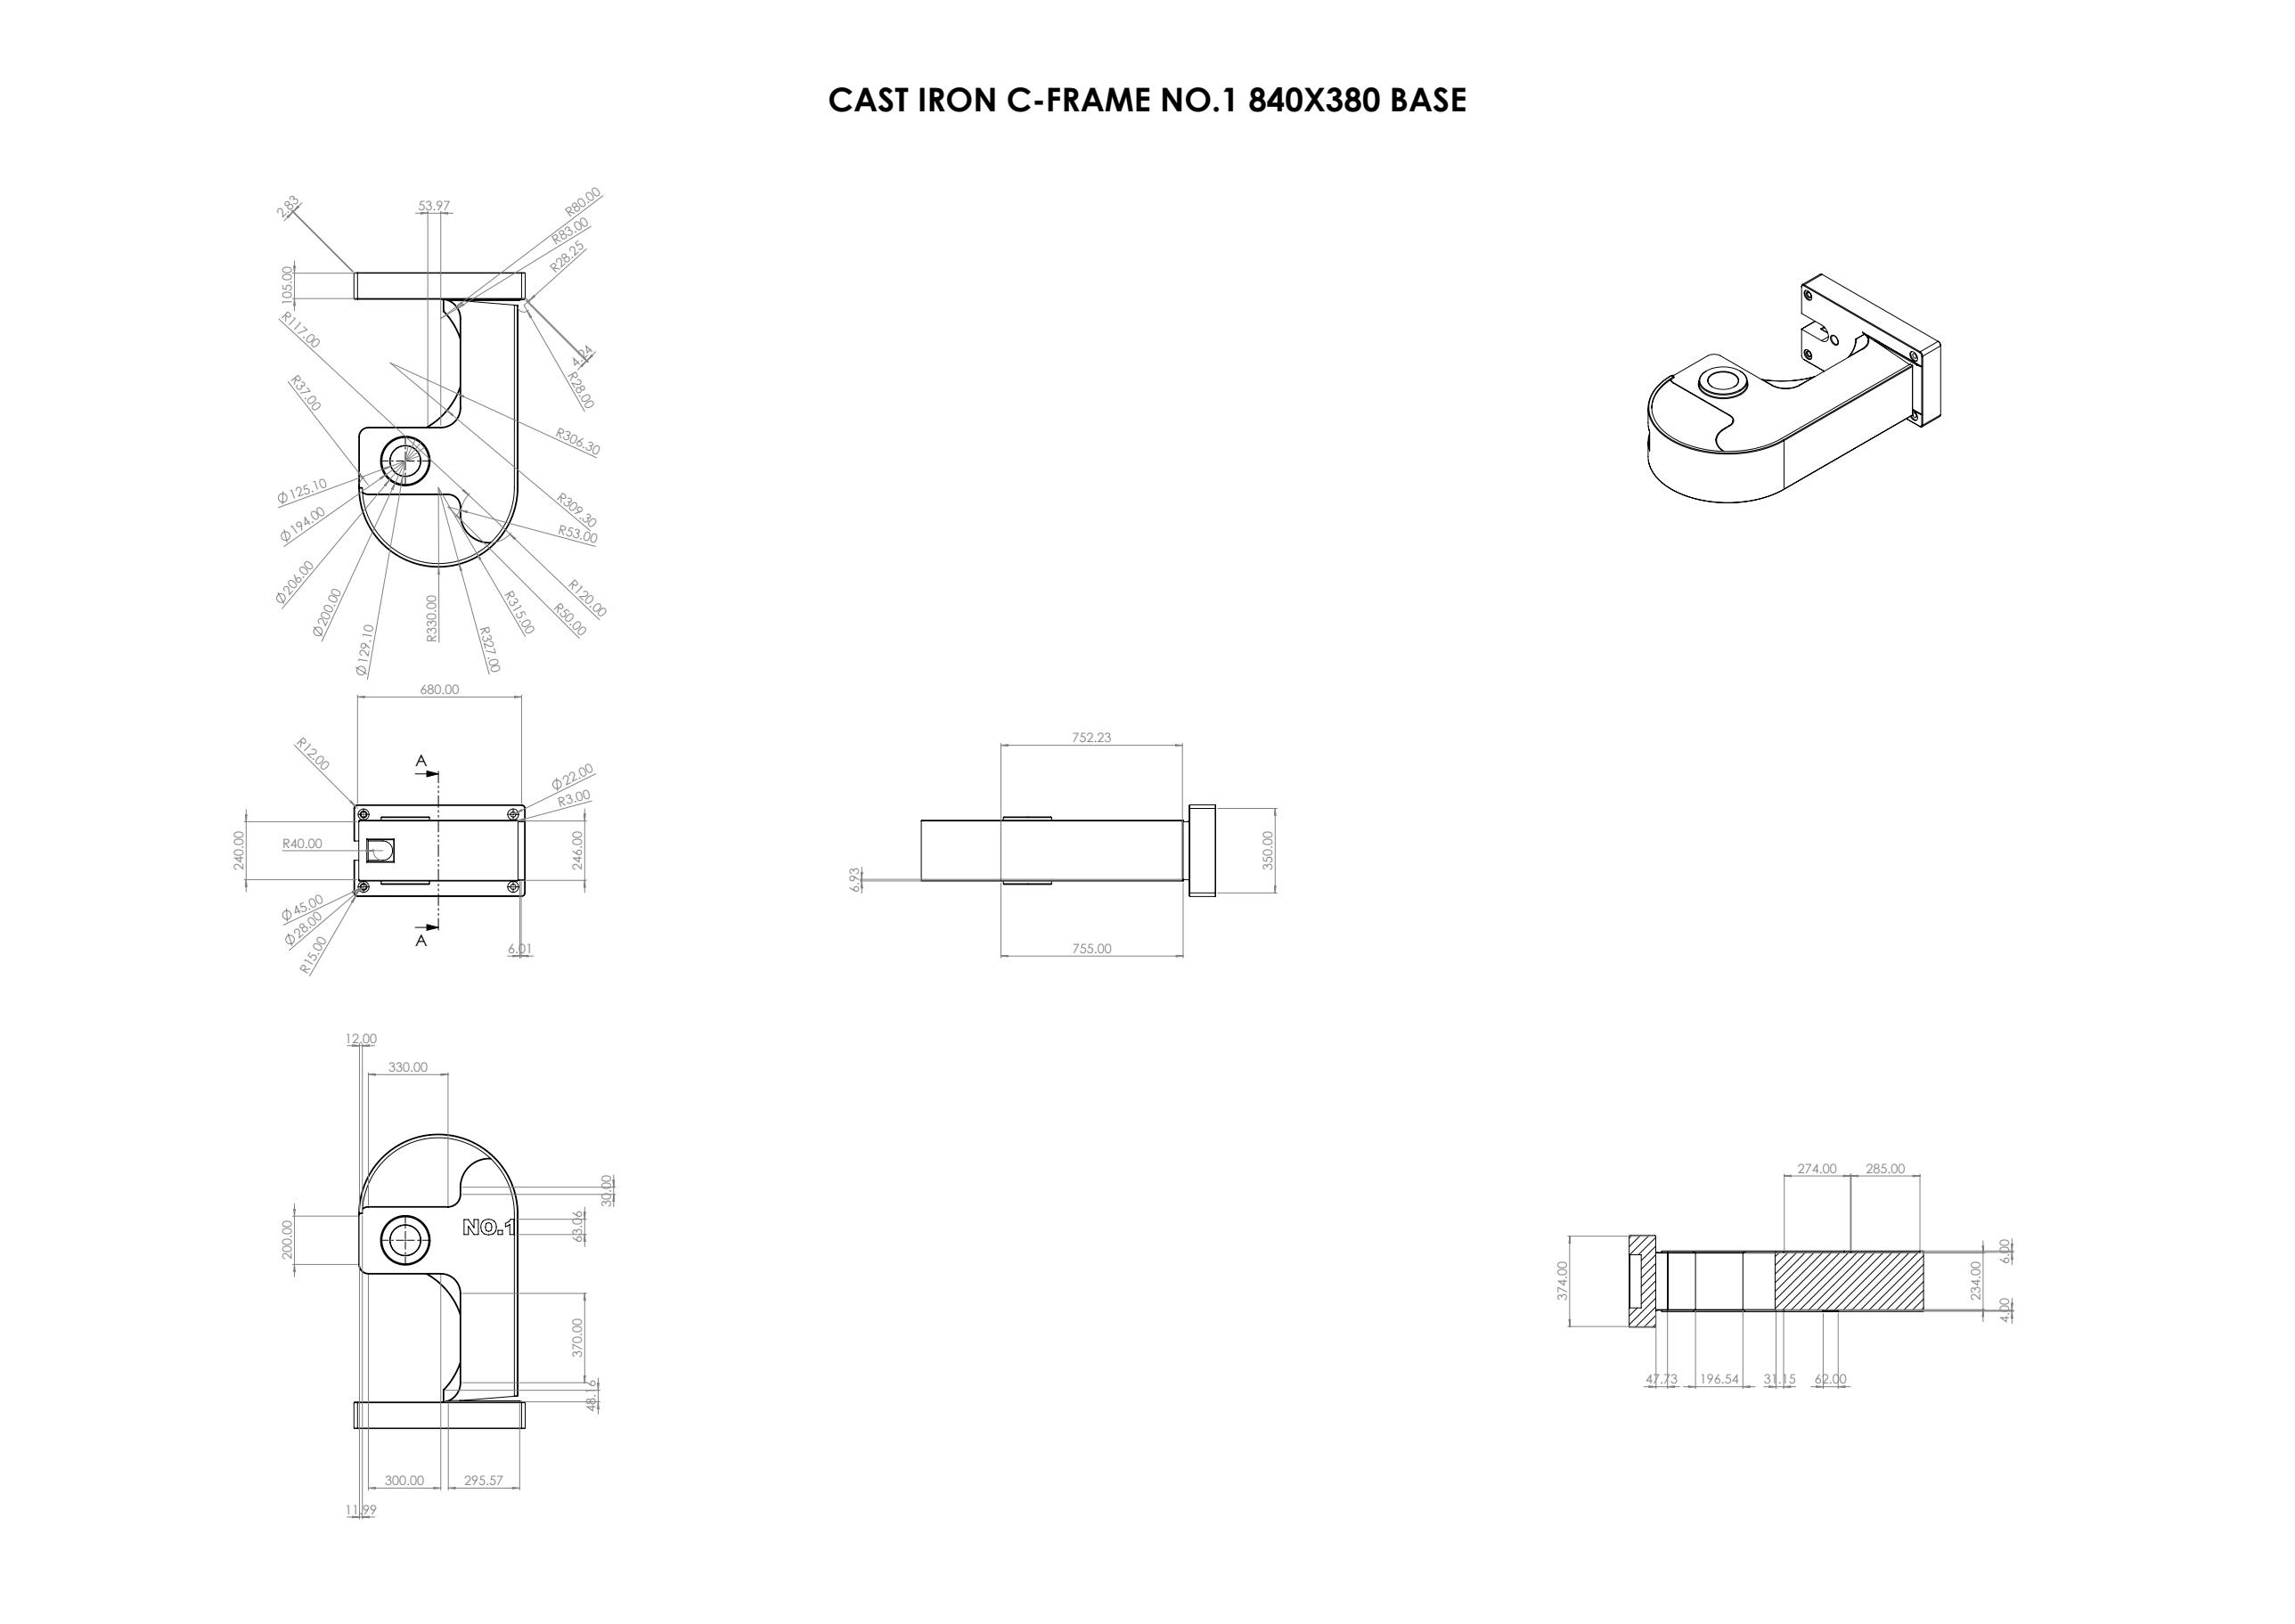
ISO-10303-21;
HEADER;
/* Generated by software containing ST-Developer
 * from STEP Tools, Inc. (www.steptools.com) 
 */

FILE_DESCRIPTION(
/* description */ (''),
/* implementation_level */ '2;1');

FILE_NAME(
/* name */ '01_Cast_Iron_C-Frame_NO.1_840x380_Base.step',
/* time_stamp */ '2026-10-19T23:58:09-07:00',
/* author */ (''),
/* organization */ (''),
/* preprocessor_version */ 'ST-DEVELOPER v20.2',
/* originating_system */ 'Autodesk Translation Framework v15.15.0.0',
/* authorisation */ '');

FILE_SCHEMA (('AP203_CONFIGURATION_CONTROLLED_3D_DESIGN_OF_MECHANICAL_PARTS_AND_ASSEMBLIES_MIM_LF { 1 0 10303 203 3 1 4 }',
'AUTOMOTIVE_DESIGN { 1 0 10303 214 3 1 1 }','INTEGRATED_CNC_SCHEMA','MODEL_BASED_INTEGRATED_MANUFACTURING_SCHEMA',
'PROCESS_PLANNING_SCHEMA','AP242_MANAGED_MODEL_BASED_3D_ENGINEERING_MIM_LF { 1 0 10303 442 3 1 4 }'));
ENDSEC;

DATA;
#10=MECHANICAL_DESIGN_GEOMETRIC_PRESENTATION_REPRESENTATION('',(#420,#421,#422,#423,#424,#425,#426,#427,#428,#429,#430,#431,#432,#433,#434,#435,#436,#437,#438,#439,#440,#441,#442,#443,#444,#445,#446,#447,#448,#449,#450,#451,#452,#453,#454,#455,#456,#457,#458,#459,#460,#461,#462,#463,#464,#465),#70757);
#103=ELLIPSE('',#28418,0.424264068711927,0.3);
#104=ELLIPSE('',#28419,0.42426406871193,0.3);
#105=ELLIPSE('',#28420,0.424264068711931,0.3);
#106=ELLIPSE('',#28425,0.42426406871193,0.3);
#107=ELLIPSE('',#28426,0.424264068711927,0.3);
#108=ELLIPSE('',#28427,0.424264068711928,0.3);
#109=ELLIPSE('',#28431,0.42426406871193,0.3);
#110=ELLIPSE('',#28438,0.424264068711929,0.3);
#111=ELLIPSE('',#28443,0.424264068711926,0.3);
#112=ELLIPSE('',#28444,0.424264068711926,0.3);
#113=ELLIPSE('',#28447,0.424264068711929,0.3);
#114=ELLIPSE('',#28449,0.424264068711931,0.3);
#115=ELLIPSE('',#28458,0.424264068711927,0.3);
#116=ELLIPSE('',#28461,0.42426406871193,0.3);
#117=ELLIPSE('',#28597,5.65698522452918,4.00009261333671);
#118=ELLIPSE('',#28598,5.65698522452918,4.00009261333671);
#119=ELLIPSE('',#28641,0.424264068711926,0.3);
#120=ELLIPSE('',#28642,0.424264068711926,0.3);
#121=ELLIPSE('',#28652,0.424264068711926,0.3);
#122=ELLIPSE('',#28653,0.424264068711926,0.3);
#123=ELLIPSE('',#28709,5.65698522452937,4.00009261333671);
#124=ELLIPSE('',#28711,5.65698522452937,4.00009261333671);
#125=ELLIPSE('',#28723,11.3137084989848,8.);
#126=ELLIPSE('',#28726,11.3137084989848,8.);
#127=ELLIPSE('',#28730,2.63010371137609,2.21164478264163);
#128=ELLIPSE('',#28733,2.63010371137609,2.21164478264163);
#129=ELLIPSE('',#28734,6.83962146739207,5.75141317362232);
#130=ELLIPSE('',#28736,3.53553390593276,2.5);
#131=ELLIPSE('',#28768,11.3130048280025,7.99950242947666);
#132=ELLIPSE('',#28770,11.3130048280025,7.99950242947666);
#133=ELLIPSE('',#28840,6.83962146739207,5.75141317362232);
#134=ELLIPSE('',#28854,3.53553390593276,2.5);
#136=SPHERICAL_SURFACE('',#28433,0.3);
#137=SPHERICAL_SURFACE('',#28439,0.300000000000001);
#138=SPHERICAL_SURFACE('',#28506,0.300000000000004);
#139=SPHERICAL_SURFACE('',#28510,0.299999999999997);
#140=SPHERICAL_SURFACE('',#28532,0.3);
#141=SPHERICAL_SURFACE('',#28555,0.3);
#143=TOROIDAL_SURFACE('',#28397,6.555,0.3);
#144=TOROIDAL_SURFACE('',#28407,6.555,0.3);
#145=TOROIDAL_SURFACE('',#28452,4.3,0.3);
#146=TOROIDAL_SURFACE('',#28476,1.4,0.3);
#147=TOROIDAL_SURFACE('',#28484,1.4,0.3);
#148=TOROIDAL_SURFACE('',#28486,1.4,0.3);
#149=TOROIDAL_SURFACE('',#28494,1.4,0.3);
#150=TOROIDAL_SURFACE('',#28496,1.4,0.3);
#151=TOROIDAL_SURFACE('',#28501,1.4,0.3);
#152=TOROIDAL_SURFACE('',#28516,30.9296013460341,0.3);
#153=TOROIDAL_SURFACE('',#28519,30.9296013460341,0.3);
#154=TOROIDAL_SURFACE('',#28541,32.7,0.3);
#155=TOROIDAL_SURFACE('',#28557,32.7,0.3);
#156=TOROIDAL_SURFACE('',#28568,1.10499999999999,0.3);
#157=TOROIDAL_SURFACE('',#28580,1.10499999999999,0.3);
#158=TOROIDAL_SURFACE('',#28586,1.10499999999999,0.3);
#159=TOROIDAL_SURFACE('',#28592,1.10499999999999,0.3);
#160=TOROIDAL_SURFACE('',#28609,2.3,0.3);
#161=TOROIDAL_SURFACE('',#28615,30.9296013460341,0.3);
#162=TOROIDAL_SURFACE('',#28621,30.9296013460341,0.3);
#163=TOROIDAL_SURFACE('',#28626,2.3,0.3);
#164=TOROIDAL_SURFACE('',#28643,1.10499999999999,0.3);
#165=TOROIDAL_SURFACE('',#28645,1.10499999999999,0.3);
#166=TOROIDAL_SURFACE('',#28647,1.10499999999999,0.3);
#167=TOROIDAL_SURFACE('',#28649,1.10499999999999,0.3);
#168=TOROIDAL_SURFACE('',#28661,32.7,0.3);
#169=TOROIDAL_SURFACE('',#28665,32.7,0.3);
#253=(
BOUNDED_CURVE()
B_SPLINE_CURVE(2,(#64951,#64952,#64953),.UNSPECIFIED.,.F.,.F.)
B_SPLINE_CURVE_WITH_KNOTS((3,3),(0.394392820917162,0.426830556686088),
 .UNSPECIFIED.)
CURVE()
GEOMETRIC_REPRESENTATION_ITEM()
RATIONAL_B_SPLINE_CURVE((1.00046081345666,1.00036632900905,1.00025318515883))
REPRESENTATION_ITEM('')
);
#254=(
BOUNDED_CURVE()
B_SPLINE_CURVE(2,(#64957,#64958,#64959),.UNSPECIFIED.,.F.,.F.)
B_SPLINE_CURVE_WITH_KNOTS((3,3),(0.0334492257654482,0.0658869615343763),
 .UNSPECIFIED.)
CURVE()
GEOMETRIC_REPRESENTATION_ITEM()
RATIONAL_B_SPLINE_CURVE((1.00025318515883,1.00036632900905,1.00046081345666))
REPRESENTATION_ITEM('')
);
#255=(
BOUNDED_CURVE()
B_SPLINE_CURVE(2,(#64996,#64997,#64998),.UNSPECIFIED.,.F.,.F.)
B_SPLINE_CURVE_WITH_KNOTS((3,3),(0.,0.193661196741385),.UNSPECIFIED.)
CURVE()
GEOMETRIC_REPRESENTATION_ITEM()
RATIONAL_B_SPLINE_CURVE((1.,1.00036563245858,1.00040353743124))
REPRESENTATION_ITEM('')
);
#256=(
BOUNDED_CURVE()
B_SPLINE_CURVE(2,(#65154,#65155,#65156),.UNSPECIFIED.,.F.,.F.)
B_SPLINE_CURVE_WITH_KNOTS((3,3),(0.238458916052879,0.432120112749345),
 .UNSPECIFIED.)
CURVE()
GEOMETRIC_REPRESENTATION_ITEM()
RATIONAL_B_SPLINE_CURVE((1.00040353742038,1.0003656324504,1.))
REPRESENTATION_ITEM('')
);
#257=(
BOUNDED_CURVE()
B_SPLINE_CURVE(2,(#65254,#65255,#65256),.UNSPECIFIED.,.F.,.F.)
B_SPLINE_CURVE_WITH_KNOTS((3,3),(0.486252464127642,0.752075607120858),
 .UNSPECIFIED.)
CURVE()
GEOMETRIC_REPRESENTATION_ITEM()
RATIONAL_B_SPLINE_CURVE((1.,1.,1.))
REPRESENTATION_ITEM('')
);
#258=(
BOUNDED_CURVE()
B_SPLINE_CURVE(2,(#65267,#65268,#65269),.UNSPECIFIED.,.F.,.F.)
B_SPLINE_CURVE_WITH_KNOTS((3,3),(0.121648463702186,0.387471606699022),
 .UNSPECIFIED.)
CURVE()
GEOMETRIC_REPRESENTATION_ITEM()
RATIONAL_B_SPLINE_CURVE((1.,1.,1.))
REPRESENTATION_ITEM('')
);
#259=(
BOUNDED_CURVE()
B_SPLINE_CURVE(2,(#65453,#65454,#65455),.UNSPECIFIED.,.F.,.F.)
B_SPLINE_CURVE_WITH_KNOTS((3,3),(0.000218747198876324,0.428298822677418),
 .UNSPECIFIED.)
CURVE()
GEOMETRIC_REPRESENTATION_ITEM()
RATIONAL_B_SPLINE_CURVE((1.,1.,1.))
REPRESENTATION_ITEM('')
);
#260=(
BOUNDED_CURVE()
B_SPLINE_CURVE(2,(#65456,#65457,#65458),.UNSPECIFIED.,.F.,.F.)
B_SPLINE_CURVE_WITH_KNOTS((3,3),(0.432240466163625,0.733007100595233),
 .UNSPECIFIED.)
CURVE()
GEOMETRIC_REPRESENTATION_ITEM()
RATIONAL_B_SPLINE_CURVE((1.,1.,1.))
REPRESENTATION_ITEM('')
);
#261=(
BOUNDED_CURVE()
B_SPLINE_CURVE(2,(#65913,#65914,#65915),.UNSPECIFIED.,.F.,.F.)
B_SPLINE_CURVE_WITH_KNOTS((3,3),(0.,0.428080075478541),.UNSPECIFIED.)
CURVE()
GEOMETRIC_REPRESENTATION_ITEM()
RATIONAL_B_SPLINE_CURVE((1.,1.,1.))
REPRESENTATION_ITEM('')
);
#262=(
BOUNDED_CURVE()
B_SPLINE_CURVE(2,(#65916,#65917,#65918),.UNSPECIFIED.,.F.,.F.)
B_SPLINE_CURVE_WITH_KNOTS((3,3),(0.12344249829562,0.424209132727228),
 .UNSPECIFIED.)
CURVE()
GEOMETRIC_REPRESENTATION_ITEM()
RATIONAL_B_SPLINE_CURVE((1.,1.,1.))
REPRESENTATION_ITEM('')
);
#287=B_SPLINE_SURFACE_WITH_KNOTS('',2,1,((#65478,#65479),(#65480,#65481),
(#65482,#65483)),.UNSPECIFIED.,.F.,.F.,.F.,(3,3),(2,2),(-1.,0.),(0.,0.4),
 .UNSPECIFIED.);
#288=B_SPLINE_SURFACE_WITH_KNOTS('',2,1,((#65489,#65490),(#65491,#65492),
(#65493,#65494)),.UNSPECIFIED.,.F.,.F.,.F.,(3,3),(2,2),(-1.,0.),(0.,0.4),
 .UNSPECIFIED.);
#289=B_SPLINE_SURFACE_WITH_KNOTS('',2,1,((#65504,#65505),(#65506,#65507),
(#65508,#65509)),.UNSPECIFIED.,.F.,.F.,.F.,(3,3),(2,2),(-1.,0.),(0.,0.4),
 .UNSPECIFIED.);
#290=B_SPLINE_SURFACE_WITH_KNOTS('',2,1,((#65515,#65516),(#65517,#65518),
(#65519,#65520)),.UNSPECIFIED.,.F.,.F.,.F.,(3,3),(2,2),(-1.,0.),(0.,0.4),
 .UNSPECIFIED.);
#291=B_SPLINE_SURFACE_WITH_KNOTS('',2,1,((#65570,#65571),(#65572,#65573),
(#65574,#65575)),.UNSPECIFIED.,.F.,.F.,.F.,(3,3),(2,2),(-1.,0.),(0.,0.4),
 .UNSPECIFIED.);
#292=B_SPLINE_SURFACE_WITH_KNOTS('',2,1,((#65588,#65589),(#65590,#65591),
(#65592,#65593)),.UNSPECIFIED.,.F.,.F.,.F.,(3,3),(2,2),(-1.,0.),(0.,0.4),
 .UNSPECIFIED.);
#293=B_SPLINE_SURFACE_WITH_KNOTS('',2,1,((#65603,#65604),(#65605,#65606),
(#65607,#65608)),.UNSPECIFIED.,.F.,.F.,.F.,(3,3),(2,2),(-1.,0.),(0.,0.4),
 .UNSPECIFIED.);
#294=B_SPLINE_SURFACE_WITH_KNOTS('',2,1,((#65618,#65619),(#65620,#65621),
(#65622,#65623)),.UNSPECIFIED.,.F.,.F.,.F.,(3,3),(2,2),(-1.,0.),(0.,0.4),
 .UNSPECIFIED.);
#295=B_SPLINE_SURFACE_WITH_KNOTS('',2,1,((#65633,#65634),(#65635,#65636),
(#65637,#65638)),.UNSPECIFIED.,.F.,.F.,.F.,(3,3),(2,2),(-1.,0.),(0.,0.4),
 .UNSPECIFIED.);
#296=B_SPLINE_SURFACE_WITH_KNOTS('',2,1,((#65648,#65649),(#65650,#65651),
(#65652,#65653)),.UNSPECIFIED.,.F.,.F.,.F.,(3,3),(2,2),(-1.,0.),(0.,0.4),
 .UNSPECIFIED.);
#297=B_SPLINE_SURFACE_WITH_KNOTS('',2,1,((#65663,#65664),(#65665,#65666),
(#65667,#65668)),.UNSPECIFIED.,.F.,.F.,.F.,(3,3),(2,2),(-1.,0.),(0.,0.4),
 .UNSPECIFIED.);
#298=B_SPLINE_SURFACE_WITH_KNOTS('',2,1,((#65678,#65679),(#65680,#65681),
(#65682,#65683)),.UNSPECIFIED.,.F.,.F.,.F.,(3,3),(2,2),(-1.,0.),(0.,0.4),
 .UNSPECIFIED.);
#299=B_SPLINE_SURFACE_WITH_KNOTS('',2,1,((#65690,#65691),(#65692,#65693),
(#65694,#65695)),.UNSPECIFIED.,.F.,.F.,.F.,(3,3),(2,2),(-1.,0.),(0.,0.4),
 .UNSPECIFIED.);
#300=B_SPLINE_SURFACE_WITH_KNOTS('',2,1,((#65703,#65704),(#65705,#65706),
(#65707,#65708)),.UNSPECIFIED.,.F.,.F.,.F.,(3,3),(2,2),(-1.,0.),(0.,0.4),
 .UNSPECIFIED.);
#301=B_SPLINE_SURFACE_WITH_KNOTS('',2,1,((#65714,#65715),(#65716,#65717),
(#65718,#65719)),.UNSPECIFIED.,.F.,.F.,.F.,(3,3),(2,2),(-1.,0.),(0.,0.4),
 .UNSPECIFIED.);
#302=B_SPLINE_SURFACE_WITH_KNOTS('',2,1,((#65725,#65726),(#65727,#65728),
(#65729,#65730)),.UNSPECIFIED.,.F.,.F.,.F.,(3,3),(2,2),(-1.,0.),(0.,0.4),
 .UNSPECIFIED.);
#303=B_SPLINE_SURFACE_WITH_KNOTS('',2,1,((#65736,#65737),(#65738,#65739),
(#65740,#65741)),.UNSPECIFIED.,.F.,.F.,.F.,(3,3),(2,2),(-1.,0.),(0.,0.4),
 .UNSPECIFIED.);
#304=B_SPLINE_SURFACE_WITH_KNOTS('',2,1,((#65747,#65748),(#65749,#65750),
(#65751,#65752)),.UNSPECIFIED.,.F.,.F.,.F.,(3,3),(2,2),(-1.,0.),(0.,0.4),
 .UNSPECIFIED.);
#305=B_SPLINE_SURFACE_WITH_KNOTS('',2,1,((#65758,#65759),(#65760,#65761),
(#65762,#65763)),.UNSPECIFIED.,.F.,.F.,.F.,(3,3),(2,2),(-1.,0.),(0.,0.4),
 .UNSPECIFIED.);
#306=B_SPLINE_SURFACE_WITH_KNOTS('',2,1,((#65769,#65770),(#65771,#65772),
(#65773,#65774)),.UNSPECIFIED.,.F.,.F.,.F.,(3,3),(2,2),(-1.,0.),(0.,0.4),
 .UNSPECIFIED.);
#307=B_SPLINE_SURFACE_WITH_KNOTS('',2,1,((#65780,#65781),(#65782,#65783),
(#65784,#65785)),.UNSPECIFIED.,.F.,.F.,.F.,(3,3),(2,2),(-1.,0.),(0.,0.4),
 .UNSPECIFIED.);
#308=B_SPLINE_SURFACE_WITH_KNOTS('',2,1,((#65791,#65792),(#65793,#65794),
(#65795,#65796)),.UNSPECIFIED.,.F.,.F.,.F.,(3,3),(2,2),(-1.,0.),(0.,0.4),
 .UNSPECIFIED.);
#390=SHAPE_REPRESENTATION_RELATIONSHIP('SRR','None',#70831,#405);
#405=ADVANCED_BREP_SHAPE_REPRESENTATION('',(#480),#70755);
#420=STYLED_ITEM('',(#71026),#26633);
#421=STYLED_ITEM('',(#71026),#26634);
#422=STYLED_ITEM('',(#71026),#26635);
#423=STYLED_ITEM('',(#71026),#26636);
#424=STYLED_ITEM('',(#71026),#26637);
#425=STYLED_ITEM('',(#71026),#26638);
#426=STYLED_ITEM('',(#71026),#26639);
#427=STYLED_ITEM('',(#71026),#26640);
#428=STYLED_ITEM('',(#71026),#26641);
#429=STYLED_ITEM('',(#71026),#26642);
#430=STYLED_ITEM('',(#71026),#26643);
#431=STYLED_ITEM('',(#71026),#26644);
#432=STYLED_ITEM('',(#71026),#26645);
#433=STYLED_ITEM('',(#71026),#26646);
#434=STYLED_ITEM('',(#71026),#26647);
#435=STYLED_ITEM('',(#71026),#26648);
#436=STYLED_ITEM('',(#71026),#26649);
#437=STYLED_ITEM('',(#71026),#26650);
#438=STYLED_ITEM('',(#71026),#26651);
#439=STYLED_ITEM('',(#71026),#26652);
#440=STYLED_ITEM('',(#71026),#26653);
#441=STYLED_ITEM('',(#71026),#26654);
#442=STYLED_ITEM('',(#71026),#26655);
#443=STYLED_ITEM('',(#71026),#26656);
#444=STYLED_ITEM('',(#71026),#26657);
#445=STYLED_ITEM('',(#71026),#26658);
#446=STYLED_ITEM('',(#71026),#26659);
#447=STYLED_ITEM('',(#71026),#26660);
#448=STYLED_ITEM('',(#71026),#26661);
#449=STYLED_ITEM('',(#71026),#26662);
#450=STYLED_ITEM('',(#71026),#26663);
#451=STYLED_ITEM('',(#71026),#26664);
#452=STYLED_ITEM('',(#71026),#26665);
#453=STYLED_ITEM('',(#71026),#26666);
#454=STYLED_ITEM('',(#71026),#26667);
#455=STYLED_ITEM('',(#71026),#26668);
#456=STYLED_ITEM('',(#71026),#26669);
#457=STYLED_ITEM('',(#71026),#26670);
#458=STYLED_ITEM('',(#71026),#26671);
#459=STYLED_ITEM('',(#71026),#26672);
#460=STYLED_ITEM('',(#71026),#26673);
#461=STYLED_ITEM('',(#71026),#26674);
#462=STYLED_ITEM('',(#71026),#26675);
#463=STYLED_ITEM('',(#71026),#26676);
#464=STYLED_ITEM('',(#71026),#26677);
#465=STYLED_ITEM('',(#71026),#480);
#480=MANIFOLD_SOLID_BREP('Frame',#26885);
#741=CYLINDRICAL_SURFACE('',#28401,0.3);
#742=CYLINDRICAL_SURFACE('',#28404,0.3);
#743=CYLINDRICAL_SURFACE('',#28414,6.255);
#744=CYLINDRICAL_SURFACE('',#28417,0.3);
#745=CYLINDRICAL_SURFACE('',#28424,0.3);
#746=CYLINDRICAL_SURFACE('',#28430,0.3);
#747=CYLINDRICAL_SURFACE('',#28437,0.3);
#748=CYLINDRICAL_SURFACE('',#28442,0.3);
#749=CYLINDRICAL_SURFACE('',#28445,0.3);
#750=CYLINDRICAL_SURFACE('',#28446,0.3);
#751=CYLINDRICAL_SURFACE('',#28448,0.3);
#752=CYLINDRICAL_SURFACE('',#28450,0.3);
#753=CYLINDRICAL_SURFACE('',#28456,0.3);
#754=CYLINDRICAL_SURFACE('',#28457,0.3);
#755=CYLINDRICAL_SURFACE('',#28459,0.3);
#756=CYLINDRICAL_SURFACE('',#28460,0.3);
#757=CYLINDRICAL_SURFACE('',#28480,1.1);
#758=CYLINDRICAL_SURFACE('',#28490,1.1);
#759=CYLINDRICAL_SURFACE('',#28499,1.1);
#760=CYLINDRICAL_SURFACE('',#28504,1.1);
#761=CYLINDRICAL_SURFACE('',#28514,0.3);
#762=CYLINDRICAL_SURFACE('',#28515,0.3);
#763=CYLINDRICAL_SURFACE('',#28522,0.3);
#764=CYLINDRICAL_SURFACE('',#28527,0.3);
#765=CYLINDRICAL_SURFACE('',#28529,0.3);
#766=CYLINDRICAL_SURFACE('',#28534,31.5);
#767=CYLINDRICAL_SURFACE('',#28544,33.);
#768=CYLINDRICAL_SURFACE('',#28550,0.3);
#769=CYLINDRICAL_SURFACE('',#28553,0.3);
#770=CYLINDRICAL_SURFACE('',#28562,31.5);
#771=CYLINDRICAL_SURFACE('',#28566,0.3);
#772=CYLINDRICAL_SURFACE('',#28578,0.804999999999993);
#773=CYLINDRICAL_SURFACE('',#28584,0.804999999999993);
#774=CYLINDRICAL_SURFACE('',#28590,0.804999999999993);
#775=CYLINDRICAL_SURFACE('',#28596,4.00009261333671);
#776=CYLINDRICAL_SURFACE('',#28599,0.804999999999993);
#777=CYLINDRICAL_SURFACE('',#28601,0.3);
#778=CYLINDRICAL_SURFACE('',#28612,2.);
#779=CYLINDRICAL_SURFACE('',#28618,30.6296013460341);
#780=CYLINDRICAL_SURFACE('',#28639,0.3);
#781=CYLINDRICAL_SURFACE('',#28651,0.3);
#782=CYLINDRICAL_SURFACE('',#28654,0.3);
#783=CYLINDRICAL_SURFACE('',#28669,0.3);
#784=CYLINDRICAL_SURFACE('',#28686,4.00009261333671);
#785=CYLINDRICAL_SURFACE('',#28691,12.);
#786=CYLINDRICAL_SURFACE('',#28705,4.00009261333671);
#787=CYLINDRICAL_SURFACE('',#28708,4.00009261333671);
#788=CYLINDRICAL_SURFACE('',#28710,4.00009261333671);
#789=CYLINDRICAL_SURFACE('',#28722,8.);
#790=CYLINDRICAL_SURFACE('',#28724,8.);
#791=CYLINDRICAL_SURFACE('',#28735,2.5);
#792=CYLINDRICAL_SURFACE('',#28740,7.99950242947665);
#793=CYLINDRICAL_SURFACE('',#28741,7.99950242947665);
#794=CYLINDRICAL_SURFACE('',#28746,12.);
#795=CYLINDRICAL_SURFACE('',#28754,4.00009261333671);
#796=CYLINDRICAL_SURFACE('',#28758,4.00009261333671);
#797=CYLINDRICAL_SURFACE('',#28760,5.00011576667089);
#798=CYLINDRICAL_SURFACE('',#28767,7.99950242947666);
#799=CYLINDRICAL_SURFACE('',#28769,7.99950242947666);
#800=CYLINDRICAL_SURFACE('',#28772,30.6296013460341);
#801=CYLINDRICAL_SURFACE('',#28802,2.25);
#802=CYLINDRICAL_SURFACE('',#28805,2.25);
#803=CYLINDRICAL_SURFACE('',#28806,2.25);
#804=CYLINDRICAL_SURFACE('',#28807,2.25);
#805=CYLINDRICAL_SURFACE('',#28811,4.);
#806=CYLINDRICAL_SURFACE('',#28830,10.);
#807=CYLINDRICAL_SURFACE('',#28836,10.);
#808=CYLINDRICAL_SURFACE('',#28851,5.);
#809=CYLINDRICAL_SURFACE('',#28853,2.5);
#810=CYLINDRICAL_SURFACE('',#28873,1.5);
#811=CYLINDRICAL_SURFACE('',#28876,1.5);
#812=CYLINDRICAL_SURFACE('',#28889,1.5);
#813=CYLINDRICAL_SURFACE('',#28890,1.5);
#887=FACE_BOUND('',#5214,.T.);
#888=FACE_BOUND('',#5215,.T.);
#889=FACE_BOUND('',#5216,.T.);
#890=FACE_BOUND('',#5217,.T.);
#891=FACE_BOUND('',#5219,.T.);
#892=FACE_BOUND('',#5225,.T.);
#893=FACE_BOUND('',#5230,.T.);
#894=FACE_BOUND('',#5252,.T.);
#895=FACE_BOUND('',#5263,.T.);
#896=FACE_BOUND('',#5264,.T.);
#897=FACE_BOUND('',#5265,.T.);
#898=FACE_BOUND('',#5276,.T.);
#899=FACE_BOUND('',#5277,.T.);
#900=FACE_BOUND('',#5278,.T.);
#901=FACE_BOUND('',#5279,.T.);
#902=FACE_BOUND('',#5290,.T.);
#903=FACE_BOUND('',#5291,.T.);
#904=FACE_BOUND('',#5292,.T.);
#905=FACE_BOUND('',#5293,.T.);
#906=FACE_BOUND('',#5294,.T.);
#907=FACE_BOUND('',#5295,.T.);
#908=FACE_BOUND('',#5318,.T.);
#909=FACE_BOUND('',#5319,.T.);
#910=FACE_BOUND('',#5320,.T.);
#911=FACE_BOUND('',#5321,.T.);
#912=FACE_BOUND('',#5322,.T.);
#913=FACE_BOUND('',#5330,.T.);
#914=FACE_BOUND('',#5418,.T.);
#915=FACE_BOUND('',#5425,.T.);
#916=FACE_BOUND('',#5428,.T.);
#917=FACE_BOUND('',#5446,.T.);
#918=FACE_BOUND('',#5449,.T.);
#1398=B_SPLINE_CURVE_WITH_KNOTS('',3,(#63938,#63939,#63940,#63941,#63942,
#63943,#63944,#63945,#63946,#63947,#63948,#63949),.UNSPECIFIED.,.F.,.F.,
(4,2,2,2,2,4),(-1.10588413989679,-1.10499782596143,-0.91656040147052,-0.772228700060969,
-0.6650055247649,-0.579920166124102),.UNSPECIFIED.);
#1399=B_SPLINE_CURVE_WITH_KNOTS('',3,(#63952,#63953,#63954,#63955,#63956,
#63957,#63958,#63959,#63960,#63961,#63962,#63963,#63964,#63965),
 .UNSPECIFIED.,.F.,.F.,(4,2,2,2,2,2,4),(-0.568877288175113,-0.484148554868537,
-0.388033769227592,-0.2597032346067,-0.133006563450214,0.,0.00108165162707012),
 .UNSPECIFIED.);
#1400=B_SPLINE_CURVE_WITH_KNOTS('',3,(#63974,#63975,#63976,#63977,#63978,
#63979,#63980,#63981,#63982,#63983,#63984,#63985),.UNSPECIFIED.,.F.,.F.,
(4,2,2,2,2,4),(-0.00108165162924514,0.,0.229967778999105,0.40610922702663,
0.536963676703178,0.64080128223702),.UNSPECIFIED.);
#1401=B_SPLINE_CURVE_WITH_KNOTS('',3,(#63996,#63997,#63998,#63999,#64000,
#64001,#64002,#64003,#64004,#64005,#64006,#64007,#64008,#64009),
 .UNSPECIFIED.,.F.,.F.,(4,2,2,2,2,2,4),(0.,0.0839640955338038,0.179211489526657,
0.306383900210746,0.431937192294976,0.563743432804494,0.564815323027158),
 .UNSPECIFIED.);
#1402=B_SPLINE_CURVE_WITH_KNOTS('',3,(#64272,#64273,#64274,#64275,#64276,
#64277,#64278,#64279,#64280,#64281),.UNSPECIFIED.,.F.,.F.,(4,2,2,2,4),(-0.454509794253164,
-0.340166127818439,-0.225822461383713,-0.112911230691856,0.),
 .UNSPECIFIED.);
#1403=B_SPLINE_CURVE_WITH_KNOTS('',3,(#64287,#64288,#64289,#64290,#64291,
#64292,#64293,#64294,#64295,#64296,#64297,#64298,#64299,#64300),
 .UNSPECIFIED.,.F.,.F.,(4,2,2,2,2,2,4),(0.896032537461048,1.25582804826943,
1.43572580367362,1.61562355907781,1.76667897073219,1.80865046008187,1.84248908085934),
 .UNSPECIFIED.);
#1404=B_SPLINE_CURVE_WITH_KNOTS('',3,(#64306,#64307,#64308,#64309,#64310,
#64311,#64312,#64313,#64314,#64315,#64316,#64317,#64318,#64319),
 .UNSPECIFIED.,.F.,.F.,(4,2,2,2,2,2,4),(-1.84248908085934,-1.80865046008187,
-1.76667897073219,-1.61562355907781,-1.43572580367362,-1.25582804826943,
-0.896032537461048),.UNSPECIFIED.);
#1405=B_SPLINE_CURVE_WITH_KNOTS('',3,(#64325,#64326,#64327,#64328,#64329,
#64330,#64331,#64332,#64333,#64334),.UNSPECIFIED.,.F.,.F.,(4,2,2,2,4),(0.910251315816355,
1.02316254650821,1.13607377720007,1.25041744363479,1.36476111006952),
 .UNSPECIFIED.);
#1406=B_SPLINE_CURVE_WITH_KNOTS('',3,(#64358,#64359,#64360,#64361,#64362,
#64363,#64364,#64365,#64366,#64367),.UNSPECIFIED.,.F.,.F.,(4,2,2,2,4),(0.45204596998448,
0.565054126336166,0.678062282687852,0.791068360433516,0.904074438179181),
 .UNSPECIFIED.);
#1407=B_SPLINE_CURVE_WITH_KNOTS('',3,(#64376,#64377,#64378,#64379,#64380,
#64381),.UNSPECIFIED.,.F.,.F.,(4,2,4),(1.02915974263557,1.15320944997464,
1.25900965381776),.UNSPECIFIED.);
#1408=B_SPLINE_CURVE_WITH_KNOTS('',3,(#64400,#64401,#64402,#64403,#64404,
#64405),.UNSPECIFIED.,.F.,.F.,(4,2,4),(1.70043874542,2.00091514457436,2.20444648124611),
 .UNSPECIFIED.);
#1409=B_SPLINE_CURVE_WITH_KNOTS('',3,(#64413,#64414,#64415,#64416,#64417,
#64418),.UNSPECIFIED.,.F.,.F.,(4,2,4),(1.92266359511738,1.95634912709283,
2.38915999737552),.UNSPECIFIED.);
#1410=B_SPLINE_CURVE_WITH_KNOTS('',3,(#64457,#64458,#64459,#64460,#64461,
#64462),.UNSPECIFIED.,.F.,.F.,(4,2,4),(0.941765464328093,1.04756566817122,
1.17161537551029),.UNSPECIFIED.);
#1411=B_SPLINE_CURVE_WITH_KNOTS('',3,(#64472,#64473,#64474,#64475,#64476,
#64477,#64478,#64479,#64480,#64481),.UNSPECIFIED.,.F.,.F.,(4,2,2,2,4),(1.80814887635836,
1.92115495410403,2.03416103184969,2.14716918820138,2.26017734455306),
 .UNSPECIFIED.);
#1412=B_SPLINE_CURVE_WITH_KNOTS('',3,(#64506,#64507,#64508,#64509,#64510,
#64511),.UNSPECIFIED.,.F.,.F.,(4,2,4),(1.52353825936373,1.95634912840093,
1.99003466162308),.UNSPECIFIED.);
#1413=B_SPLINE_CURVE_WITH_KNOTS('',3,(#64519,#64520,#64521,#64522,#64523,
#64524),.UNSPECIFIED.,.F.,.F.,(4,2,4),(1.79738380790266,2.00091514457441,
2.30139154372878),.UNSPECIFIED.);
#1414=B_SPLINE_CURVE_WITH_KNOTS('',3,(#64530,#64531,#64532,#64533,#64534,
#64535,#64536,#64537,#64538,#64539),.UNSPECIFIED.,.F.,.F.,(4,2,2,2,4),(-0.385669957148059,
-0.267638091880424,-0.132795783635376,0.,0.000970573886634806),
 .UNSPECIFIED.);
#1415=B_SPLINE_CURVE_WITH_KNOTS('',3,(#64542,#64543,#64544,#64545,#64546,
#64547,#64548,#64549,#64550,#64551),.UNSPECIFIED.,.F.,.F.,(4,2,2,2,4),(-0.384357938358326,
-0.383393117455112,-0.251376894581821,-0.117331137795169,-6.31601177111807E-6),
 .UNSPECIFIED.);
#1416=B_SPLINE_CURVE_WITH_KNOTS('',3,(#64554,#64555,#64556,#64557,#64558,
#64559),.UNSPECIFIED.,.F.,.F.,(4,2,4),(0.29237536973302,0.349212088502275,
0.491998450222318),.UNSPECIFIED.);
#1417=B_SPLINE_CURVE_WITH_KNOTS('',3,(#64566,#64567,#64568,#64569,#64570,
#64571),.UNSPECIFIED.,.F.,.F.,(4,2,4),(1.47810928760726,1.6208956493273,
1.67773236809654),.UNSPECIFIED.);
#1418=B_SPLINE_CURVE_WITH_KNOTS('',3,(#64629,#64630,#64631,#64632,#64633,
#64634,#64635,#64636,#64637,#64638),.UNSPECIFIED.,.F.,.F.,(4,2,2,2,4),(-0.00645513076503384,
0.,0.607350167241916,1.21470033231699,1.22115546305417),.UNSPECIFIED.);
#1419=B_SPLINE_CURVE_WITH_KNOTS('',3,(#64646,#64647,#64648,#64649,#64650,
#64651,#64652,#64653,#64654,#64655,#64656,#64657,#64658,#64659,#64660,#64661,
#64662,#64663),.UNSPECIFIED.,.F.,.F.,(4,2,2,2,2,2,2,2,4),(0.,0.753367592696705,
1.50673518539341,2.26010277809012,3.01347037078682,3.76683796348352,4.52020555618022,
5.27357314887692,6.02694074157362),.UNSPECIFIED.);
#1420=B_SPLINE_CURVE_WITH_KNOTS('',3,(#64674,#64675,#64676,#64677,#64678,
#64679,#64680,#64681,#64682,#64683,#64684,#64685,#64686,#64687,#64688,#64689,
#64690,#64691),.UNSPECIFIED.,.F.,.F.,(4,2,2,2,2,2,2,2,4),(-6.02694148316008,
-5.27373586786722,-4.52034502960047,-3.76695419133371,-3.01356335306695,
-2.26017251480021,-1.50678167653347,-0.753390838266739,0.),
 .UNSPECIFIED.);
#1421=B_SPLINE_CURVE_WITH_KNOTS('',3,(#64698,#64699,#64700,#64701,#64702,
#64703,#64704,#64705,#64706,#64707,#64708,#64709,#64710,#64711),
 .UNSPECIFIED.,.F.,.F.,(4,2,2,2,2,2,4),(-1.35055637186862,-1.34938170454602,
-1.1819777528807,-1.01919166368985,-0.865721094274056,-0.748962828335224,
-0.646651719983809),.UNSPECIFIED.);
#1422=B_SPLINE_CURVE_WITH_KNOTS('',3,(#64713,#64714,#64715,#64716,#64717,
#64718,#64719,#64720,#64721,#64722,#64723,#64724,#64725,#64726),
 .UNSPECIFIED.,.F.,.F.,(4,2,2,2,2,2,4),(-0.575633174348645,-0.491826207716573,
-0.3961850186411,-0.270471368845074,-0.13712701884174,0.,0.000962215215251001),
 .UNSPECIFIED.);
#1423=B_SPLINE_CURVE_WITH_KNOTS('',3,(#64768,#64769,#64770,#64771,#64772,
#64773,#64774,#64775,#64776,#64777,#64778,#64779,#64780,#64781),
 .UNSPECIFIED.,.F.,.F.,(4,2,2,2,2,2,4),(-1.35886617414881,-1.31800777766679,
-1.27191156834586,-1.14095894304151,-0.942079387318738,-0.807488859272477,
-0.672898331226217),.UNSPECIFIED.);
#1424=B_SPLINE_CURVE_WITH_KNOTS('',3,(#64785,#64786,#64787,#64788,#64789,
#64790,#64791,#64792,#64793,#64794,#64795,#64796,#64797,#64798),
 .UNSPECIFIED.,.F.,.F.,(4,2,2,2,2,2,4),(0.896032537461047,1.25582804826943,
1.43572580367362,1.61562355907781,1.76667897073219,1.80865046008187,1.84248908085934),
 .UNSPECIFIED.);
#1425=B_SPLINE_CURVE_WITH_KNOTS('',3,(#64814,#64815,#64816,#64817,#64818,
#64819,#64820,#64821,#64822,#64823,#64824,#64825,#64826,#64827),
 .UNSPECIFIED.,.F.,.F.,(4,2,2,2,2,2,4),(-1.84248908085934,-1.80865046008187,
-1.76667897073219,-1.61562355907781,-1.43572580367362,-1.25582804826943,
-0.896032537461046),.UNSPECIFIED.);
#1426=B_SPLINE_CURVE_WITH_KNOTS('',3,(#64830,#64831,#64832,#64833,#64834,
#64835,#64836,#64837,#64838,#64839,#64840,#64841,#64842,#64843),
 .UNSPECIFIED.,.F.,.F.,(4,2,2,2,2,2,4),(0.672898331226217,0.807488859272477,
0.942079387318738,1.14095894304151,1.27191156834586,1.31800777766679,1.35886617414881),
 .UNSPECIFIED.);
#1427=B_SPLINE_CURVE_WITH_KNOTS('',3,(#64924,#64925,#64926,#64927,#64928,
#64929),.UNSPECIFIED.,.F.,.F.,(4,2,4),(-0.154287651470972,-0.153320461931147,
-0.0301403351196061),.UNSPECIFIED.);
#1428=B_SPLINE_CURVE_WITH_KNOTS('',3,(#64933,#64934,#64935,#64936,#64937,
#64938),.UNSPECIFIED.,.F.,.F.,(4,2,4),(0.0301403351196109,0.153320461931147,
0.154287651470978),.UNSPECIFIED.);
#1429=B_SPLINE_CURVE_WITH_KNOTS('',3,(#65002,#65003,#65004,#65005),
 .UNSPECIFIED.,.F.,.F.,(4,4),(23.0837010026238,23.1300949206487),
 .UNSPECIFIED.);
#1430=B_SPLINE_CURVE_WITH_KNOTS('',3,(#65006,#65007,#65008,#65009,#65010,
#65011),.UNSPECIFIED.,.F.,.F.,(4,2,4),(-0.978411907643555,-0.753390838266736,
0.),.UNSPECIFIED.);
#1431=B_SPLINE_CURVE_WITH_KNOTS('',3,(#65020,#65021,#65022,#65023,#65024,
#65025,#65026,#65027,#65028,#65029),.UNSPECIFIED.,.F.,.F.,(4,2,2,2,4),(-6.02694148316005,
-5.27373586786722,-4.52034502960046,-3.7669541913337,-3.53970622743003),
 .UNSPECIFIED.);
#1432=B_SPLINE_CURVE_WITH_KNOTS('',2,(#65054,#65055,#65056),
 .UNSPECIFIED.,.F.,.F.,(3,3),(0.,1.),.UNSPECIFIED.);
#1433=B_SPLINE_CURVE_WITH_KNOTS('',2,(#65058,#65059,#65060),
 .UNSPECIFIED.,.F.,.F.,(3,3),(0.,1.),.UNSPECIFIED.);
#1434=B_SPLINE_CURVE_WITH_KNOTS('',2,(#65062,#65063,#65064),
 .UNSPECIFIED.,.F.,.F.,(3,3),(0.,1.),.UNSPECIFIED.);
#1435=B_SPLINE_CURVE_WITH_KNOTS('',2,(#65066,#65067,#65068),
 .UNSPECIFIED.,.F.,.F.,(3,3),(0.,1.),.UNSPECIFIED.);
#1436=B_SPLINE_CURVE_WITH_KNOTS('',2,(#65070,#65071,#65072),
 .UNSPECIFIED.,.F.,.F.,(3,3),(0.,1.),.UNSPECIFIED.);
#1437=B_SPLINE_CURVE_WITH_KNOTS('',2,(#65074,#65075,#65076),
 .UNSPECIFIED.,.F.,.F.,(3,3),(0.,1.),.UNSPECIFIED.);
#1438=B_SPLINE_CURVE_WITH_KNOTS('',2,(#65078,#65079,#65080),
 .UNSPECIFIED.,.F.,.F.,(3,3),(0.,1.),.UNSPECIFIED.);
#1439=B_SPLINE_CURVE_WITH_KNOTS('',2,(#65082,#65083,#65084),
 .UNSPECIFIED.,.F.,.F.,(3,3),(0.,1.),.UNSPECIFIED.);
#1440=B_SPLINE_CURVE_WITH_KNOTS('',2,(#65086,#65087,#65088),
 .UNSPECIFIED.,.F.,.F.,(3,3),(0.,1.),.UNSPECIFIED.);
#1441=B_SPLINE_CURVE_WITH_KNOTS('',2,(#65089,#65090,#65091),
 .UNSPECIFIED.,.F.,.F.,(3,3),(0.,1.),.UNSPECIFIED.);
#1442=B_SPLINE_CURVE_WITH_KNOTS('',2,(#65130,#65131,#65132),
 .UNSPECIFIED.,.F.,.F.,(3,3),(0.,1.),.UNSPECIFIED.);
#1443=B_SPLINE_CURVE_WITH_KNOTS('',2,(#65134,#65135,#65136),
 .UNSPECIFIED.,.F.,.F.,(3,3),(0.,1.),.UNSPECIFIED.);
#1444=B_SPLINE_CURVE_WITH_KNOTS('',2,(#65140,#65141,#65142),
 .UNSPECIFIED.,.F.,.F.,(3,3),(0.,1.),.UNSPECIFIED.);
#1445=B_SPLINE_CURVE_WITH_KNOTS('',2,(#65144,#65145,#65146),
 .UNSPECIFIED.,.F.,.F.,(3,3),(0.,1.),.UNSPECIFIED.);
#1446=B_SPLINE_CURVE_WITH_KNOTS('',3,(#65197,#65198,#65199,#65200,#65201,
#65202),.UNSPECIFIED.,.F.,.F.,(4,2,4),(0.,0.753367592696704,0.978410263145562),
 .UNSPECIFIED.);
#1447=B_SPLINE_CURVE_WITH_KNOTS('',3,(#65203,#65204,#65205,#65206),
 .UNSPECIFIED.,.F.,.F.,(4,4),(0.978410263146837,1.02480406428257),
 .UNSPECIFIED.);
#1448=B_SPLINE_CURVE_WITH_KNOTS('',3,(#65281,#65282,#65283,#65284,#65285,
#65286,#65287,#65288,#65289,#65290,#65291,#65292,#65293,#65294,#65295,#65296,
#65297,#65298,#65299,#65300),.UNSPECIFIED.,.F.,.F.,(4,2,2,2,2,2,2,2,2,4),
(0.,1.50665307727383,3.01330615454765,4.51995923182148,6.0266123090953,
7.53326538636832,9.03991846364135,10.5465715409144,12.0532246181874,12.0542197677389),
 .UNSPECIFIED.);
#1449=B_SPLINE_CURVE_WITH_KNOTS('',3,(#65302,#65303,#65304,#65305,#65306,
#65307,#65308,#65309,#65310,#65311,#65312,#65313,#65314,#65315,#65316,#65317,
#65318,#65319),.UNSPECIFIED.,.F.,.F.,(4,2,2,2,2,2,2,2,4),(-12.0542237737762,
-10.5474458020542,-9.04066783033219,-7.53388985861016,-6.02711188688813,
-4.5203339151661,-3.01355594344407,-1.50677797172204,0.),.UNSPECIFIED.);
#1450=B_SPLINE_CURVE_WITH_KNOTS('',3,(#65378,#65379,#65380,#65381,#65382,
#65383,#65384,#65385,#65386,#65387),.UNSPECIFIED.,.F.,.F.,(4,2,2,2,4),(3.5397019033151,
3.76683796348352,4.52020555618022,5.27357314887692,6.02694074157362),
 .UNSPECIFIED.);
#1451=B_SPLINE_CURVE_WITH_KNOTS('',3,(#65410,#65411,#65412,#65413,#65414,
#65415,#65416,#65417,#65418,#65419,#65420,#65421,#65422,#65423,#65424,#65425),
 .UNSPECIFIED.,.F.,.F.,(4,2,2,2,2,2,2,4),(0.,1.50665307727383,3.01330615454765,
4.51995923182148,6.02661230909531,7.53326538636833,9.03991846364136,9.06280469595813),
 .UNSPECIFIED.);
#1452=B_SPLINE_CURVE_WITH_KNOTS('',3,(#65431,#65432,#65433,#65434,#65435,
#65436,#65437,#65438,#65439,#65440,#65441,#65442,#65443,#65444,#65445,#65446),
 .UNSPECIFIED.,.F.,.F.,(4,2,2,2,2,2,2,4),(-9.06285135664527,-9.0406678303322,
-7.53388985861017,-6.02711188688814,-4.5203339151661,-3.01355594344407,
-1.50677797172204,0.),.UNSPECIFIED.);
#1453=B_SPLINE_CURVE_WITH_KNOTS('',2,(#65485,#65486,#65487),
 .UNSPECIFIED.,.F.,.F.,(3,3),(-1.,0.),.UNSPECIFIED.);
#1454=B_SPLINE_CURVE_WITH_KNOTS('',2,(#65496,#65497,#65498),
 .UNSPECIFIED.,.F.,.F.,(3,3),(-1.,0.),.UNSPECIFIED.);
#1455=B_SPLINE_CURVE_WITH_KNOTS('',2,(#65511,#65512,#65513),
 .UNSPECIFIED.,.F.,.F.,(3,3),(-1.,0.),.UNSPECIFIED.);
#1456=B_SPLINE_CURVE_WITH_KNOTS('',2,(#65522,#65523,#65524),
 .UNSPECIFIED.,.F.,.F.,(3,3),(-1.,0.),.UNSPECIFIED.);
#1457=B_SPLINE_CURVE_WITH_KNOTS('',2,(#65578,#65579,#65580),
 .UNSPECIFIED.,.F.,.F.,(3,3),(0.,1.),.UNSPECIFIED.);
#1458=B_SPLINE_CURVE_WITH_KNOTS('',2,(#65584,#65585,#65586),
 .UNSPECIFIED.,.F.,.F.,(3,3),(-1.,0.),.UNSPECIFIED.);
#1459=B_SPLINE_CURVE_WITH_KNOTS('',2,(#65595,#65596,#65597),
 .UNSPECIFIED.,.F.,.F.,(3,3),(0.,1.),.UNSPECIFIED.);
#1460=B_SPLINE_CURVE_WITH_KNOTS('',2,(#65599,#65600,#65601),
 .UNSPECIFIED.,.F.,.F.,(3,3),(-1.,0.),.UNSPECIFIED.);
#1461=B_SPLINE_CURVE_WITH_KNOTS('',2,(#65610,#65611,#65612),
 .UNSPECIFIED.,.F.,.F.,(3,3),(0.,1.),.UNSPECIFIED.);
#1462=B_SPLINE_CURVE_WITH_KNOTS('',2,(#65614,#65615,#65616),
 .UNSPECIFIED.,.F.,.F.,(3,3),(-1.,0.),.UNSPECIFIED.);
#1463=B_SPLINE_CURVE_WITH_KNOTS('',2,(#65625,#65626,#65627),
 .UNSPECIFIED.,.F.,.F.,(3,3),(0.,1.),.UNSPECIFIED.);
#1464=B_SPLINE_CURVE_WITH_KNOTS('',2,(#65629,#65630,#65631),
 .UNSPECIFIED.,.F.,.F.,(3,3),(-1.,0.),.UNSPECIFIED.);
#1465=B_SPLINE_CURVE_WITH_KNOTS('',2,(#65640,#65641,#65642),
 .UNSPECIFIED.,.F.,.F.,(3,3),(0.,1.),.UNSPECIFIED.);
#1466=B_SPLINE_CURVE_WITH_KNOTS('',2,(#65644,#65645,#65646),
 .UNSPECIFIED.,.F.,.F.,(3,3),(-1.,0.),.UNSPECIFIED.);
#1467=B_SPLINE_CURVE_WITH_KNOTS('',2,(#65655,#65656,#65657),
 .UNSPECIFIED.,.F.,.F.,(3,3),(0.,1.),.UNSPECIFIED.);
#1468=B_SPLINE_CURVE_WITH_KNOTS('',2,(#65659,#65660,#65661),
 .UNSPECIFIED.,.F.,.F.,(3,3),(-1.,0.),.UNSPECIFIED.);
#1469=B_SPLINE_CURVE_WITH_KNOTS('',2,(#65670,#65671,#65672),
 .UNSPECIFIED.,.F.,.F.,(3,3),(0.,1.),.UNSPECIFIED.);
#1470=B_SPLINE_CURVE_WITH_KNOTS('',2,(#65674,#65675,#65676),
 .UNSPECIFIED.,.F.,.F.,(3,3),(-1.,0.),.UNSPECIFIED.);
#1471=B_SPLINE_CURVE_WITH_KNOTS('',2,(#65684,#65685,#65686),
 .UNSPECIFIED.,.F.,.F.,(3,3),(0.,1.),.UNSPECIFIED.);
#1472=B_SPLINE_CURVE_WITH_KNOTS('',2,(#65687,#65688,#65689),
 .UNSPECIFIED.,.F.,.F.,(3,3),(-1.,0.),.UNSPECIFIED.);
#1473=B_SPLINE_CURVE_WITH_KNOTS('',2,(#65699,#65700,#65701),
 .UNSPECIFIED.,.F.,.F.,(3,3),(-1.,0.),.UNSPECIFIED.);
#1474=B_SPLINE_CURVE_WITH_KNOTS('',2,(#65710,#65711,#65712),
 .UNSPECIFIED.,.F.,.F.,(3,3),(-1.,0.),.UNSPECIFIED.);
#1475=B_SPLINE_CURVE_WITH_KNOTS('',2,(#65721,#65722,#65723),
 .UNSPECIFIED.,.F.,.F.,(3,3),(-1.,0.),.UNSPECIFIED.);
#1476=B_SPLINE_CURVE_WITH_KNOTS('',2,(#65732,#65733,#65734),
 .UNSPECIFIED.,.F.,.F.,(3,3),(-1.,0.),.UNSPECIFIED.);
#1477=B_SPLINE_CURVE_WITH_KNOTS('',2,(#65743,#65744,#65745),
 .UNSPECIFIED.,.F.,.F.,(3,3),(-1.,0.),.UNSPECIFIED.);
#1478=B_SPLINE_CURVE_WITH_KNOTS('',2,(#65754,#65755,#65756),
 .UNSPECIFIED.,.F.,.F.,(3,3),(-1.,0.),.UNSPECIFIED.);
#1479=B_SPLINE_CURVE_WITH_KNOTS('',2,(#65765,#65766,#65767),
 .UNSPECIFIED.,.F.,.F.,(3,3),(-1.,0.),.UNSPECIFIED.);
#1480=B_SPLINE_CURVE_WITH_KNOTS('',2,(#65776,#65777,#65778),
 .UNSPECIFIED.,.F.,.F.,(3,3),(-1.,0.),.UNSPECIFIED.);
#1481=B_SPLINE_CURVE_WITH_KNOTS('',2,(#65787,#65788,#65789),
 .UNSPECIFIED.,.F.,.F.,(3,3),(-1.,0.),.UNSPECIFIED.);
#1482=B_SPLINE_CURVE_WITH_KNOTS('',2,(#65797,#65798,#65799),
 .UNSPECIFIED.,.F.,.F.,(3,3),(-1.,0.),.UNSPECIFIED.);
#2426=PLANE('',#28411);
#2427=PLANE('',#28412);
#2428=PLANE('',#28421);
#2429=PLANE('',#28422);
#2430=PLANE('',#28423);
#2431=PLANE('',#28428);
#2432=PLANE('',#28429);
#2433=PLANE('',#28462);
#2434=PLANE('',#28463);
#2435=PLANE('',#28472);
#2436=PLANE('',#28474);
#2437=PLANE('',#28475);
#2438=PLANE('',#28482);
#2439=PLANE('',#28492);
#2440=PLANE('',#28523);
#2441=PLANE('',#28526);
#2442=PLANE('',#28539);
#2443=PLANE('',#28560);
#2444=PLANE('',#28567);
#2445=PLANE('',#28573);
#2446=PLANE('',#28604);
#2447=PLANE('',#28620);
#2448=PLANE('',#28623);
#2449=PLANE('',#28625);
#2450=PLANE('',#28629);
#2451=PLANE('',#28656);
#2452=PLANE('',#28659);
#2453=PLANE('',#28660);
#2454=PLANE('',#28663);
#2455=PLANE('',#28667);
#2456=PLANE('',#28671);
#2457=PLANE('',#28672);
#2458=PLANE('',#28673);
#2459=PLANE('',#28678);
#2460=PLANE('',#28688);
#2461=PLANE('',#28689);
#2462=PLANE('',#28690);
#2463=PLANE('',#28696);
#2464=PLANE('',#28707);
#2465=PLANE('',#28712);
#2466=PLANE('',#28715);
#2467=PLANE('',#28718);
#2468=PLANE('',#28720);
#2469=PLANE('',#28727);
#2470=PLANE('',#28732);
#2471=PLANE('',#28738);
#2472=PLANE('',#28739);
#2473=PLANE('',#28743);
#2474=PLANE('',#28744);
#2475=PLANE('',#28749);
#2476=PLANE('',#28750);
#2477=PLANE('',#28751);
#2478=PLANE('',#28752);
#2479=PLANE('',#28753);
#2480=PLANE('',#28756);
#2481=PLANE('',#28762);
#2482=PLANE('',#28764);
#2483=PLANE('',#28765);
#2484=PLANE('',#28766);
#2485=PLANE('',#28773);
#2486=PLANE('',#28774);
#2487=PLANE('',#28776);
#2488=PLANE('',#28777);
#2489=PLANE('',#28778);
#2490=PLANE('',#28779);
#2491=PLANE('',#28780);
#2492=PLANE('',#28781);
#2493=PLANE('',#28782);
#2494=PLANE('',#28783);
#2495=PLANE('',#28784);
#2496=PLANE('',#28785);
#2497=PLANE('',#28786);
#2498=PLANE('',#28787);
#2499=PLANE('',#28788);
#2500=PLANE('',#28789);
#2501=PLANE('',#28790);
#2502=PLANE('',#28791);
#2503=PLANE('',#28792);
#2504=PLANE('',#28793);
#2505=PLANE('',#28794);
#2506=PLANE('',#28795);
#2507=PLANE('',#28796);
#2508=PLANE('',#28797);
#2509=PLANE('',#28798);
#2510=PLANE('',#28799);
#2511=PLANE('',#28800);
#2512=PLANE('',#28803);
#2513=PLANE('',#28808);
#2514=PLANE('',#28809);
#2515=PLANE('',#28810);
#2516=PLANE('',#28812);
#2517=PLANE('',#28813);
#2518=PLANE('',#28814);
#2519=PLANE('',#28815);
#2520=PLANE('',#28816);
#2521=PLANE('',#28817);
#2522=PLANE('',#28818);
#2523=PLANE('',#28819);
#2524=PLANE('',#28822);
#2525=PLANE('',#28826);
#2526=PLANE('',#28832);
#2527=PLANE('',#28839);
#2528=PLANE('',#28842);
#2529=PLANE('',#28845);
#2530=PLANE('',#28846);
#2531=PLANE('',#28848);
#2532=PLANE('',#28849);
#2533=PLANE('',#28855);
#2534=PLANE('',#28857);
#2535=PLANE('',#28858);
#2536=PLANE('',#28859);
#2537=PLANE('',#28861);
#2538=PLANE('',#28862);
#2539=PLANE('',#28865);
#2540=PLANE('',#28870);
#2541=PLANE('',#28875);
#2542=PLANE('',#28878);
#2543=PLANE('',#28879);
#2544=PLANE('',#28883);
#2545=PLANE('',#28886);
#2546=PLANE('',#28888);
#2547=PLANE('',#28891);
#3653=FACE_OUTER_BOUND('',#5184,.T.);
#3654=FACE_OUTER_BOUND('',#5185,.T.);
#3655=FACE_OUTER_BOUND('',#5186,.T.);
#3656=FACE_OUTER_BOUND('',#5187,.T.);
#3657=FACE_OUTER_BOUND('',#5188,.T.);
#3658=FACE_OUTER_BOUND('',#5189,.T.);
#3659=FACE_OUTER_BOUND('',#5190,.T.);
#3660=FACE_OUTER_BOUND('',#5191,.T.);
#3661=FACE_OUTER_BOUND('',#5192,.T.);
#3662=FACE_OUTER_BOUND('',#5193,.T.);
#3663=FACE_OUTER_BOUND('',#5194,.T.);
#3664=FACE_OUTER_BOUND('',#5195,.T.);
#3665=FACE_OUTER_BOUND('',#5196,.T.);
#3666=FACE_OUTER_BOUND('',#5197,.T.);
#3667=FACE_OUTER_BOUND('',#5198,.T.);
#3668=FACE_OUTER_BOUND('',#5199,.T.);
#3669=FACE_OUTER_BOUND('',#5200,.T.);
#3670=FACE_OUTER_BOUND('',#5201,.T.);
#3671=FACE_OUTER_BOUND('',#5202,.T.);
#3672=FACE_OUTER_BOUND('',#5203,.T.);
#3673=FACE_OUTER_BOUND('',#5204,.T.);
#3674=FACE_OUTER_BOUND('',#5205,.T.);
#3675=FACE_OUTER_BOUND('',#5206,.T.);
#3676=FACE_OUTER_BOUND('',#5207,.T.);
#3677=FACE_OUTER_BOUND('',#5208,.T.);
#3678=FACE_OUTER_BOUND('',#5209,.T.);
#3679=FACE_OUTER_BOUND('',#5210,.T.);
#3680=FACE_OUTER_BOUND('',#5211,.T.);
#3681=FACE_OUTER_BOUND('',#5212,.T.);
#3682=FACE_OUTER_BOUND('',#5213,.T.);
#3683=FACE_OUTER_BOUND('',#5218,.T.);
#3684=FACE_OUTER_BOUND('',#5220,.T.);
#3685=FACE_OUTER_BOUND('',#5221,.T.);
#3686=FACE_OUTER_BOUND('',#5222,.T.);
#3687=FACE_OUTER_BOUND('',#5223,.T.);
#3688=FACE_OUTER_BOUND('',#5224,.T.);
#3689=FACE_OUTER_BOUND('',#5226,.T.);
#3690=FACE_OUTER_BOUND('',#5227,.T.);
#3691=FACE_OUTER_BOUND('',#5228,.T.);
#3692=FACE_OUTER_BOUND('',#5229,.T.);
#3693=FACE_OUTER_BOUND('',#5231,.T.);
#3694=FACE_OUTER_BOUND('',#5232,.T.);
#3695=FACE_OUTER_BOUND('',#5233,.T.);
#3696=FACE_OUTER_BOUND('',#5234,.T.);
#3697=FACE_OUTER_BOUND('',#5235,.T.);
#3698=FACE_OUTER_BOUND('',#5236,.T.);
#3699=FACE_OUTER_BOUND('',#5237,.T.);
#3700=FACE_OUTER_BOUND('',#5238,.T.);
#3701=FACE_OUTER_BOUND('',#5239,.T.);
#3702=FACE_OUTER_BOUND('',#5240,.T.);
#3703=FACE_OUTER_BOUND('',#5241,.T.);
#3704=FACE_OUTER_BOUND('',#5242,.T.);
#3705=FACE_OUTER_BOUND('',#5243,.T.);
#3706=FACE_OUTER_BOUND('',#5244,.T.);
#3707=FACE_OUTER_BOUND('',#5245,.T.);
#3708=FACE_OUTER_BOUND('',#5246,.T.);
#3709=FACE_OUTER_BOUND('',#5247,.T.);
#3710=FACE_OUTER_BOUND('',#5248,.T.);
#3711=FACE_OUTER_BOUND('',#5249,.T.);
#3712=FACE_OUTER_BOUND('',#5250,.T.);
#3713=FACE_OUTER_BOUND('',#5251,.T.);
#3714=FACE_OUTER_BOUND('',#5253,.T.);
#3715=FACE_OUTER_BOUND('',#5254,.T.);
#3716=FACE_OUTER_BOUND('',#5255,.T.);
#3717=FACE_OUTER_BOUND('',#5256,.T.);
#3718=FACE_OUTER_BOUND('',#5257,.T.);
#3719=FACE_OUTER_BOUND('',#5258,.T.);
#3720=FACE_OUTER_BOUND('',#5259,.T.);
#3721=FACE_OUTER_BOUND('',#5260,.T.);
#3722=FACE_OUTER_BOUND('',#5261,.T.);
#3723=FACE_OUTER_BOUND('',#5262,.T.);
#3724=FACE_OUTER_BOUND('',#5266,.T.);
#3725=FACE_OUTER_BOUND('',#5267,.T.);
#3726=FACE_OUTER_BOUND('',#5268,.T.);
#3727=FACE_OUTER_BOUND('',#5269,.T.);
#3728=FACE_OUTER_BOUND('',#5270,.T.);
#3729=FACE_OUTER_BOUND('',#5271,.T.);
#3730=FACE_OUTER_BOUND('',#5272,.T.);
#3731=FACE_OUTER_BOUND('',#5273,.T.);
#3732=FACE_OUTER_BOUND('',#5274,.T.);
#3733=FACE_OUTER_BOUND('',#5275,.T.);
#3734=FACE_OUTER_BOUND('',#5280,.T.);
#3735=FACE_OUTER_BOUND('',#5281,.T.);
#3736=FACE_OUTER_BOUND('',#5282,.T.);
#3737=FACE_OUTER_BOUND('',#5283,.T.);
#3738=FACE_OUTER_BOUND('',#5284,.T.);
#3739=FACE_OUTER_BOUND('',#5285,.T.);
#3740=FACE_OUTER_BOUND('',#5286,.T.);
#3741=FACE_OUTER_BOUND('',#5287,.T.);
#3742=FACE_OUTER_BOUND('',#5288,.T.);
#3743=FACE_OUTER_BOUND('',#5289,.T.);
#3744=FACE_OUTER_BOUND('',#5296,.T.);
#3745=FACE_OUTER_BOUND('',#5297,.T.);
#3746=FACE_OUTER_BOUND('',#5298,.T.);
#3747=FACE_OUTER_BOUND('',#5299,.T.);
#3748=FACE_OUTER_BOUND('',#5300,.T.);
#3749=FACE_OUTER_BOUND('',#5301,.T.);
#3750=FACE_OUTER_BOUND('',#5302,.T.);
#3751=FACE_OUTER_BOUND('',#5303,.T.);
#3752=FACE_OUTER_BOUND('',#5304,.T.);
#3753=FACE_OUTER_BOUND('',#5305,.T.);
#3754=FACE_OUTER_BOUND('',#5306,.T.);
#3755=FACE_OUTER_BOUND('',#5307,.T.);
#3756=FACE_OUTER_BOUND('',#5308,.T.);
#3757=FACE_OUTER_BOUND('',#5309,.T.);
#3758=FACE_OUTER_BOUND('',#5310,.T.);
#3759=FACE_OUTER_BOUND('',#5311,.T.);
#3760=FACE_OUTER_BOUND('',#5312,.T.);
#3761=FACE_OUTER_BOUND('',#5313,.T.);
#3762=FACE_OUTER_BOUND('',#5314,.T.);
#3763=FACE_OUTER_BOUND('',#5315,.T.);
#3764=FACE_OUTER_BOUND('',#5316,.T.);
#3765=FACE_OUTER_BOUND('',#5317,.T.);
#3766=FACE_OUTER_BOUND('',#5323,.T.);
#3767=FACE_OUTER_BOUND('',#5324,.T.);
#3768=FACE_OUTER_BOUND('',#5325,.T.);
#3769=FACE_OUTER_BOUND('',#5326,.T.);
#3770=FACE_OUTER_BOUND('',#5327,.T.);
#3771=FACE_OUTER_BOUND('',#5328,.T.);
#3772=FACE_OUTER_BOUND('',#5329,.T.);
#3773=FACE_OUTER_BOUND('',#5331,.T.);
#3774=FACE_OUTER_BOUND('',#5332,.T.);
#3775=FACE_OUTER_BOUND('',#5333,.T.);
#3776=FACE_OUTER_BOUND('',#5334,.T.);
#3777=FACE_OUTER_BOUND('',#5335,.T.);
#3778=FACE_OUTER_BOUND('',#5336,.T.);
#3779=FACE_OUTER_BOUND('',#5337,.T.);
#3780=FACE_OUTER_BOUND('',#5338,.T.);
#3781=FACE_OUTER_BOUND('',#5339,.T.);
#3782=FACE_OUTER_BOUND('',#5340,.T.);
#3783=FACE_OUTER_BOUND('',#5341,.T.);
#3784=FACE_OUTER_BOUND('',#5342,.T.);
#3785=FACE_OUTER_BOUND('',#5343,.T.);
#3786=FACE_OUTER_BOUND('',#5344,.T.);
#3787=FACE_OUTER_BOUND('',#5345,.T.);
#3788=FACE_OUTER_BOUND('',#5346,.T.);
#3789=FACE_OUTER_BOUND('',#5347,.T.);
#3790=FACE_OUTER_BOUND('',#5348,.T.);
#3791=FACE_OUTER_BOUND('',#5349,.T.);
#3792=FACE_OUTER_BOUND('',#5350,.T.);
#3793=FACE_OUTER_BOUND('',#5351,.T.);
#3794=FACE_OUTER_BOUND('',#5352,.T.);
#3795=FACE_OUTER_BOUND('',#5353,.T.);
#3796=FACE_OUTER_BOUND('',#5354,.T.);
#3797=FACE_OUTER_BOUND('',#5355,.T.);
#3798=FACE_OUTER_BOUND('',#5356,.T.);
#3799=FACE_OUTER_BOUND('',#5357,.T.);
#3800=FACE_OUTER_BOUND('',#5358,.T.);
#3801=FACE_OUTER_BOUND('',#5359,.T.);
#3802=FACE_OUTER_BOUND('',#5360,.T.);
#3803=FACE_OUTER_BOUND('',#5361,.T.);
#3804=FACE_OUTER_BOUND('',#5362,.T.);
#3805=FACE_OUTER_BOUND('',#5363,.T.);
#3806=FACE_OUTER_BOUND('',#5364,.T.);
#3807=FACE_OUTER_BOUND('',#5365,.T.);
#3808=FACE_OUTER_BOUND('',#5366,.T.);
#3809=FACE_OUTER_BOUND('',#5367,.T.);
#3810=FACE_OUTER_BOUND('',#5368,.T.);
#3811=FACE_OUTER_BOUND('',#5369,.T.);
#3812=FACE_OUTER_BOUND('',#5370,.T.);
#3813=FACE_OUTER_BOUND('',#5371,.T.);
#3814=FACE_OUTER_BOUND('',#5372,.T.);
#3815=FACE_OUTER_BOUND('',#5373,.T.);
#3816=FACE_OUTER_BOUND('',#5374,.T.);
#3817=FACE_OUTER_BOUND('',#5375,.T.);
#3818=FACE_OUTER_BOUND('',#5376,.T.);
#3819=FACE_OUTER_BOUND('',#5377,.T.);
#3820=FACE_OUTER_BOUND('',#5378,.T.);
#3821=FACE_OUTER_BOUND('',#5379,.T.);
#3822=FACE_OUTER_BOUND('',#5380,.T.);
#3823=FACE_OUTER_BOUND('',#5381,.T.);
#3824=FACE_OUTER_BOUND('',#5382,.T.);
#3825=FACE_OUTER_BOUND('',#5383,.T.);
#3826=FACE_OUTER_BOUND('',#5384,.T.);
#3827=FACE_OUTER_BOUND('',#5385,.T.);
#3828=FACE_OUTER_BOUND('',#5386,.T.);
#3829=FACE_OUTER_BOUND('',#5387,.T.);
#3830=FACE_OUTER_BOUND('',#5388,.T.);
#3831=FACE_OUTER_BOUND('',#5389,.T.);
#3832=FACE_OUTER_BOUND('',#5390,.T.);
#3833=FACE_OUTER_BOUND('',#5391,.T.);
#3834=FACE_OUTER_BOUND('',#5392,.T.);
#3835=FACE_OUTER_BOUND('',#5393,.T.);
#3836=FACE_OUTER_BOUND('',#5394,.T.);
#3837=FACE_OUTER_BOUND('',#5395,.T.);
#3838=FACE_OUTER_BOUND('',#5396,.T.);
#3839=FACE_OUTER_BOUND('',#5397,.T.);
#3840=FACE_OUTER_BOUND('',#5398,.T.);
#3841=FACE_OUTER_BOUND('',#5399,.T.);
#3842=FACE_OUTER_BOUND('',#5400,.T.);
#3843=FACE_OUTER_BOUND('',#5401,.T.);
#3844=FACE_OUTER_BOUND('',#5402,.T.);
#3845=FACE_OUTER_BOUND('',#5403,.T.);
#3846=FACE_OUTER_BOUND('',#5404,.T.);
#3847=FACE_OUTER_BOUND('',#5405,.T.);
#3848=FACE_OUTER_BOUND('',#5406,.T.);
#3849=FACE_OUTER_BOUND('',#5407,.T.);
#3850=FACE_OUTER_BOUND('',#5408,.T.);
#3851=FACE_OUTER_BOUND('',#5409,.T.);
#3852=FACE_OUTER_BOUND('',#5410,.T.);
#3853=FACE_OUTER_BOUND('',#5411,.T.);
#3854=FACE_OUTER_BOUND('',#5412,.T.);
#3855=FACE_OUTER_BOUND('',#5413,.T.);
#3856=FACE_OUTER_BOUND('',#5414,.T.);
#3857=FACE_OUTER_BOUND('',#5415,.T.);
#3858=FACE_OUTER_BOUND('',#5416,.T.);
#3859=FACE_OUTER_BOUND('',#5417,.T.);
#3860=FACE_OUTER_BOUND('',#5419,.T.);
#3861=FACE_OUTER_BOUND('',#5420,.T.);
#3862=FACE_OUTER_BOUND('',#5421,.T.);
#3863=FACE_OUTER_BOUND('',#5422,.T.);
#3864=FACE_OUTER_BOUND('',#5423,.T.);
#3865=FACE_OUTER_BOUND('',#5424,.T.);
#3866=FACE_OUTER_BOUND('',#5426,.T.);
#3867=FACE_OUTER_BOUND('',#5427,.T.);
#3868=FACE_OUTER_BOUND('',#5429,.T.);
#3869=FACE_OUTER_BOUND('',#5430,.T.);
#3870=FACE_OUTER_BOUND('',#5431,.T.);
#3871=FACE_OUTER_BOUND('',#5432,.T.);
#3872=FACE_OUTER_BOUND('',#5433,.T.);
#3873=FACE_OUTER_BOUND('',#5434,.T.);
#3874=FACE_OUTER_BOUND('',#5435,.T.);
#3875=FACE_OUTER_BOUND('',#5436,.T.);
#3876=FACE_OUTER_BOUND('',#5437,.T.);
#3877=FACE_OUTER_BOUND('',#5438,.T.);
#3878=FACE_OUTER_BOUND('',#5439,.T.);
#3879=FACE_OUTER_BOUND('',#5440,.T.);
#3880=FACE_OUTER_BOUND('',#5441,.T.);
#3881=FACE_OUTER_BOUND('',#5442,.T.);
#3882=FACE_OUTER_BOUND('',#5443,.T.);
#3883=FACE_OUTER_BOUND('',#5444,.T.);
#3884=FACE_OUTER_BOUND('',#5445,.T.);
#3885=FACE_OUTER_BOUND('',#5447,.T.);
#3886=FACE_OUTER_BOUND('',#5448,.T.);
#3887=FACE_OUTER_BOUND('',#5450,.T.);
#3888=FACE_OUTER_BOUND('',#5451,.T.);
#3889=FACE_OUTER_BOUND('',#5452,.T.);
#3890=FACE_OUTER_BOUND('',#5453,.T.);
#3891=FACE_OUTER_BOUND('',#5454,.T.);
#3892=FACE_OUTER_BOUND('',#5455,.T.);
#3893=FACE_OUTER_BOUND('',#5456,.T.);
#3894=FACE_OUTER_BOUND('',#5457,.T.);
#3895=FACE_OUTER_BOUND('',#5458,.T.);
#3896=FACE_OUTER_BOUND('',#5459,.T.);
#3897=FACE_OUTER_BOUND('',#5460,.T.);
#3898=FACE_OUTER_BOUND('',#5461,.T.);
#3899=FACE_OUTER_BOUND('',#5462,.T.);
#3900=FACE_OUTER_BOUND('',#5463,.T.);
#3901=FACE_OUTER_BOUND('',#5464,.T.);
#3902=FACE_OUTER_BOUND('',#5465,.T.);
#3903=FACE_OUTER_BOUND('',#5466,.T.);
#3904=FACE_OUTER_BOUND('',#5467,.T.);
#3905=FACE_OUTER_BOUND('',#5468,.T.);
#3906=FACE_OUTER_BOUND('',#5469,.T.);
#3907=FACE_OUTER_BOUND('',#5470,.T.);
#3908=FACE_OUTER_BOUND('',#5471,.T.);
#3909=FACE_OUTER_BOUND('',#5472,.T.);
#3910=FACE_OUTER_BOUND('',#5473,.T.);
#3911=FACE_OUTER_BOUND('',#5474,.T.);
#3912=FACE_OUTER_BOUND('',#5475,.T.);
#3913=FACE_OUTER_BOUND('',#5476,.T.);
#3914=FACE_OUTER_BOUND('',#5477,.T.);
#3915=FACE_OUTER_BOUND('',#5478,.T.);
#3916=FACE_OUTER_BOUND('',#5479,.T.);
#3917=FACE_OUTER_BOUND('',#5480,.T.);
#3918=FACE_OUTER_BOUND('',#5481,.T.);
#3919=FACE_OUTER_BOUND('',#5482,.T.);
#3920=FACE_OUTER_BOUND('',#5483,.T.);
#3921=FACE_OUTER_BOUND('',#5484,.T.);
#3922=FACE_OUTER_BOUND('',#5485,.T.);
#3923=FACE_OUTER_BOUND('',#5486,.T.);
#3924=FACE_OUTER_BOUND('',#5487,.T.);
#3925=FACE_OUTER_BOUND('',#5488,.T.);
#3926=FACE_OUTER_BOUND('',#5489,.T.);
#3927=FACE_OUTER_BOUND('',#5490,.T.);
#3928=FACE_OUTER_BOUND('',#5491,.T.);
#3929=FACE_OUTER_BOUND('',#5492,.T.);
#3930=FACE_OUTER_BOUND('',#5493,.T.);
#3931=FACE_OUTER_BOUND('',#5494,.T.);
#3932=FACE_OUTER_BOUND('',#5495,.T.);
#3933=FACE_OUTER_BOUND('',#5496,.T.);
#3934=FACE_OUTER_BOUND('',#5497,.T.);
#5184=EDGE_LOOP('',(#23168,#23169,#23170,#23171,#23172));
#5185=EDGE_LOOP('',(#23173,#23174,#23175,#23176,#23177,#23178));
#5186=EDGE_LOOP('',(#23179,#23180,#23181,#23182,#23183,#23184));
#5187=EDGE_LOOP('',(#23185,#23186,#23187,#23188,#23189));
#5188=EDGE_LOOP('',(#23190,#23191,#23192,#23193));
#5189=EDGE_LOOP('',(#23194,#23195,#23196,#23197,#23198,#23199,#23200,#23201,
#23202));
#5190=EDGE_LOOP('',(#23203,#23204,#23205,#23206,#23207,#23208,#23209,#23210,
#23211,#23212,#23213,#23214));
#5191=EDGE_LOOP('',(#23215,#23216,#23217,#23218,#23219));
#5192=EDGE_LOOP('',(#23220,#23221,#23222,#23223,#23224,#23225));
#5193=EDGE_LOOP('',(#23226,#23227,#23228,#23229));
#5194=EDGE_LOOP('',(#23230,#23231,#23232,#23233));
#5195=EDGE_LOOP('',(#23234,#23235,#23236,#23237,#23238));
#5196=EDGE_LOOP('',(#23239,#23240,#23241,#23242));
#5197=EDGE_LOOP('',(#23243,#23244,#23245,#23246,#23247,#23248));
#5198=EDGE_LOOP('',(#23249,#23250,#23251,#23252,#23253));
#5199=EDGE_LOOP('',(#23254,#23255,#23256));
#5200=EDGE_LOOP('',(#23257,#23258,#23259,#23260));
#5201=EDGE_LOOP('',(#23261,#23262,#23263));
#5202=EDGE_LOOP('',(#23264,#23265,#23266,#23267));
#5203=EDGE_LOOP('',(#23268,#23269,#23270,#23271));
#5204=EDGE_LOOP('',(#23272,#23273,#23274,#23275));
#5205=EDGE_LOOP('',(#23276,#23277,#23278,#23279));
#5206=EDGE_LOOP('',(#23280,#23281,#23282,#23283));
#5207=EDGE_LOOP('',(#23284,#23285,#23286,#23287));
#5208=EDGE_LOOP('',(#23288,#23289,#23290,#23291));
#5209=EDGE_LOOP('',(#23292,#23293,#23294,#23295));
#5210=EDGE_LOOP('',(#23296,#23297,#23298,#23299));
#5211=EDGE_LOOP('',(#23300,#23301,#23302,#23303,#23304));
#5212=EDGE_LOOP('',(#23305,#23306,#23307,#23308,#23309));
#5213=EDGE_LOOP('',(#23310,#23311,#23312,#23313,#23314,#23315,#23316,#23317,
#23318,#23319,#23320,#23321,#23322,#23323,#23324,#23325));
#5214=EDGE_LOOP('',(#23326));
#5215=EDGE_LOOP('',(#23327));
#5216=EDGE_LOOP('',(#23328));
#5217=EDGE_LOOP('',(#23329));
#5218=EDGE_LOOP('',(#23330,#23331,#23332,#23333,#23334,#23335,#23336,#23337));
#5219=EDGE_LOOP('',(#23338));
#5220=EDGE_LOOP('',(#23339,#23340,#23341,#23342));
#5221=EDGE_LOOP('',(#23343,#23344,#23345,#23346));
#5222=EDGE_LOOP('',(#23347,#23348,#23349,#23350));
#5223=EDGE_LOOP('',(#23351,#23352,#23353,#23354));
#5224=EDGE_LOOP('',(#23355));
#5225=EDGE_LOOP('',(#23356));
#5226=EDGE_LOOP('',(#23357,#23358,#23359,#23360));
#5227=EDGE_LOOP('',(#23361,#23362,#23363,#23364));
#5228=EDGE_LOOP('',(#23365,#23366,#23367,#23368));
#5229=EDGE_LOOP('',(#23369));
#5230=EDGE_LOOP('',(#23370));
#5231=EDGE_LOOP('',(#23371,#23372,#23373,#23374));
#5232=EDGE_LOOP('',(#23375,#23376,#23377,#23378));
#5233=EDGE_LOOP('',(#23379,#23380,#23381,#23382));
#5234=EDGE_LOOP('',(#23383,#23384,#23385,#23386));
#5235=EDGE_LOOP('',(#23387,#23388,#23389,#23390));
#5236=EDGE_LOOP('',(#23391,#23392,#23393));
#5237=EDGE_LOOP('',(#23394,#23395,#23396));
#5238=EDGE_LOOP('',(#23397,#23398,#23399,#23400));
#5239=EDGE_LOOP('',(#23401,#23402,#23403,#23404));
#5240=EDGE_LOOP('',(#23405,#23406,#23407,#23408));
#5241=EDGE_LOOP('',(#23409,#23410,#23411,#23412));
#5242=EDGE_LOOP('',(#23413,#23414,#23415,#23416));
#5243=EDGE_LOOP('',(#23417,#23418,#23419,#23420,#23421,#23422));
#5244=EDGE_LOOP('',(#23423,#23424,#23425,#23426,#23427,#23428,#23429,#23430));
#5245=EDGE_LOOP('',(#23431,#23432,#23433,#23434));
#5246=EDGE_LOOP('',(#23435,#23436,#23437,#23438,#23439,#23440));
#5247=EDGE_LOOP('',(#23441,#23442,#23443));
#5248=EDGE_LOOP('',(#23444,#23445,#23446,#23447,#23448,#23449,#23450,#23451,
#23452,#23453,#23454));
#5249=EDGE_LOOP('',(#23455,#23456,#23457,#23458,#23459,#23460));
#5250=EDGE_LOOP('',(#23461,#23462,#23463,#23464));
#5251=EDGE_LOOP('',(#23465,#23466,#23467,#23468,#23469,#23470,#23471,#23472));
#5252=EDGE_LOOP('',(#23473,#23474,#23475,#23476));
#5253=EDGE_LOOP('',(#23477,#23478,#23479,#23480,#23481,#23482));
#5254=EDGE_LOOP('',(#23483,#23484,#23485,#23486));
#5255=EDGE_LOOP('',(#23487,#23488,#23489));
#5256=EDGE_LOOP('',(#23490,#23491,#23492,#23493));
#5257=EDGE_LOOP('',(#23494,#23495,#23496,#23497,#23498,#23499));
#5258=EDGE_LOOP('',(#23500,#23501,#23502,#23503,#23504,#23505,#23506,#23507,
#23508,#23509,#23510));
#5259=EDGE_LOOP('',(#23511,#23512,#23513,#23514));
#5260=EDGE_LOOP('',(#23515,#23516,#23517,#23518,#23519,#23520));
#5261=EDGE_LOOP('',(#23521,#23522,#23523,#23524,#23525));
#5262=EDGE_LOOP('',(#23526,#23527,#23528,#23529,#23530,#23531,#23532,#23533,
#23534,#23535,#23536));
#5263=EDGE_LOOP('',(#23537));
#5264=EDGE_LOOP('',(#23538));
#5265=EDGE_LOOP('',(#23539));
#5266=EDGE_LOOP('',(#23540,#23541,#23542,#23543,#23544));
#5267=EDGE_LOOP('',(#23545,#23546,#23547,#23548,#23549));
#5268=EDGE_LOOP('',(#23550,#23551,#23552,#23553,#23554));
#5269=EDGE_LOOP('',(#23555,#23556,#23557,#23558,#23559));
#5270=EDGE_LOOP('',(#23560,#23561,#23562,#23563,#23564));
#5271=EDGE_LOOP('',(#23565,#23566,#23567,#23568,#23569,#23570,#23571));
#5272=EDGE_LOOP('',(#23572,#23573,#23574,#23575,#23576,#23577,#23578,#23579,
#23580,#23581));
#5273=EDGE_LOOP('',(#23582,#23583,#23584,#23585,#23586));
#5274=EDGE_LOOP('',(#23587,#23588,#23589,#23590,#23591,#23592));
#5275=EDGE_LOOP('',(#23593,#23594,#23595,#23596,#23597,#23598,#23599,#23600,
#23601,#23602));
#5276=EDGE_LOOP('',(#23603));
#5277=EDGE_LOOP('',(#23604));
#5278=EDGE_LOOP('',(#23605));
#5279=EDGE_LOOP('',(#23606));
#5280=EDGE_LOOP('',(#23607,#23608,#23609,#23610));
#5281=EDGE_LOOP('',(#23611,#23612,#23613,#23614,#23615));
#5282=EDGE_LOOP('',(#23616,#23617,#23618,#23619));
#5283=EDGE_LOOP('',(#23620,#23621,#23622,#23623));
#5284=EDGE_LOOP('',(#23624,#23625,#23626,#23627));
#5285=EDGE_LOOP('',(#23628,#23629,#23630,#23631));
#5286=EDGE_LOOP('',(#23632,#23633,#23634,#23635));
#5287=EDGE_LOOP('',(#23636,#23637,#23638,#23639));
#5288=EDGE_LOOP('',(#23640,#23641,#23642,#23643,#23644));
#5289=EDGE_LOOP('',(#23645,#23646,#23647,#23648,#23649,#23650,#23651,#23652,
#23653,#23654,#23655,#23656));
#5290=EDGE_LOOP('',(#23657));
#5291=EDGE_LOOP('',(#23658));
#5292=EDGE_LOOP('',(#23659));
#5293=EDGE_LOOP('',(#23660));
#5294=EDGE_LOOP('',(#23661,#23662,#23663,#23664,#23665,#23666,#23667,#23668,
#23669,#23670,#23671,#23672));
#5295=EDGE_LOOP('',(#23673));
#5296=EDGE_LOOP('',(#23674,#23675,#23676,#23677,#23678,#23679));
#5297=EDGE_LOOP('',(#23680,#23681,#23682,#23683));
#5298=EDGE_LOOP('',(#23684,#23685,#23686,#23687));
#5299=EDGE_LOOP('',(#23688,#23689,#23690,#23691));
#5300=EDGE_LOOP('',(#23692,#23693,#23694,#23695));
#5301=EDGE_LOOP('',(#23696,#23697,#23698,#23699,#23700,#23701,#23702,#23703));
#5302=EDGE_LOOP('',(#23704,#23705,#23706,#23707,#23708));
#5303=EDGE_LOOP('',(#23709,#23710,#23711,#23712,#23713,#23714));
#5304=EDGE_LOOP('',(#23715,#23716,#23717,#23718));
#5305=EDGE_LOOP('',(#23719,#23720,#23721,#23722,#23723,#23724,#23725,#23726,
#23727,#23728));
#5306=EDGE_LOOP('',(#23729,#23730,#23731,#23732));
#5307=EDGE_LOOP('',(#23733,#23734,#23735,#23736,#23737));
#5308=EDGE_LOOP('',(#23738,#23739,#23740,#23741,#23742,#23743));
#5309=EDGE_LOOP('',(#23744,#23745,#23746,#23747,#23748));
#5310=EDGE_LOOP('',(#23749,#23750,#23751,#23752,#23753,#23754));
#5311=EDGE_LOOP('',(#23755,#23756,#23757,#23758,#23759));
#5312=EDGE_LOOP('',(#23760,#23761,#23762,#23763,#23764,#23765));
#5313=EDGE_LOOP('',(#23766,#23767,#23768,#23769));
#5314=EDGE_LOOP('',(#23770,#23771,#23772,#23773,#23774));
#5315=EDGE_LOOP('',(#23775,#23776,#23777,#23778,#23779,#23780));
#5316=EDGE_LOOP('',(#23781,#23782,#23783,#23784));
#5317=EDGE_LOOP('',(#23785,#23786,#23787,#23788,#23789,#23790,#23791,#23792,
#23793,#23794,#23795,#23796,#23797,#23798,#23799,#23800,#23801,#23802,#23803,
#23804));
#5318=EDGE_LOOP('',(#23805,#23806,#23807,#23808,#23809,#23810,#23811,#23812,
#23813,#23814));
#5319=EDGE_LOOP('',(#23815,#23816,#23817,#23818));
#5320=EDGE_LOOP('',(#23819));
#5321=EDGE_LOOP('',(#23820,#23821,#23822,#23823,#23824,#23825,#23826,#23827,
#23828,#23829));
#5322=EDGE_LOOP('',(#23830,#23831,#23832,#23833,#23834,#23835,#23836,#23837,
#23838));
#5323=EDGE_LOOP('',(#23839,#23840,#23841,#23842,#23843));
#5324=EDGE_LOOP('',(#23844,#23845,#23846,#23847));
#5325=EDGE_LOOP('',(#23848,#23849,#23850,#23851,#23852));
#5326=EDGE_LOOP('',(#23853,#23854,#23855,#23856));
#5327=EDGE_LOOP('',(#23857,#23858,#23859,#23860));
#5328=EDGE_LOOP('',(#23861,#23862,#23863,#23864));
#5329=EDGE_LOOP('',(#23865,#23866,#23867,#23868,#23869,#23870,#23871,#23872,
#23873,#23874,#23875,#23876,#23877,#23878,#23879,#23880,#23881,#23882,#23883,
#23884));
#5330=EDGE_LOOP('',(#23885));
#5331=EDGE_LOOP('',(#23886,#23887,#23888,#23889,#23890,#23891));
#5332=EDGE_LOOP('',(#23892,#23893,#23894,#23895,#23896));
#5333=EDGE_LOOP('',(#23897,#23898,#23899,#23900));
#5334=EDGE_LOOP('',(#23901,#23902,#23903,#23904));
#5335=EDGE_LOOP('',(#23905,#23906,#23907,#23908));
#5336=EDGE_LOOP('',(#23909,#23910,#23911,#23912,#23913,#23914));
#5337=EDGE_LOOP('',(#23915,#23916,#23917,#23918,#23919,#23920));
#5338=EDGE_LOOP('',(#23921,#23922,#23923));
#5339=EDGE_LOOP('',(#23924,#23925,#23926));
#5340=EDGE_LOOP('',(#23927,#23928,#23929,#23930,#23931,#23932));
#5341=EDGE_LOOP('',(#23933,#23934,#23935,#23936,#23937,#23938));
#5342=EDGE_LOOP('',(#23939,#23940,#23941,#23942,#23943));
#5343=EDGE_LOOP('',(#23944,#23945,#23946,#23947));
#5344=EDGE_LOOP('',(#23948,#23949,#23950));
#5345=EDGE_LOOP('',(#23951,#23952,#23953,#23954));
#5346=EDGE_LOOP('',(#23955,#23956,#23957,#23958,#23959,#23960));
#5347=EDGE_LOOP('',(#23961,#23962,#23963));
#5348=EDGE_LOOP('',(#23964,#23965,#23966));
#5349=EDGE_LOOP('',(#23967,#23968,#23969,#23970));
#5350=EDGE_LOOP('',(#23971,#23972,#23973,#23974));
#5351=EDGE_LOOP('',(#23975,#23976,#23977,#23978));
#5352=EDGE_LOOP('',(#23979,#23980,#23981,#23982));
#5353=EDGE_LOOP('',(#23983,#23984,#23985,#23986));
#5354=EDGE_LOOP('',(#23987,#23988,#23989,#23990,#23991,#23992,#23993,#23994));
#5355=EDGE_LOOP('',(#23995,#23996,#23997,#23998));
#5356=EDGE_LOOP('',(#23999,#24000,#24001,#24002));
#5357=EDGE_LOOP('',(#24003,#24004,#24005,#24006));
#5358=EDGE_LOOP('',(#24007,#24008,#24009,#24010));
#5359=EDGE_LOOP('',(#24011,#24012,#24013,#24014,#24015,#24016,#24017,#24018));
#5360=EDGE_LOOP('',(#24019,#24020,#24021,#24022));
#5361=EDGE_LOOP('',(#24023,#24024,#24025,#24026));
#5362=EDGE_LOOP('',(#24027,#24028,#24029,#24030));
#5363=EDGE_LOOP('',(#24031,#24032,#24033,#24034,#24035,#24036));
#5364=EDGE_LOOP('',(#24037,#24038,#24039,#24040));
#5365=EDGE_LOOP('',(#24041,#24042,#24043,#24044,#24045,#24046,#24047,#24048));
#5366=EDGE_LOOP('',(#24049,#24050,#24051,#24052,#24053,#24054));
#5367=EDGE_LOOP('',(#24055,#24056,#24057,#24058));
#5368=EDGE_LOOP('',(#24059,#24060,#24061,#24062,#24063));
#5369=EDGE_LOOP('',(#24064,#24065,#24066,#24067));
#5370=EDGE_LOOP('',(#24068,#24069,#24070,#24071));
#5371=EDGE_LOOP('',(#24072,#24073,#24074,#24075));
#5372=EDGE_LOOP('',(#24076,#24077,#24078,#24079));
#5373=EDGE_LOOP('',(#24080,#24081,#24082,#24083));
#5374=EDGE_LOOP('',(#24084,#24085,#24086,#24087,#24088,#24089));
#5375=EDGE_LOOP('',(#24090,#24091,#24092,#24093,#24094,#24095,#24096,#24097,
#24098,#24099));
#5376=EDGE_LOOP('',(#24100,#24101,#24102,#24103,#24104,#24105));
#5377=EDGE_LOOP('',(#24106,#24107,#24108,#24109));
#5378=EDGE_LOOP('',(#24110,#24111,#24112,#24113));
#5379=EDGE_LOOP('',(#24114,#24115,#24116,#24117));
#5380=EDGE_LOOP('',(#24118,#24119,#24120,#24121));
#5381=EDGE_LOOP('',(#24122,#24123,#24124,#24125));
#5382=EDGE_LOOP('',(#24126,#24127,#24128,#24129));
#5383=EDGE_LOOP('',(#24130,#24131,#24132,#24133));
#5384=EDGE_LOOP('',(#24134,#24135,#24136,#24137));
#5385=EDGE_LOOP('',(#24138,#24139,#24140,#24141));
#5386=EDGE_LOOP('',(#24142,#24143,#24144,#24145));
#5387=EDGE_LOOP('',(#24146,#24147,#24148,#24149,#24150,#24151,#24152,#24153,
#24154));
#5388=EDGE_LOOP('',(#24155,#24156,#24157,#24158));
#5389=EDGE_LOOP('',(#24159,#24160,#24161,#24162));
#5390=EDGE_LOOP('',(#24163,#24164,#24165,#24166));
#5391=EDGE_LOOP('',(#24167,#24168,#24169,#24170));
#5392=EDGE_LOOP('',(#24171,#24172,#24173,#24174));
#5393=EDGE_LOOP('',(#24175,#24176,#24177,#24178));
#5394=EDGE_LOOP('',(#24179,#24180,#24181,#24182));
#5395=EDGE_LOOP('',(#24183,#24184,#24185,#24186));
#5396=EDGE_LOOP('',(#24187,#24188,#24189,#24190));
#5397=EDGE_LOOP('',(#24191,#24192,#24193,#24194));
#5398=EDGE_LOOP('',(#24195,#24196,#24197,#24198,#24199,#24200,#24201,#24202,
#24203,#24204));
#5399=EDGE_LOOP('',(#24205,#24206,#24207,#24208));
#5400=EDGE_LOOP('',(#24209,#24210,#24211,#24212));
#5401=EDGE_LOOP('',(#24213,#24214,#24215,#24216));
#5402=EDGE_LOOP('',(#24217,#24218,#24219,#24220));
#5403=EDGE_LOOP('',(#24221,#24222,#24223,#24224));
#5404=EDGE_LOOP('',(#24225,#24226,#24227,#24228));
#5405=EDGE_LOOP('',(#24229,#24230,#24231,#24232));
#5406=EDGE_LOOP('',(#24233,#24234,#24235,#24236));
#5407=EDGE_LOOP('',(#24237,#24238,#24239,#24240));
#5408=EDGE_LOOP('',(#24241,#24242,#24243,#24244));
#5409=EDGE_LOOP('',(#24245,#24246,#24247,#24248));
#5410=EDGE_LOOP('',(#24249,#24250,#24251,#24252));
#5411=EDGE_LOOP('',(#24253,#24254,#24255,#24256));
#5412=EDGE_LOOP('',(#24257,#24258,#24259,#24260));
#5413=EDGE_LOOP('',(#24261,#24262,#24263,#24264));
#5414=EDGE_LOOP('',(#24265,#24266,#24267,#24268));
#5415=EDGE_LOOP('',(#24269,#24270,#24271,#24272));
#5416=EDGE_LOOP('',(#24273,#24274,#24275,#24276));
#5417=EDGE_LOOP('',(#24277,#24278,#24279,#24280,#24281,#24282,#24283,#24284,
#24285,#24286));
#5418=EDGE_LOOP('',(#24287,#24288,#24289,#24290,#24291,#24292,#24293,#24294));
#5419=EDGE_LOOP('',(#24295,#24296,#24297,#24298));
#5420=EDGE_LOOP('',(#24299,#24300,#24301,#24302));
#5421=EDGE_LOOP('',(#24303,#24304,#24305,#24306));
#5422=EDGE_LOOP('',(#24307,#24308,#24309,#24310));
#5423=EDGE_LOOP('',(#24311,#24312,#24313,#24314));
#5424=EDGE_LOOP('',(#24315));
#5425=EDGE_LOOP('',(#24316));
#5426=EDGE_LOOP('',(#24317,#24318,#24319,#24320));
#5427=EDGE_LOOP('',(#24321));
#5428=EDGE_LOOP('',(#24322));
#5429=EDGE_LOOP('',(#24323,#24324,#24325,#24326));
#5430=EDGE_LOOP('',(#24327,#24328,#24329,#24330));
#5431=EDGE_LOOP('',(#24331,#24332,#24333,#24334));
#5432=EDGE_LOOP('',(#24335,#24336,#24337,#24338));
#5433=EDGE_LOOP('',(#24339,#24340,#24341,#24342));
#5434=EDGE_LOOP('',(#24343,#24344,#24345,#24346));
#5435=EDGE_LOOP('',(#24347,#24348,#24349,#24350));
#5436=EDGE_LOOP('',(#24351,#24352,#24353,#24354,#24355));
#5437=EDGE_LOOP('',(#24356,#24357,#24358,#24359));
#5438=EDGE_LOOP('',(#24360,#24361,#24362,#24363));
#5439=EDGE_LOOP('',(#24364,#24365,#24366,#24367,#24368));
#5440=EDGE_LOOP('',(#24369,#24370,#24371,#24372,#24373,#24374,#24375,#24376,
#24377));
#5441=EDGE_LOOP('',(#24378,#24379,#24380,#24381));
#5442=EDGE_LOOP('',(#24382,#24383,#24384,#24385,#24386));
#5443=EDGE_LOOP('',(#24387,#24388,#24389,#24390));
#5444=EDGE_LOOP('',(#24391,#24392,#24393,#24394));
#5445=EDGE_LOOP('',(#24395));
#5446=EDGE_LOOP('',(#24396));
#5447=EDGE_LOOP('',(#24397,#24398,#24399,#24400));
#5448=EDGE_LOOP('',(#24401));
#5449=EDGE_LOOP('',(#24402));
#5450=EDGE_LOOP('',(#24403,#24404,#24405,#24406));
#5451=EDGE_LOOP('',(#24407,#24408,#24409,#24410));
#5452=EDGE_LOOP('',(#24411,#24412,#24413,#24414,#24415,#24416,#24417,#24418));
#5453=EDGE_LOOP('',(#24419,#24420,#24421,#24422));
#5454=EDGE_LOOP('',(#24423,#24424,#24425,#24426));
#5455=EDGE_LOOP('',(#24427,#24428,#24429,#24430));
#5456=EDGE_LOOP('',(#24431,#24432,#24433,#24434));
#5457=EDGE_LOOP('',(#24435,#24436,#24437,#24438,#24439,#24440));
#5458=EDGE_LOOP('',(#24441,#24442,#24443,#24444));
#5459=EDGE_LOOP('',(#24445,#24446,#24447,#24448));
#5460=EDGE_LOOP('',(#24449,#24450,#24451,#24452));
#5461=EDGE_LOOP('',(#24453,#24454,#24455,#24456));
#5462=EDGE_LOOP('',(#24457,#24458,#24459,#24460));
#5463=EDGE_LOOP('',(#24461,#24462,#24463,#24464));
#5464=EDGE_LOOP('',(#24465,#24466,#24467,#24468,#24469));
#5465=EDGE_LOOP('',(#24470,#24471,#24472,#24473,#24474,#24475));
#5466=EDGE_LOOP('',(#24476,#24477,#24478,#24479,#24480,#24481));
#5467=EDGE_LOOP('',(#24482,#24483,#24484,#24485));
#5468=EDGE_LOOP('',(#24486,#24487,#24488));
#5469=EDGE_LOOP('',(#24489,#24490,#24491,#24492,#24493,#24494));
#5470=EDGE_LOOP('',(#24495,#24496,#24497,#24498));
#5471=EDGE_LOOP('',(#24499,#24500,#24501,#24502,#24503));
#5472=EDGE_LOOP('',(#24504,#24505,#24506,#24507));
#5473=EDGE_LOOP('',(#24508,#24509,#24510,#24511));
#5474=EDGE_LOOP('',(#24512,#24513,#24514,#24515));
#5475=EDGE_LOOP('',(#24516,#24517,#24518,#24519));
#5476=EDGE_LOOP('',(#24520,#24521,#24522,#24523));
#5477=EDGE_LOOP('',(#24524,#24525,#24526,#24527));
#5478=EDGE_LOOP('',(#24528,#24529,#24530,#24531));
#5479=EDGE_LOOP('',(#24532,#24533,#24534,#24535));
#5480=EDGE_LOOP('',(#24536,#24537,#24538,#24539));
#5481=EDGE_LOOP('',(#24540,#24541,#24542,#24543));
#5482=EDGE_LOOP('',(#24544,#24545,#24546,#24547));
#5483=EDGE_LOOP('',(#24548,#24549,#24550,#24551));
#5484=EDGE_LOOP('',(#24552,#24553,#24554,#24555));
#5485=EDGE_LOOP('',(#24556,#24557,#24558,#24559));
#5486=EDGE_LOOP('',(#24560,#24561,#24562,#24563));
#5487=EDGE_LOOP('',(#24564,#24565,#24566,#24567,#24568,#24569,#24570,#24571,
#24572,#24573));
#5488=EDGE_LOOP('',(#24574,#24575,#24576,#24577));
#5489=EDGE_LOOP('',(#24578,#24579,#24580,#24581));
#5490=EDGE_LOOP('',(#24582,#24583,#24584,#24585));
#5491=EDGE_LOOP('',(#24586,#24587,#24588,#24589));
#5492=EDGE_LOOP('',(#24590,#24591,#24592,#24593));
#5493=EDGE_LOOP('',(#24594,#24595,#24596,#24597));
#5494=EDGE_LOOP('',(#24598,#24599,#24600,#24601));
#5495=EDGE_LOOP('',(#24602,#24603,#24604,#24605));
#5496=EDGE_LOOP('',(#24606,#24607,#24608,#24609));
#5497=EDGE_LOOP('',(#24610,#24611,#24612,#24613));
#7613=LINE('',#63969,#10110);
#7614=LINE('',#63972,#10111);
#7615=LINE('',#63989,#10112);
#7616=LINE('',#63993,#10113);
#7617=LINE('',#64017,#10114);
#7618=LINE('',#64019,#10115);
#7619=LINE('',#64020,#10116);
#7620=LINE('',#64023,#10117);
#7621=LINE('',#64025,#10118);
#7622=LINE('',#64027,#10119);
#7623=LINE('',#64030,#10120);
#7624=LINE('',#64034,#10121);
#7625=LINE('',#64036,#10122);
#7626=LINE('',#64043,#10123);
#7627=LINE('',#64047,#10124);
#7628=LINE('',#64051,#10125);
#7629=LINE('',#64053,#10126);
#7630=LINE('',#64055,#10127);
#7631=LINE('',#64057,#10128);
#7632=LINE('',#64058,#10129);
#7633=LINE('',#64061,#10130);
#7634=LINE('',#64063,#10131);
#7635=LINE('',#64064,#10132);
#7636=LINE('',#64067,#10133);
#7637=LINE('',#64068,#10134);
#7638=LINE('',#64074,#10135);
#7639=LINE('',#64079,#10136);
#7640=LINE('',#64082,#10137);
#7641=LINE('',#64084,#10138);
#7642=LINE('',#64085,#10139);
#7643=LINE('',#64088,#10140);
#7644=LINE('',#64090,#10141);
#7645=LINE('',#64092,#10142);
#7646=LINE('',#64094,#10143);
#7647=LINE('',#64095,#10144);
#7648=LINE('',#64100,#10145);
#7649=LINE('',#64110,#10146);
#7650=LINE('',#64119,#10147);
#7651=LINE('',#64123,#10148);
#7652=LINE('',#64126,#10149);
#7653=LINE('',#64127,#10150);
#7654=LINE('',#64130,#10151);
#7655=LINE('',#64134,#10152);
#7656=LINE('',#64136,#10153);
#7657=LINE('',#64140,#10154);
#7658=LINE('',#64148,#10155);
#7659=LINE('',#64151,#10156);
#7660=LINE('',#64153,#10157);
#7661=LINE('',#64156,#10158);
#7662=LINE('',#64157,#10159);
#7663=LINE('',#64160,#10160);
#7664=LINE('',#64164,#10161);
#7665=LINE('',#64165,#10162);
#7666=LINE('',#64168,#10163);
#7667=LINE('',#64172,#10164);
#7668=LINE('',#64176,#10165);
#7669=LINE('',#64180,#10166);
#7670=LINE('',#64192,#10167);
#7671=LINE('',#64194,#10168);
#7672=LINE('',#64196,#10169);
#7673=LINE('',#64198,#10170);
#7674=LINE('',#64199,#10171);
#7675=LINE('',#64203,#10172);
#7676=LINE('',#64205,#10173);
#7677=LINE('',#64215,#10174);
#7678=LINE('',#64230,#10175);
#7679=LINE('',#64242,#10176);
#7680=LINE('',#64250,#10177);
#7681=LINE('',#64267,#10178);
#7682=LINE('',#64268,#10179);
#7683=LINE('',#64282,#10180);
#7684=LINE('',#64283,#10181);
#7685=LINE('',#64335,#10182);
#7686=LINE('',#64336,#10183);
#7687=LINE('',#64341,#10184);
#7688=LINE('',#64344,#10185);
#7689=LINE('',#64347,#10186);
#7690=LINE('',#64349,#10187);
#7691=LINE('',#64351,#10188);
#7692=LINE('',#64353,#10189);
#7693=LINE('',#64354,#10190);
#7694=LINE('',#64369,#10191);
#7695=LINE('',#64372,#10192);
#7696=LINE('',#64383,#10193);
#7697=LINE('',#64387,#10194);
#7698=LINE('',#64389,#10195);
#7699=LINE('',#64396,#10196);
#7700=LINE('',#64407,#10197);
#7701=LINE('',#64411,#10198);
#7702=LINE('',#64421,#10199);
#7703=LINE('',#64426,#10200);
#7704=LINE('',#64428,#10201);
#7705=LINE('',#64429,#10202);
#7706=LINE('',#64438,#10203);
#7707=LINE('',#64442,#10204);
#7708=LINE('',#64445,#10205);
#7709=LINE('',#64450,#10206);
#7710=LINE('',#64453,#10207);
#7711=LINE('',#64464,#10208);
#7712=LINE('',#64468,#10209);
#7713=LINE('',#64483,#10210);
#7714=LINE('',#64485,#10211);
#7715=LINE('',#64496,#10212);
#7716=LINE('',#64498,#10213);
#7717=LINE('',#64499,#10214);
#7718=LINE('',#64502,#10215);
#7719=LINE('',#64513,#10216);
#7720=LINE('',#64517,#10217);
#7721=LINE('',#64527,#10218);
#7722=LINE('',#64541,#10219);
#7723=LINE('',#64561,#10220);
#7724=LINE('',#64563,#10221);
#7725=LINE('',#64565,#10222);
#7726=LINE('',#64585,#10223);
#7727=LINE('',#64587,#10224);
#7728=LINE('',#64589,#10225);
#7729=LINE('',#64590,#10226);
#7730=LINE('',#64592,#10227);
#7731=LINE('',#64594,#10228);
#7732=LINE('',#64596,#10229);
#7733=LINE('',#64598,#10230);
#7734=LINE('',#64607,#10231);
#7735=LINE('',#64617,#10232);
#7736=LINE('',#64627,#10233);
#7737=LINE('',#64665,#10234);
#7738=LINE('',#64669,#10235);
#7739=LINE('',#64673,#10236);
#7740=LINE('',#64695,#10237);
#7741=LINE('',#64730,#10238);
#7742=LINE('',#64734,#10239);
#7743=LINE('',#64736,#10240);
#7744=LINE('',#64738,#10241);
#7745=LINE('',#64740,#10242);
#7746=LINE('',#64741,#10243);
#7747=LINE('',#64743,#10244);
#7748=LINE('',#64745,#10245);
#7749=LINE('',#64746,#10246);
#7750=LINE('',#64761,#10247);
#7751=LINE('',#64802,#10248);
#7752=LINE('',#64805,#10249);
#7753=LINE('',#64808,#10250);
#7754=LINE('',#64810,#10251);
#7755=LINE('',#64811,#10252);
#7756=LINE('',#64846,#10253);
#7757=LINE('',#64849,#10254);
#7758=LINE('',#64852,#10255);
#7759=LINE('',#64853,#10256);
#7760=LINE('',#64863,#10257);
#7761=LINE('',#64867,#10258);
#7762=LINE('',#64871,#10259);
#7763=LINE('',#64883,#10260);
#7764=LINE('',#64885,#10261);
#7765=LINE('',#64887,#10262);
#7766=LINE('',#64888,#10263);
#7767=LINE('',#64889,#10264);
#7768=LINE('',#64891,#10265);
#7769=LINE('',#64893,#10266);
#7770=LINE('',#64895,#10267);
#7771=LINE('',#64897,#10268);
#7772=LINE('',#64898,#10269);
#7773=LINE('',#64899,#10270);
#7774=LINE('',#64918,#10271);
#7775=LINE('',#64922,#10272);
#7776=LINE('',#64931,#10273);
#7777=LINE('',#64939,#10274);
#7778=LINE('',#64942,#10275);
#7779=LINE('',#64945,#10276);
#7780=LINE('',#64947,#10277);
#7781=LINE('',#64948,#10278);
#7782=LINE('',#64961,#10279);
#7783=LINE('',#64963,#10280);
#7784=LINE('',#64964,#10281);
#7785=LINE('',#64966,#10282);
#7786=LINE('',#64968,#10283);
#7787=LINE('',#64969,#10284);
#7788=LINE('',#64971,#10285);
#7789=LINE('',#64976,#10286);
#7790=LINE('',#64983,#10287);
#7791=LINE('',#64988,#10288);
#7792=LINE('',#64990,#10289);
#7793=LINE('',#64991,#10290);
#7794=LINE('',#64993,#10291);
#7795=LINE('',#64999,#10292);
#7796=LINE('',#65013,#10293);
#7797=LINE('',#65019,#10294);
#7798=LINE('',#65032,#10295);
#7799=LINE('',#65036,#10296);
#7800=LINE('',#65040,#10297);
#7801=LINE('',#65043,#10298);
#7802=LINE('',#65048,#10299);
#7803=LINE('',#65051,#10300);
#7804=LINE('',#65094,#10301);
#7805=LINE('',#65096,#10302);
#7806=LINE('',#65098,#10303);
#7807=LINE('',#65099,#10304);
#7808=LINE('',#65104,#10305);
#7809=LINE('',#65106,#10306);
#7810=LINE('',#65108,#10307);
#7811=LINE('',#65110,#10308);
#7812=LINE('',#65112,#10309);
#7813=LINE('',#65114,#10310);
#7814=LINE('',#65116,#10311);
#7815=LINE('',#65118,#10312);
#7816=LINE('',#65120,#10313);
#7817=LINE('',#65121,#10314);
#7818=LINE('',#65124,#10315);
#7819=LINE('',#65126,#10316);
#7820=LINE('',#65128,#10317);
#7821=LINE('',#65138,#10318);
#7822=LINE('',#65147,#10319);
#7823=LINE('',#65153,#10320);
#7824=LINE('',#65158,#10321);
#7825=LINE('',#65163,#10322);
#7826=LINE('',#65168,#10323);
#7827=LINE('',#65171,#10324);
#7828=LINE('',#65175,#10325);
#7829=LINE('',#65179,#10326);
#7830=LINE('',#65183,#10327);
#7831=LINE('',#65188,#10328);
#7832=LINE('',#65191,#10329);
#7833=LINE('',#65195,#10330);
#7834=LINE('',#65212,#10331);
#7835=LINE('',#65217,#10332);
#7836=LINE('',#65220,#10333);
#7837=LINE('',#65224,#10334);
#7838=LINE('',#65228,#10335);
#7839=LINE('',#65232,#10336);
#7840=LINE('',#65246,#10337);
#7841=LINE('',#65247,#10338);
#7842=LINE('',#65249,#10339);
#7843=LINE('',#65250,#10340);
#7844=LINE('',#65262,#10341);
#7845=LINE('',#65272,#10342);
#7846=LINE('',#65273,#10343);
#7847=LINE('',#65276,#10344);
#7848=LINE('',#65278,#10345);
#7849=LINE('',#65279,#10346);
#7850=LINE('',#65323,#10347);
#7851=LINE('',#65325,#10348);
#7852=LINE('',#65326,#10349);
#7853=LINE('',#65327,#10350);
#7854=LINE('',#65329,#10351);
#7855=LINE('',#65330,#10352);
#7856=LINE('',#65335,#10353);
#7857=LINE('',#65339,#10354);
#7858=LINE('',#65341,#10355);
#7859=LINE('',#65342,#10356);
#7860=LINE('',#65345,#10357);
#7861=LINE('',#65347,#10358);
#7862=LINE('',#65348,#10359);
#7863=LINE('',#65351,#10360);
#7864=LINE('',#65353,#10361);
#7865=LINE('',#65354,#10362);
#7866=LINE('',#65357,#10363);
#7867=LINE('',#65359,#10364);
#7868=LINE('',#65361,#10365);
#7869=LINE('',#65362,#10366);
#7870=LINE('',#65366,#10367);
#7871=LINE('',#65368,#10368);
#7872=LINE('',#65370,#10369);
#7873=LINE('',#65371,#10370);
#7874=LINE('',#65389,#10371);
#7875=LINE('',#65391,#10372);
#7876=LINE('',#65394,#10373);
#7877=LINE('',#65396,#10374);
#7878=LINE('',#65399,#10375);
#7879=LINE('',#65400,#10376);
#7880=LINE('',#65403,#10377);
#7881=LINE('',#65405,#10378);
#7882=LINE('',#65406,#10379);
#7883=LINE('',#65448,#10380);
#7884=LINE('',#65450,#10381);
#7885=LINE('',#65460,#10382);
#7886=LINE('',#65462,#10383);
#7887=LINE('',#65463,#10384);
#7888=LINE('',#65466,#10385);
#7889=LINE('',#65468,#10386);
#7890=LINE('',#65469,#10387);
#7891=LINE('',#65472,#10388);
#7892=LINE('',#65473,#10389);
#7893=LINE('',#65476,#10390);
#7894=LINE('',#65477,#10391);
#7895=LINE('',#65488,#10392);
#7896=LINE('',#65499,#10393);
#7897=LINE('',#65502,#10394);
#7898=LINE('',#65503,#10395);
#7899=LINE('',#65514,#10396);
#7900=LINE('',#65525,#10397);
#7901=LINE('',#65527,#10398);
#7902=LINE('',#65531,#10399);
#7903=LINE('',#65533,#10400);
#7904=LINE('',#65534,#10401);
#7905=LINE('',#65537,#10402);
#7906=LINE('',#65538,#10403);
#7907=LINE('',#65541,#10404);
#7908=LINE('',#65542,#10405);
#7909=LINE('',#65545,#10406);
#7910=LINE('',#65546,#10407);
#7911=LINE('',#65549,#10408);
#7912=LINE('',#65550,#10409);
#7913=LINE('',#65553,#10410);
#7914=LINE('',#65554,#10411);
#7915=LINE('',#65557,#10412);
#7916=LINE('',#65558,#10413);
#7917=LINE('',#65561,#10414);
#7918=LINE('',#65562,#10415);
#7919=LINE('',#65565,#10416);
#7920=LINE('',#65566,#10417);
#7921=LINE('',#65568,#10418);
#7922=LINE('',#65582,#10419);
#7923=LINE('',#65587,#10420);
#7924=LINE('',#65602,#10421);
#7925=LINE('',#65617,#10422);
#7926=LINE('',#65632,#10423);
#7927=LINE('',#65647,#10424);
#7928=LINE('',#65662,#10425);
#7929=LINE('',#65677,#10426);
#7930=LINE('',#65697,#10427);
#7931=LINE('',#65702,#10428);
#7932=LINE('',#65713,#10429);
#7933=LINE('',#65724,#10430);
#7934=LINE('',#65735,#10431);
#7935=LINE('',#65746,#10432);
#7936=LINE('',#65757,#10433);
#7937=LINE('',#65768,#10434);
#7938=LINE('',#65779,#10435);
#7939=LINE('',#65790,#10436);
#7940=LINE('',#65803,#10437);
#7941=LINE('',#65805,#10438);
#7942=LINE('',#65806,#10439);
#7943=LINE('',#65809,#10440);
#7944=LINE('',#65810,#10441);
#7945=LINE('',#65813,#10442);
#7946=LINE('',#65814,#10443);
#7947=LINE('',#65816,#10444);
#7948=LINE('',#65822,#10445);
#7949=LINE('',#65827,#10446);
#7950=LINE('',#65829,#10447);
#7951=LINE('',#65831,#10448);
#7952=LINE('',#65833,#10449);
#7953=LINE('',#65835,#10450);
#7954=LINE('',#65840,#10451);
#7955=LINE('',#65841,#10452);
#7956=LINE('',#65843,#10453);
#7957=LINE('',#65845,#10454);
#7958=LINE('',#65847,#10455);
#7959=LINE('',#65850,#10456);
#7960=LINE('',#65851,#10457);
#7961=LINE('',#65853,#10458);
#7962=LINE('',#65854,#10459);
#7963=LINE('',#65860,#10460);
#7964=LINE('',#65867,#10461);
#7965=LINE('',#65873,#10462);
#7966=LINE('',#65877,#10463);
#7967=LINE('',#65881,#10464);
#7968=LINE('',#65884,#10465);
#7969=LINE('',#65889,#10466);
#7970=LINE('',#65891,#10467);
#7971=LINE('',#65895,#10468);
#7972=LINE('',#65897,#10469);
#7973=LINE('',#65899,#10470);
#7974=LINE('',#65901,#10471);
#7975=LINE('',#65905,#10472);
#7976=LINE('',#65907,#10473);
#7977=LINE('',#65910,#10474);
#7978=LINE('',#65924,#10475);
#7979=LINE('',#65926,#10476);
#7980=LINE('',#65930,#10477);
#7981=LINE('',#65932,#10478);
#7982=LINE('',#65936,#10479);
#7983=LINE('',#65938,#10480);
#7984=LINE('',#65939,#10481);
#7985=LINE('',#65942,#10482);
#7986=LINE('',#65946,#10483);
#7987=LINE('',#65947,#10484);
#7988=LINE('',#65952,#10485);
#7989=LINE('',#65956,#10486);
#7990=LINE('',#65957,#10487);
#7991=LINE('',#65962,#10488);
#7992=LINE('',#65966,#10489);
#7993=LINE('',#65967,#10490);
#7994=LINE('',#65970,#10491);
#7995=LINE('',#65974,#10492);
#7996=LINE('',#65975,#10493);
#7997=LINE('',#65978,#10494);
#7998=LINE('',#65981,#10495);
#7999=LINE('',#65985,#10496);
#8000=LINE('',#65986,#10497);
#8001=LINE('',#65988,#10498);
#8002=LINE('',#65991,#10499);
#8003=LINE('',#65993,#10500);
#8004=LINE('',#65996,#10501);
#8005=LINE('',#65998,#10502);
#10110=VECTOR('',#33666,1.);
#10111=VECTOR('',#33669,1.);
#10112=VECTOR('',#33674,1.);
#10113=VECTOR('',#33677,1.);
#10114=VECTOR('',#33690,1.);
#10115=VECTOR('',#33691,1.);
#10116=VECTOR('',#33692,1.);
#10117=VECTOR('',#33695,1.);
#10118=VECTOR('',#33696,1.);
#10119=VECTOR('',#33697,1.);
#10120=VECTOR('',#33700,1.);
#10121=VECTOR('',#33705,6.255);
#10122=VECTOR('',#33706,6.255);
#10123=VECTOR('',#33713,1.);
#10124=VECTOR('',#33716,1.);
#10125=VECTOR('',#33721,1.);
#10126=VECTOR('',#33722,1.);
#10127=VECTOR('',#33723,1.);
#10128=VECTOR('',#33724,1.);
#10129=VECTOR('',#33725,1.);
#10130=VECTOR('',#33728,1.);
#10131=VECTOR('',#33729,1.);
#10132=VECTOR('',#33730,1.);
#10133=VECTOR('',#33733,1.);
#10134=VECTOR('',#33734,1.);
#10135=VECTOR('',#33739,1.);
#10136=VECTOR('',#33744,1.);
#10137=VECTOR('',#33747,1.);
#10138=VECTOR('',#33748,1.);
#10139=VECTOR('',#33749,1.);
#10140=VECTOR('',#33752,1.);
#10141=VECTOR('',#33753,1.);
#10142=VECTOR('',#33754,1.);
#10143=VECTOR('',#33755,1.);
#10144=VECTOR('',#33756,1.);
#10145=VECTOR('',#33761,1.);
#10146=VECTOR('',#33774,1.);
#10147=VECTOR('',#33785,1.);
#10148=VECTOR('',#33788,1.);
#10149=VECTOR('',#33793,1.);
#10150=VECTOR('',#33794,1.);
#10151=VECTOR('',#33797,1.);
#10152=VECTOR('',#33802,1.);
#10153=VECTOR('',#33803,1.);
#10154=VECTOR('',#33808,1.);
#10155=VECTOR('',#33821,1.);
#10156=VECTOR('',#33824,1.);
#10157=VECTOR('',#33825,1.);
#10158=VECTOR('',#33830,1.);
#10159=VECTOR('',#33831,1.);
#10160=VECTOR('',#33834,1.);
#10161=VECTOR('',#33839,1.);
#10162=VECTOR('',#33840,1.);
#10163=VECTOR('',#33843,1.);
#10164=VECTOR('',#33846,1.);
#10165=VECTOR('',#33849,1.);
#10166=VECTOR('',#33852,1.);
#10167=VECTOR('',#33865,1.);
#10168=VECTOR('',#33866,1.);
#10169=VECTOR('',#33867,1.);
#10170=VECTOR('',#33868,1.);
#10171=VECTOR('',#33869,1.);
#10172=VECTOR('',#33874,1.);
#10173=VECTOR('',#33877,1.);
#10174=VECTOR('',#33890,1.1);
#10175=VECTOR('',#33911,1.1);
#10176=VECTOR('',#33928,1.1);
#10177=VECTOR('',#33939,1.1);
#10178=VECTOR('',#33960,1.);
#10179=VECTOR('',#33961,1.);
#10180=VECTOR('',#33964,1.);
#10181=VECTOR('',#33965,1.);
#10182=VECTOR('',#33980,1.);
#10183=VECTOR('',#33981,1.);
#10184=VECTOR('',#33986,1.);
#10185=VECTOR('',#33989,1.);
#10186=VECTOR('',#33992,1.);
#10187=VECTOR('',#33993,1.);
#10188=VECTOR('',#33994,1.);
#10189=VECTOR('',#33995,1.);
#10190=VECTOR('',#33996,1.);
#10191=VECTOR('',#33999,1.);
#10192=VECTOR('',#34002,1.);
#10193=VECTOR('',#34005,1.);
#10194=VECTOR('',#34008,1.);
#10195=VECTOR('',#34011,1.);
#10196=VECTOR('',#34020,1.);
#10197=VECTOR('',#34023,1.);
#10198=VECTOR('',#34026,1.);
#10199=VECTOR('',#34029,1.);
#10200=VECTOR('',#34034,1.);
#10201=VECTOR('',#34035,1.);
#10202=VECTOR('',#34036,1.);
#10203=VECTOR('',#34047,1.);
#10204=VECTOR('',#34050,1.);
#10205=VECTOR('',#34053,1.);
#10206=VECTOR('',#34056,1.);
#10207=VECTOR('',#34059,1.);
#10208=VECTOR('',#34062,1.);
#10209=VECTOR('',#34067,1.);
#10210=VECTOR('',#34070,1.);
#10211=VECTOR('',#34073,1.);
#10212=VECTOR('',#34088,1.);
#10213=VECTOR('',#34089,1.);
#10214=VECTOR('',#34090,1.);
#10215=VECTOR('',#34093,1.);
#10216=VECTOR('',#34096,1.);
#10217=VECTOR('',#34099,1.);
#10218=VECTOR('',#34102,1.);
#10219=VECTOR('',#34105,1.);
#10220=VECTOR('',#34108,1.);
#10221=VECTOR('',#34109,1.);
#10222=VECTOR('',#34110,1.);
#10223=VECTOR('',#34125,1.);
#10224=VECTOR('',#34126,1.);
#10225=VECTOR('',#34127,1.);
#10226=VECTOR('',#34128,1.);
#10227=VECTOR('',#34129,1.);
#10228=VECTOR('',#34130,1.);
#10229=VECTOR('',#34131,1.);
#10230=VECTOR('',#34132,1.);
#10231=VECTOR('',#34143,0.804999999999993);
#10232=VECTOR('',#34156,0.804999999999993);
#10233=VECTOR('',#34169,0.804999999999993);
#10234=VECTOR('',#34180,1.);
#10235=VECTOR('',#34183,1.);
#10236=VECTOR('',#34186,1.);
#10237=VECTOR('',#34191,0.804999999999993);
#10238=VECTOR('',#34196,1.);
#10239=VECTOR('',#34201,1.);
#10240=VECTOR('',#34202,1.);
#10241=VECTOR('',#34203,1.);
#10242=VECTOR('',#34204,1.);
#10243=VECTOR('',#34205,1.);
#10244=VECTOR('',#34206,1.);
#10245=VECTOR('',#34207,1.);
#10246=VECTOR('',#34208,1.);
#10247=VECTOR('',#34225,2.);
#10248=VECTOR('',#34238,1.);
#10249=VECTOR('',#34241,1.);
#10250=VECTOR('',#34244,1.);
#10251=VECTOR('',#34245,1.);
#10252=VECTOR('',#34246,1.);
#10253=VECTOR('',#34253,1.);
#10254=VECTOR('',#34256,1.);
#10255=VECTOR('',#34259,1.);
#10256=VECTOR('',#34260,1.);
#10257=VECTOR('',#34273,1.);
#10258=VECTOR('',#34276,1.);
#10259=VECTOR('',#34279,1.);
#10260=VECTOR('',#34290,1.);
#10261=VECTOR('',#34291,1.);
#10262=VECTOR('',#34292,1.);
#10263=VECTOR('',#34293,1.);
#10264=VECTOR('',#34294,1.);
#10265=VECTOR('',#34295,1.);
#10266=VECTOR('',#34296,1.);
#10267=VECTOR('',#34297,1.);
#10268=VECTOR('',#34298,1.);
#10269=VECTOR('',#34299,1.);
#10270=VECTOR('',#34300,1.);
#10271=VECTOR('',#34329,1.);
#10272=VECTOR('',#34332,1.);
#10273=VECTOR('',#34333,1.);
#10274=VECTOR('',#34334,1.);
#10275=VECTOR('',#34339,1.);
#10276=VECTOR('',#34342,1.);
#10277=VECTOR('',#34343,1.);
#10278=VECTOR('',#34344,1.);
#10279=VECTOR('',#34351,1.);
#10280=VECTOR('',#34352,1.);
#10281=VECTOR('',#34353,1.);
#10282=VECTOR('',#34354,1.);
#10283=VECTOR('',#34355,1.);
#10284=VECTOR('',#34356,1.);
#10285=VECTOR('',#34359,1.);
#10286=VECTOR('',#34366,1.);
#10287=VECTOR('',#34377,1.);
#10288=VECTOR('',#34384,1.);
#10289=VECTOR('',#34385,1.);
#10290=VECTOR('',#34386,1.);
#10291=VECTOR('',#34389,1.);
#10292=VECTOR('',#34392,1.);
#10293=VECTOR('',#34395,1.);
#10294=VECTOR('',#34402,1.);
#10295=VECTOR('',#34405,1.);
#10296=VECTOR('',#34408,1.);
#10297=VECTOR('',#34411,1.);
#10298=VECTOR('',#34414,1.);
#10299=VECTOR('',#34419,1.);
#10300=VECTOR('',#34422,1.);
#10301=VECTOR('',#34423,1.);
#10302=VECTOR('',#34424,1.);
#10303=VECTOR('',#34425,1.);
#10304=VECTOR('',#34426,1.);
#10305=VECTOR('',#34429,1.);
#10306=VECTOR('',#34430,1.);
#10307=VECTOR('',#34431,1.);
#10308=VECTOR('',#34432,1.);
#10309=VECTOR('',#34433,1.);
#10310=VECTOR('',#34434,1.);
#10311=VECTOR('',#34435,1.);
#10312=VECTOR('',#34436,1.);
#10313=VECTOR('',#34437,1.);
#10314=VECTOR('',#34438,1.);
#10315=VECTOR('',#34439,1.);
#10316=VECTOR('',#34440,1.);
#10317=VECTOR('',#34441,1.);
#10318=VECTOR('',#34442,1.);
#10319=VECTOR('',#34443,1.);
#10320=VECTOR('',#34452,1.);
#10321=VECTOR('',#34455,1.);
#10322=VECTOR('',#34460,1.);
#10323=VECTOR('',#34467,1.);
#10324=VECTOR('',#34470,1.);
#10325=VECTOR('',#34473,1.);
#10326=VECTOR('',#34476,1.);
#10327=VECTOR('',#34479,1.);
#10328=VECTOR('',#34484,1.);
#10329=VECTOR('',#34487,1.);
#10330=VECTOR('',#34492,1.);
#10331=VECTOR('',#34501,1.);
#10332=VECTOR('',#34508,1.);
#10333=VECTOR('',#34511,1.);
#10334=VECTOR('',#34514,1.);
#10335=VECTOR('',#34519,1.);
#10336=VECTOR('',#34522,1.);
#10337=VECTOR('',#34545,1.);
#10338=VECTOR('',#34546,1.);
#10339=VECTOR('',#34549,1.);
#10340=VECTOR('',#34550,1.);
#10341=VECTOR('',#34561,1.);
#10342=VECTOR('',#34572,1.);
#10343=VECTOR('',#34573,1.);
#10344=VECTOR('',#34576,1.);
#10345=VECTOR('',#34577,1.);
#10346=VECTOR('',#34578,1.);
#10347=VECTOR('',#34589,1.);
#10348=VECTOR('',#34590,1.);
#10349=VECTOR('',#34591,1.);
#10350=VECTOR('',#34592,1.);
#10351=VECTOR('',#34595,1.);
#10352=VECTOR('',#34596,1.);
#10353=VECTOR('',#34601,1.);
#10354=VECTOR('',#34606,1.);
#10355=VECTOR('',#34607,1.);
#10356=VECTOR('',#34608,1.);
#10357=VECTOR('',#34611,1.);
#10358=VECTOR('',#34612,1.);
#10359=VECTOR('',#34613,1.);
#10360=VECTOR('',#34616,1.);
#10361=VECTOR('',#34617,1.);
#10362=VECTOR('',#34618,1.);
#10363=VECTOR('',#34621,1.);
#10364=VECTOR('',#34622,1.);
#10365=VECTOR('',#34623,1.);
#10366=VECTOR('',#34624,1.);
#10367=VECTOR('',#34627,1.);
#10368=VECTOR('',#34628,1.);
#10369=VECTOR('',#34629,1.);
#10370=VECTOR('',#34630,1.);
#10371=VECTOR('',#34645,1.);
#10372=VECTOR('',#34648,1.);
#10373=VECTOR('',#34653,1.);
#10374=VECTOR('',#34656,1.);
#10375=VECTOR('',#34659,1.);
#10376=VECTOR('',#34660,1.);
#10377=VECTOR('',#34663,1.);
#10378=VECTOR('',#34664,1.);
#10379=VECTOR('',#34665,1.);
#10380=VECTOR('',#34678,1.);
#10381=VECTOR('',#34681,1.);
#10382=VECTOR('',#34686,1.);
#10383=VECTOR('',#34689,1.);
#10384=VECTOR('',#34690,1.);
#10385=VECTOR('',#34693,1.);
#10386=VECTOR('',#34694,1.);
#10387=VECTOR('',#34695,1.);
#10388=VECTOR('',#34698,1.);
#10389=VECTOR('',#34699,1.);
#10390=VECTOR('',#34702,1.);
#10391=VECTOR('',#34703,1.);
#10392=VECTOR('',#34704,1.);
#10393=VECTOR('',#34705,1.);
#10394=VECTOR('',#34708,1.);
#10395=VECTOR('',#34709,1.);
#10396=VECTOR('',#34710,1.);
#10397=VECTOR('',#34711,1.);
#10398=VECTOR('',#34714,1.);
#10399=VECTOR('',#34719,1.);
#10400=VECTOR('',#34720,1.);
#10401=VECTOR('',#34721,1.);
#10402=VECTOR('',#34724,1.);
#10403=VECTOR('',#34725,1.);
#10404=VECTOR('',#34728,1.);
#10405=VECTOR('',#34729,1.);
#10406=VECTOR('',#34732,1.);
#10407=VECTOR('',#34733,1.);
#10408=VECTOR('',#34736,1.);
#10409=VECTOR('',#34737,1.);
#10410=VECTOR('',#34740,1.);
#10411=VECTOR('',#34741,1.);
#10412=VECTOR('',#34744,1.);
#10413=VECTOR('',#34745,1.);
#10414=VECTOR('',#34748,1.);
#10415=VECTOR('',#34749,1.);
#10416=VECTOR('',#34752,1.);
#10417=VECTOR('',#34753,1.);
#10418=VECTOR('',#34756,1.);
#10419=VECTOR('',#34759,1.);
#10420=VECTOR('',#34760,1.);
#10421=VECTOR('',#34761,1.);
#10422=VECTOR('',#34762,1.);
#10423=VECTOR('',#34763,1.);
#10424=VECTOR('',#34764,1.);
#10425=VECTOR('',#34765,1.);
#10426=VECTOR('',#34766,1.);
#10427=VECTOR('',#34767,1.);
#10428=VECTOR('',#34768,1.);
#10429=VECTOR('',#34769,1.);
#10430=VECTOR('',#34770,1.);
#10431=VECTOR('',#34771,1.);
#10432=VECTOR('',#34772,1.);
#10433=VECTOR('',#34773,1.);
#10434=VECTOR('',#34774,1.);
#10435=VECTOR('',#34775,1.);
#10436=VECTOR('',#34776,1.);
#10437=VECTOR('',#34781,1.);
#10438=VECTOR('',#34782,1.);
#10439=VECTOR('',#34783,1.);
#10440=VECTOR('',#34786,1.);
#10441=VECTOR('',#34787,1.);
#10442=VECTOR('',#34790,1.);
#10443=VECTOR('',#34791,1.);
#10444=VECTOR('',#34794,1.);
#10445=VECTOR('',#34803,2.25);
#10446=VECTOR('',#34810,2.25);
#10447=VECTOR('',#34813,2.25);
#10448=VECTOR('',#34816,2.25);
#10449=VECTOR('',#34819,1.);
#10450=VECTOR('',#34822,1.);
#10451=VECTOR('',#34829,1.);
#10452=VECTOR('',#34830,1.);
#10453=VECTOR('',#34833,1.);
#10454=VECTOR('',#34836,1.);
#10455=VECTOR('',#34839,1.);
#10456=VECTOR('',#34842,1.);
#10457=VECTOR('',#34843,1.);
#10458=VECTOR('',#34846,1.);
#10459=VECTOR('',#34847,1.);
#10460=VECTOR('',#34856,6.355);
#10461=VECTOR('',#34865,6.355);
#10462=VECTOR('',#34872,10.15);
#10463=VECTOR('',#34877,10.);
#10464=VECTOR('',#34884,9.85);
#10465=VECTOR('',#34887,10.15);
#10466=VECTOR('',#34894,10.);
#10467=VECTOR('',#34897,9.85);
#10468=VECTOR('',#34902,1.);
#10469=VECTOR('',#34905,1.);
#10470=VECTOR('',#34908,1.);
#10471=VECTOR('',#34911,1.);
#10472=VECTOR('',#34918,1.);
#10473=VECTOR('',#34921,1.);
#10474=VECTOR('',#34926,1.);
#10475=VECTOR('',#34939,1.);
#10476=VECTOR('',#34942,1.);
#10477=VECTOR('',#34949,1.);
#10478=VECTOR('',#34952,1.);
#10479=VECTOR('',#34957,1.);
#10480=VECTOR('',#34958,1.);
#10481=VECTOR('',#34959,1.);
#10482=VECTOR('',#34962,1.);
#10483=VECTOR('',#34967,1.);
#10484=VECTOR('',#34968,1.);
#10485=VECTOR('',#34975,1.);
#10486=VECTOR('',#34980,1.);
#10487=VECTOR('',#34981,1.);
#10488=VECTOR('',#34988,1.);
#10489=VECTOR('',#34993,1.);
#10490=VECTOR('',#34994,1.);
#10491=VECTOR('',#34997,1.);
#10492=VECTOR('',#35002,1.);
#10493=VECTOR('',#35003,1.);
#10494=VECTOR('',#35008,1.);
#10495=VECTOR('',#35011,1.);
#10496=VECTOR('',#35016,1.);
#10497=VECTOR('',#35017,1.);
#10498=VECTOR('',#35020,1.);
#10499=VECTOR('',#35025,1.);
#10500=VECTOR('',#35028,1.);
#10501=VECTOR('',#35033,1.);
#10502=VECTOR('',#35036,1.);
#10923=CIRCLE('',#28398,6.255);
#10924=CIRCLE('',#28399,6.255);
#10925=CIRCLE('',#28400,6.555);
#10926=CIRCLE('',#28402,0.3);
#10927=CIRCLE('',#28403,0.3);
#10928=CIRCLE('',#28405,0.3);
#10929=CIRCLE('',#28406,0.3);
#10930=CIRCLE('',#28408,6.255);
#10931=CIRCLE('',#28409,6.255);
#10932=CIRCLE('',#28410,6.555);
#10933=CIRCLE('',#28413,0.3);
#10934=CIRCLE('',#28415,6.255);
#10935=CIRCLE('',#28416,6.255);
#10936=CIRCLE('',#28432,0.300000000000001);
#10937=CIRCLE('',#28434,0.3);
#10938=CIRCLE('',#28435,0.3);
#10939=CIRCLE('',#28436,0.3);
#10940=CIRCLE('',#28440,0.300000000000001);
#10941=CIRCLE('',#28441,0.299999999999999);
#10942=CIRCLE('',#28451,0.3);
#10943=CIRCLE('',#28453,0.3);
#10944=CIRCLE('',#28454,4.);
#10945=CIRCLE('',#28455,4.3);
#10946=CIRCLE('',#28464,1.3);
#10947=CIRCLE('',#28465,1.3);
#10948=CIRCLE('',#28466,1.3);
#10949=CIRCLE('',#28467,1.3);
#10950=CIRCLE('',#28468,1.4);
#10951=CIRCLE('',#28469,1.4);
#10952=CIRCLE('',#28470,1.4);
#10953=CIRCLE('',#28471,1.4);
#10954=CIRCLE('',#28473,2.3);
#10955=CIRCLE('',#28477,1.1);
#10956=CIRCLE('',#28478,0.3);
#10957=CIRCLE('',#28479,1.4);
#10958=CIRCLE('',#28481,1.1);
#10959=CIRCLE('',#28483,2.25);
#10960=CIRCLE('',#28485,0.3);
#10961=CIRCLE('',#28487,1.1);
#10962=CIRCLE('',#28488,0.3);
#10963=CIRCLE('',#28489,1.4);
#10964=CIRCLE('',#28491,1.1);
#10965=CIRCLE('',#28493,2.25);
#10966=CIRCLE('',#28495,0.3);
#10967=CIRCLE('',#28497,0.3);
#10968=CIRCLE('',#28498,1.1);
#10969=CIRCLE('',#28500,1.1);
#10970=CIRCLE('',#28502,0.3);
#10971=CIRCLE('',#28503,1.1);
#10972=CIRCLE('',#28505,1.1);
#10973=CIRCLE('',#28507,0.300000000000001);
#10974=CIRCLE('',#28508,0.300000000000004);
#10975=CIRCLE('',#28509,0.300000000000001);
#10976=CIRCLE('',#28511,0.299999999999998);
#10977=CIRCLE('',#28512,0.299999999999997);
#10978=CIRCLE('',#28513,0.300000000000001);
#10979=CIRCLE('',#28517,30.6296013460341);
#10980=CIRCLE('',#28518,30.9296013460341);
#10981=CIRCLE('',#28520,30.9296013460341);
#10982=CIRCLE('',#28521,30.6296013460341);
#10983=CIRCLE('',#28524,8.);
#10984=CIRCLE('',#28525,7.99950242947666);
#10985=CIRCLE('',#28528,0.299999999999997);
#10986=CIRCLE('',#28530,0.3);
#10987=CIRCLE('',#28531,0.299999999999998);
#10988=CIRCLE('',#28533,0.3);
#10989=CIRCLE('',#28535,31.5);
#10990=CIRCLE('',#28536,31.5);
#10991=CIRCLE('',#28537,31.5);
#10992=CIRCLE('',#28538,31.5);
#10993=CIRCLE('',#28540,32.7);
#10994=CIRCLE('',#28542,33.);
#10995=CIRCLE('',#28543,0.299999999999997);
#10996=CIRCLE('',#28545,33.);
#10997=CIRCLE('',#28546,33.);
#10998=CIRCLE('',#28547,33.);
#10999=CIRCLE('',#28548,33.);
#11000=CIRCLE('',#28549,33.);
#11001=CIRCLE('',#28551,0.299999999999997);
#11002=CIRCLE('',#28552,0.3);
#11003=CIRCLE('',#28554,0.300000000000002);
#11004=CIRCLE('',#28556,0.3);
#11005=CIRCLE('',#28558,32.7);
#11006=CIRCLE('',#28559,0.299999999999997);
#11007=CIRCLE('',#28561,31.5);
#11008=CIRCLE('',#28563,31.5);
#11009=CIRCLE('',#28564,31.5);
#11010=CIRCLE('',#28565,31.5);
#11011=CIRCLE('',#28569,1.10499999999999);
#11012=CIRCLE('',#28570,0.3);
#11013=CIRCLE('',#28571,0.804999999999993);
#11014=CIRCLE('',#28572,0.804999999999993);
#11015=CIRCLE('',#28574,1.10499999999999);
#11016=CIRCLE('',#28575,1.10499999999999);
#11017=CIRCLE('',#28576,1.10499999999999);
#11018=CIRCLE('',#28577,1.10499999999999);
#11019=CIRCLE('',#28579,0.804999999999993);
#11020=CIRCLE('',#28581,0.3);
#11021=CIRCLE('',#28582,0.804999999999993);
#11022=CIRCLE('',#28583,0.804999999999993);
#11023=CIRCLE('',#28585,0.804999999999993);
#11024=CIRCLE('',#28587,0.3);
#11025=CIRCLE('',#28588,0.804999999999993);
#11026=CIRCLE('',#28589,0.804999999999993);
#11027=CIRCLE('',#28591,0.804999999999993);
#11028=CIRCLE('',#28593,0.3);
#11029=CIRCLE('',#28594,0.804999999999993);
#11030=CIRCLE('',#28595,0.804999999999993);
#11031=CIRCLE('',#28600,0.804999999999993);
#11032=CIRCLE('',#28602,0.3);
#11033=CIRCLE('',#28603,0.3);
#11034=CIRCLE('',#28605,1.10499999999999);
#11035=CIRCLE('',#28606,1.10499999999999);
#11036=CIRCLE('',#28607,1.10499999999999);
#11037=CIRCLE('',#28608,1.10499999999999);
#11038=CIRCLE('',#28610,0.3);
#11039=CIRCLE('',#28611,2.);
#11040=CIRCLE('',#28613,2.);
#11041=CIRCLE('',#28614,2.);
#11042=CIRCLE('',#28616,30.9296013460341);
#11043=CIRCLE('',#28617,30.6296013460341);
#11044=CIRCLE('',#28619,30.6296013460341);
#11045=CIRCLE('',#28622,30.9296013460341);
#11046=CIRCLE('',#28624,7.99950242947665);
#11047=CIRCLE('',#28627,2.3);
#11048=CIRCLE('',#28628,0.3);
#11049=CIRCLE('',#28630,4.);
#11050=CIRCLE('',#28631,1.2);
#11051=CIRCLE('',#28632,1.2);
#11052=CIRCLE('',#28633,1.2);
#11053=CIRCLE('',#28634,1.2);
#11054=CIRCLE('',#28635,2.25);
#11055=CIRCLE('',#28636,2.25);
#11056=CIRCLE('',#28637,2.25);
#11057=CIRCLE('',#28638,2.25);
#11058=CIRCLE('',#28640,0.3);
#11059=CIRCLE('',#28644,0.3);
#11060=CIRCLE('',#28646,0.3);
#11061=CIRCLE('',#28648,0.3);
#11062=CIRCLE('',#28650,0.3);
#11063=CIRCLE('',#28655,0.3);
#11064=CIRCLE('',#28658,2.8);
#11065=CIRCLE('',#28662,32.7);
#11066=CIRCLE('',#28664,4.00009261333671);
#11067=CIRCLE('',#28666,32.7);
#11068=CIRCLE('',#28668,4.00009261333671);
#11069=CIRCLE('',#28670,0.3);
#11070=CIRCLE('',#28675,3.70000000000001);
#11071=CIRCLE('',#28677,3.70000000000001);
#11072=CIRCLE('',#28679,3.70000000000002);
#11073=CIRCLE('',#28680,8.3);
#11074=CIRCLE('',#28681,8.3);
#11075=CIRCLE('',#28682,2.8);
#11076=CIRCLE('',#28683,11.7);
#11077=CIRCLE('',#28684,5.29999999999999);
#11078=CIRCLE('',#28685,10.3);
#11079=CIRCLE('',#28687,4.00009261333671);
#11080=CIRCLE('',#28692,12.);
#11081=CIRCLE('',#28693,12.);
#11082=CIRCLE('',#28695,11.7);
#11083=CIRCLE('',#28697,8.3);
#11084=CIRCLE('',#28698,8.3);
#11085=CIRCLE('',#28699,3.70000000000002);
#11086=CIRCLE('',#28700,3.70000000000001);
#11087=CIRCLE('',#28701,3.70000000000001);
#11088=CIRCLE('',#28702,5.29999999999999);
#11089=CIRCLE('',#28703,10.3);
#11090=CIRCLE('',#28706,4.00009261333671);
#11091=CIRCLE('',#28713,2.825);
#11092=CIRCLE('',#28714,2.5);
#11093=CIRCLE('',#28716,2.5);
#11094=CIRCLE('',#28717,2.825);
#11095=CIRCLE('',#28719,8.);
#11096=CIRCLE('',#28721,8.);
#11097=CIRCLE('',#28725,8.);
#11098=CIRCLE('',#28742,7.99950242947665);
#11099=CIRCLE('',#28747,12.);
#11100=CIRCLE('',#28748,12.);
#11101=CIRCLE('',#28755,4.00009261333671);
#11102=CIRCLE('',#28757,5.00011576667089);
#11103=CIRCLE('',#28759,4.00009261333671);
#11104=CIRCLE('',#28761,5.00011576667089);
#11105=CIRCLE('',#28771,7.99950242947666);
#11106=CIRCLE('',#28801,2.25);
#11107=CIRCLE('',#28804,2.25);
#11108=CIRCLE('',#28821,6.455);
#11109=CIRCLE('',#28823,9.7);
#11110=CIRCLE('',#28825,6.455);
#11111=CIRCLE('',#28827,9.7);
#11112=CIRCLE('',#28829,10.);
#11113=CIRCLE('',#28831,10.);
#11114=CIRCLE('',#28835,10.);
#11115=CIRCLE('',#28837,10.);
#11116=CIRCLE('',#28844,5.);
#11117=CIRCLE('',#28852,5.);
#11118=CIRCLE('',#28864,1.5);
#11119=CIRCLE('',#28867,1.5);
#11120=CIRCLE('',#28869,1.5);
#11121=CIRCLE('',#28872,1.5);
#11122=CIRCLE('',#28874,1.5);
#11123=CIRCLE('',#28877,1.5);
#11124=CIRCLE('',#28882,1.5);
#11125=CIRCLE('',#28885,1.5);
#12931=VERTEX_POINT('',#63932);
#12932=VERTEX_POINT('',#63933);
#12933=VERTEX_POINT('',#63935);
#12934=VERTEX_POINT('',#63937);
#12935=VERTEX_POINT('',#63950);
#12936=VERTEX_POINT('',#63967);
#12937=VERTEX_POINT('',#63968);
#12938=VERTEX_POINT('',#63971);
#12939=VERTEX_POINT('',#63973);
#12940=VERTEX_POINT('',#63988);
#12941=VERTEX_POINT('',#63990);
#12942=VERTEX_POINT('',#63992);
#12943=VERTEX_POINT('',#63994);
#12944=VERTEX_POINT('',#64011);
#12945=VERTEX_POINT('',#64016);
#12946=VERTEX_POINT('',#64018);
#12947=VERTEX_POINT('',#64022);
#12948=VERTEX_POINT('',#64024);
#12949=VERTEX_POINT('',#64026);
#12950=VERTEX_POINT('',#64028);
#12951=VERTEX_POINT('',#64032);
#12952=VERTEX_POINT('',#64035);
#12953=VERTEX_POINT('',#64039);
#12954=VERTEX_POINT('',#64040);
#12955=VERTEX_POINT('',#64042);
#12956=VERTEX_POINT('',#64044);
#12957=VERTEX_POINT('',#64046);
#12958=VERTEX_POINT('',#64050);
#12959=VERTEX_POINT('',#64052);
#12960=VERTEX_POINT('',#64054);
#12961=VERTEX_POINT('',#64056);
#12962=VERTEX_POINT('',#64060);
#12963=VERTEX_POINT('',#64062);
#12964=VERTEX_POINT('',#64066);
#12965=VERTEX_POINT('',#64070);
#12966=VERTEX_POINT('',#64071);
#12967=VERTEX_POINT('',#64073);
#12968=VERTEX_POINT('',#64075);
#12969=VERTEX_POINT('',#64077);
#12970=VERTEX_POINT('',#64081);
#12971=VERTEX_POINT('',#64083);
#12972=VERTEX_POINT('',#64087);
#12973=VERTEX_POINT('',#64089);
#12974=VERTEX_POINT('',#64091);
#12975=VERTEX_POINT('',#64093);
#12976=VERTEX_POINT('',#64097);
#12977=VERTEX_POINT('',#64099);
#12978=VERTEX_POINT('',#64103);
#12979=VERTEX_POINT('',#64105);
#12980=VERTEX_POINT('',#64109);
#12981=VERTEX_POINT('',#64113);
#12982=VERTEX_POINT('',#64117);
#12983=VERTEX_POINT('',#64118);
#12984=VERTEX_POINT('',#64120);
#12985=VERTEX_POINT('',#64122);
#12986=VERTEX_POINT('',#64129);
#12987=VERTEX_POINT('',#64133);
#12988=VERTEX_POINT('',#64135);
#12989=VERTEX_POINT('',#64139);
#12990=VERTEX_POINT('',#64143);
#12991=VERTEX_POINT('',#64150);
#12992=VERTEX_POINT('',#64152);
#12993=VERTEX_POINT('',#64159);
#12994=VERTEX_POINT('',#64163);
#12995=VERTEX_POINT('',#64167);
#12996=VERTEX_POINT('',#64169);
#12997=VERTEX_POINT('',#64171);
#12998=VERTEX_POINT('',#64173);
#12999=VERTEX_POINT('',#64175);
#13000=VERTEX_POINT('',#64177);
#13001=VERTEX_POINT('',#64179);
#13002=VERTEX_POINT('',#64182);
#13003=VERTEX_POINT('',#64184);
#13004=VERTEX_POINT('',#64186);
#13005=VERTEX_POINT('',#64188);
#13006=VERTEX_POINT('',#64191);
#13007=VERTEX_POINT('',#64193);
#13008=VERTEX_POINT('',#64195);
#13009=VERTEX_POINT('',#64197);
#13010=VERTEX_POINT('',#64200);
#13011=VERTEX_POINT('',#64207);
#13012=VERTEX_POINT('',#64209);
#13013=VERTEX_POINT('',#64213);
#13014=VERTEX_POINT('',#64217);
#13015=VERTEX_POINT('',#64222);
#13016=VERTEX_POINT('',#64224);
#13017=VERTEX_POINT('',#64228);
#13018=VERTEX_POINT('',#64232);
#13019=VERTEX_POINT('',#64237);
#13020=VERTEX_POINT('',#64241);
#13021=VERTEX_POINT('',#64245);
#13022=VERTEX_POINT('',#64249);
#13023=VERTEX_POINT('',#64253);
#13024=VERTEX_POINT('',#64254);
#13025=VERTEX_POINT('',#64256);
#13026=VERTEX_POINT('',#64260);
#13027=VERTEX_POINT('',#64261);
#13028=VERTEX_POINT('',#64263);
#13029=VERTEX_POINT('',#64270);
#13030=VERTEX_POINT('',#64271);
#13031=VERTEX_POINT('',#64285);
#13032=VERTEX_POINT('',#64286);
#13033=VERTEX_POINT('',#64304);
#13034=VERTEX_POINT('',#64305);
#13035=VERTEX_POINT('',#64323);
#13036=VERTEX_POINT('',#64324);
#13037=VERTEX_POINT('',#64338);
#13038=VERTEX_POINT('',#64340);
#13039=VERTEX_POINT('',#64342);
#13040=VERTEX_POINT('',#64346);
#13041=VERTEX_POINT('',#64348);
#13042=VERTEX_POINT('',#64350);
#13043=VERTEX_POINT('',#64352);
#13044=VERTEX_POINT('',#64356);
#13045=VERTEX_POINT('',#64357);
#13046=VERTEX_POINT('',#64368);
#13047=VERTEX_POINT('',#64370);
#13048=VERTEX_POINT('',#64374);
#13049=VERTEX_POINT('',#64375);
#13050=VERTEX_POINT('',#64382);
#13051=VERTEX_POINT('',#64384);
#13052=VERTEX_POINT('',#64386);
#13053=VERTEX_POINT('',#64393);
#13054=VERTEX_POINT('',#64395);
#13055=VERTEX_POINT('',#64397);
#13056=VERTEX_POINT('',#64399);
#13057=VERTEX_POINT('',#64406);
#13058=VERTEX_POINT('',#64408);
#13059=VERTEX_POINT('',#64410);
#13060=VERTEX_POINT('',#64412);
#13061=VERTEX_POINT('',#64419);
#13062=VERTEX_POINT('',#64423);
#13063=VERTEX_POINT('',#64425);
#13064=VERTEX_POINT('',#64427);
#13065=VERTEX_POINT('',#64431);
#13066=VERTEX_POINT('',#64435);
#13067=VERTEX_POINT('',#64437);
#13068=VERTEX_POINT('',#64439);
#13069=VERTEX_POINT('',#64441);
#13070=VERTEX_POINT('',#64443);
#13071=VERTEX_POINT('',#64446);
#13072=VERTEX_POINT('',#64447);
#13073=VERTEX_POINT('',#64449);
#13074=VERTEX_POINT('',#64451);
#13075=VERTEX_POINT('',#64455);
#13076=VERTEX_POINT('',#64456);
#13077=VERTEX_POINT('',#64463);
#13078=VERTEX_POINT('',#64466);
#13079=VERTEX_POINT('',#64470);
#13080=VERTEX_POINT('',#64471);
#13081=VERTEX_POINT('',#64482);
#13082=VERTEX_POINT('',#64489);
#13083=VERTEX_POINT('',#64493);
#13084=VERTEX_POINT('',#64495);
#13085=VERTEX_POINT('',#64497);
#13086=VERTEX_POINT('',#64501);
#13087=VERTEX_POINT('',#64503);
#13088=VERTEX_POINT('',#64505);
#13089=VERTEX_POINT('',#64512);
#13090=VERTEX_POINT('',#64514);
#13091=VERTEX_POINT('',#64516);
#13092=VERTEX_POINT('',#64518);
#13093=VERTEX_POINT('',#64525);
#13094=VERTEX_POINT('',#64529);
#13095=VERTEX_POINT('',#64540);
#13096=VERTEX_POINT('',#64553);
#13097=VERTEX_POINT('',#64560);
#13098=VERTEX_POINT('',#64562);
#13099=VERTEX_POINT('',#64564);
#13100=VERTEX_POINT('',#64573);
#13101=VERTEX_POINT('',#64575);
#13102=VERTEX_POINT('',#64577);
#13103=VERTEX_POINT('',#64581);
#13104=VERTEX_POINT('',#64582);
#13105=VERTEX_POINT('',#64584);
#13106=VERTEX_POINT('',#64586);
#13107=VERTEX_POINT('',#64588);
#13108=VERTEX_POINT('',#64591);
#13109=VERTEX_POINT('',#64593);
#13110=VERTEX_POINT('',#64595);
#13111=VERTEX_POINT('',#64597);
#13112=VERTEX_POINT('',#64600);
#13113=VERTEX_POINT('',#64602);
#13114=VERTEX_POINT('',#64605);
#13115=VERTEX_POINT('',#64609);
#13116=VERTEX_POINT('',#64611);
#13117=VERTEX_POINT('',#64615);
#13118=VERTEX_POINT('',#64619);
#13119=VERTEX_POINT('',#64621);
#13120=VERTEX_POINT('',#64625);
#13121=VERTEX_POINT('',#64639);
#13122=VERTEX_POINT('',#64641);
#13123=VERTEX_POINT('',#64645);
#13124=VERTEX_POINT('',#64664);
#13125=VERTEX_POINT('',#64666);
#13126=VERTEX_POINT('',#64668);
#13127=VERTEX_POINT('',#64670);
#13128=VERTEX_POINT('',#64672);
#13129=VERTEX_POINT('',#64693);
#13130=VERTEX_POINT('',#64697);
#13131=VERTEX_POINT('',#64712);
#13132=VERTEX_POINT('',#64727);
#13133=VERTEX_POINT('',#64729);
#13134=VERTEX_POINT('',#64733);
#13135=VERTEX_POINT('',#64735);
#13136=VERTEX_POINT('',#64737);
#13137=VERTEX_POINT('',#64739);
#13138=VERTEX_POINT('',#64742);
#13139=VERTEX_POINT('',#64744);
#13140=VERTEX_POINT('',#64747);
#13141=VERTEX_POINT('',#64749);
#13142=VERTEX_POINT('',#64751);
#13143=VERTEX_POINT('',#64753);
#13144=VERTEX_POINT('',#64756);
#13145=VERTEX_POINT('',#64760);
#13146=VERTEX_POINT('',#64762);
#13147=VERTEX_POINT('',#64766);
#13148=VERTEX_POINT('',#64767);
#13149=VERTEX_POINT('',#64782);
#13150=VERTEX_POINT('',#64784);
#13151=VERTEX_POINT('',#64801);
#13152=VERTEX_POINT('',#64803);
#13153=VERTEX_POINT('',#64807);
#13154=VERTEX_POINT('',#64809);
#13155=VERTEX_POINT('',#64813);
#13156=VERTEX_POINT('',#64828);
#13157=VERTEX_POINT('',#64845);
#13158=VERTEX_POINT('',#64847);
#13159=VERTEX_POINT('',#64851);
#13160=VERTEX_POINT('',#64855);
#13161=VERTEX_POINT('',#64860);
#13162=VERTEX_POINT('',#64862);
#13163=VERTEX_POINT('',#64864);
#13164=VERTEX_POINT('',#64866);
#13165=VERTEX_POINT('',#64868);
#13166=VERTEX_POINT('',#64870);
#13167=VERTEX_POINT('',#64873);
#13168=VERTEX_POINT('',#64875);
#13169=VERTEX_POINT('',#64877);
#13170=VERTEX_POINT('',#64879);
#13171=VERTEX_POINT('',#64881);
#13172=VERTEX_POINT('',#64882);
#13173=VERTEX_POINT('',#64884);
#13174=VERTEX_POINT('',#64886);
#13175=VERTEX_POINT('',#64890);
#13176=VERTEX_POINT('',#64892);
#13177=VERTEX_POINT('',#64894);
#13178=VERTEX_POINT('',#64896);
#13179=VERTEX_POINT('',#64901);
#13180=VERTEX_POINT('',#64914);
#13181=VERTEX_POINT('',#64915);
#13182=VERTEX_POINT('',#64917);
#13183=VERTEX_POINT('',#64919);
#13184=VERTEX_POINT('',#64921);
#13185=VERTEX_POINT('',#64923);
#13186=VERTEX_POINT('',#64930);
#13187=VERTEX_POINT('',#64932);
#13188=VERTEX_POINT('',#64944);
#13189=VERTEX_POINT('',#64946);
#13190=VERTEX_POINT('',#64950);
#13191=VERTEX_POINT('',#64956);
#13192=VERTEX_POINT('',#64960);
#13193=VERTEX_POINT('',#64962);
#13194=VERTEX_POINT('',#64965);
#13195=VERTEX_POINT('',#64967);
#13196=VERTEX_POINT('',#64975);
#13197=VERTEX_POINT('',#64981);
#13198=VERTEX_POINT('',#64987);
#13199=VERTEX_POINT('',#64989);
#13200=VERTEX_POINT('',#64995);
#13201=VERTEX_POINT('',#65001);
#13202=VERTEX_POINT('',#65012);
#13203=VERTEX_POINT('',#65016);
#13204=VERTEX_POINT('',#65018);
#13205=VERTEX_POINT('',#65031);
#13206=VERTEX_POINT('',#65033);
#13207=VERTEX_POINT('',#65035);
#13208=VERTEX_POINT('',#65037);
#13209=VERTEX_POINT('',#65039);
#13210=VERTEX_POINT('',#65041);
#13211=VERTEX_POINT('',#65045);
#13212=VERTEX_POINT('',#65047);
#13213=VERTEX_POINT('',#65049);
#13214=VERTEX_POINT('',#65052);
#13215=VERTEX_POINT('',#65053);
#13216=VERTEX_POINT('',#65057);
#13217=VERTEX_POINT('',#65061);
#13218=VERTEX_POINT('',#65065);
#13219=VERTEX_POINT('',#65069);
#13220=VERTEX_POINT('',#65073);
#13221=VERTEX_POINT('',#65077);
#13222=VERTEX_POINT('',#65081);
#13223=VERTEX_POINT('',#65085);
#13224=VERTEX_POINT('',#65092);
#13225=VERTEX_POINT('',#65093);
#13226=VERTEX_POINT('',#65095);
#13227=VERTEX_POINT('',#65097);
#13228=VERTEX_POINT('',#65100);
#13229=VERTEX_POINT('',#65102);
#13230=VERTEX_POINT('',#65103);
#13231=VERTEX_POINT('',#65105);
#13232=VERTEX_POINT('',#65107);
#13233=VERTEX_POINT('',#65109);
#13234=VERTEX_POINT('',#65111);
#13235=VERTEX_POINT('',#65113);
#13236=VERTEX_POINT('',#65115);
#13237=VERTEX_POINT('',#65117);
#13238=VERTEX_POINT('',#65119);
#13239=VERTEX_POINT('',#65122);
#13240=VERTEX_POINT('',#65123);
#13241=VERTEX_POINT('',#65125);
#13242=VERTEX_POINT('',#65127);
#13243=VERTEX_POINT('',#65129);
#13244=VERTEX_POINT('',#65133);
#13245=VERTEX_POINT('',#65137);
#13246=VERTEX_POINT('',#65139);
#13247=VERTEX_POINT('',#65143);
#13248=VERTEX_POINT('',#65152);
#13249=VERTEX_POINT('',#65160);
#13250=VERTEX_POINT('',#65162);
#13251=VERTEX_POINT('',#65166);
#13252=VERTEX_POINT('',#65170);
#13253=VERTEX_POINT('',#65172);
#13254=VERTEX_POINT('',#65174);
#13255=VERTEX_POINT('',#65176);
#13256=VERTEX_POINT('',#65178);
#13257=VERTEX_POINT('',#65180);
#13258=VERTEX_POINT('',#65182);
#13259=VERTEX_POINT('',#65185);
#13260=VERTEX_POINT('',#65187);
#13261=VERTEX_POINT('',#65189);
#13262=VERTEX_POINT('',#65192);
#13263=VERTEX_POINT('',#65196);
#13264=VERTEX_POINT('',#65211);
#13265=VERTEX_POINT('',#65215);
#13266=VERTEX_POINT('',#65219);
#13267=VERTEX_POINT('',#65221);
#13268=VERTEX_POINT('',#65223);
#13269=VERTEX_POINT('',#65227);
#13270=VERTEX_POINT('',#65229);
#13271=VERTEX_POINT('',#65231);
#13272=VERTEX_POINT('',#65241);
#13273=VERTEX_POINT('',#65245);
#13274=VERTEX_POINT('',#65252);
#13275=VERTEX_POINT('',#65259);
#13276=VERTEX_POINT('',#65261);
#13277=VERTEX_POINT('',#65271);
#13278=VERTEX_POINT('',#65275);
#13279=VERTEX_POINT('',#65277);
#13280=VERTEX_POINT('',#65324);
#13281=VERTEX_POINT('',#65332);
#13282=VERTEX_POINT('',#65334);
#13283=VERTEX_POINT('',#65338);
#13284=VERTEX_POINT('',#65340);
#13285=VERTEX_POINT('',#65344);
#13286=VERTEX_POINT('',#65346);
#13287=VERTEX_POINT('',#65350);
#13288=VERTEX_POINT('',#65352);
#13289=VERTEX_POINT('',#65356);
#13290=VERTEX_POINT('',#65358);
#13291=VERTEX_POINT('',#65360);
#13292=VERTEX_POINT('',#65364);
#13293=VERTEX_POINT('',#65365);
#13294=VERTEX_POINT('',#65367);
#13295=VERTEX_POINT('',#65369);
#13296=VERTEX_POINT('',#65398);
#13297=VERTEX_POINT('',#65402);
#13298=VERTEX_POINT('',#65404);
#13299=VERTEX_POINT('',#65408);
#13300=VERTEX_POINT('',#65427);
#13301=VERTEX_POINT('',#65428);
#13302=VERTEX_POINT('',#65452);
#13303=VERTEX_POINT('',#65465);
#13304=VERTEX_POINT('',#65467);
#13305=VERTEX_POINT('',#65471);
#13306=VERTEX_POINT('',#65475);
#13307=VERTEX_POINT('',#65484);
#13308=VERTEX_POINT('',#65495);
#13309=VERTEX_POINT('',#65501);
#13310=VERTEX_POINT('',#65510);
#13311=VERTEX_POINT('',#65521);
#13312=VERTEX_POINT('',#65530);
#13313=VERTEX_POINT('',#65532);
#13314=VERTEX_POINT('',#65536);
#13315=VERTEX_POINT('',#65540);
#13316=VERTEX_POINT('',#65544);
#13317=VERTEX_POINT('',#65548);
#13318=VERTEX_POINT('',#65552);
#13319=VERTEX_POINT('',#65556);
#13320=VERTEX_POINT('',#65560);
#13321=VERTEX_POINT('',#65564);
#13322=VERTEX_POINT('',#65576);
#13323=VERTEX_POINT('',#65577);
#13324=VERTEX_POINT('',#65581);
#13325=VERTEX_POINT('',#65583);
#13326=VERTEX_POINT('',#65594);
#13327=VERTEX_POINT('',#65598);
#13328=VERTEX_POINT('',#65609);
#13329=VERTEX_POINT('',#65613);
#13330=VERTEX_POINT('',#65624);
#13331=VERTEX_POINT('',#65628);
#13332=VERTEX_POINT('',#65639);
#13333=VERTEX_POINT('',#65643);
#13334=VERTEX_POINT('',#65654);
#13335=VERTEX_POINT('',#65658);
#13336=VERTEX_POINT('',#65669);
#13337=VERTEX_POINT('',#65673);
#13338=VERTEX_POINT('',#65696);
#13339=VERTEX_POINT('',#65698);
#13340=VERTEX_POINT('',#65709);
#13341=VERTEX_POINT('',#65720);
#13342=VERTEX_POINT('',#65731);
#13343=VERTEX_POINT('',#65742);
#13344=VERTEX_POINT('',#65753);
#13345=VERTEX_POINT('',#65764);
#13346=VERTEX_POINT('',#65775);
#13347=VERTEX_POINT('',#65786);
#13348=VERTEX_POINT('',#65802);
#13349=VERTEX_POINT('',#65804);
#13350=VERTEX_POINT('',#65808);
#13351=VERTEX_POINT('',#65812);
#13352=VERTEX_POINT('',#65819);
#13353=VERTEX_POINT('',#65824);
#13354=VERTEX_POINT('',#65839);
#13355=VERTEX_POINT('',#65849);
#13356=VERTEX_POINT('',#65858);
#13357=VERTEX_POINT('',#65862);
#13358=VERTEX_POINT('',#65865);
#13359=VERTEX_POINT('',#65869);
#13360=VERTEX_POINT('',#65872);
#13361=VERTEX_POINT('',#65876);
#13362=VERTEX_POINT('',#65883);
#13363=VERTEX_POINT('',#65887);
#13364=VERTEX_POINT('',#65893);
#13365=VERTEX_POINT('',#65912);
#13366=VERTEX_POINT('',#65935);
#13367=VERTEX_POINT('',#65937);
#13368=VERTEX_POINT('',#65941);
#13369=VERTEX_POINT('',#65945);
#13370=VERTEX_POINT('',#65951);
#13371=VERTEX_POINT('',#65955);
#13372=VERTEX_POINT('',#65961);
#13373=VERTEX_POINT('',#65965);
#13374=VERTEX_POINT('',#65969);
#13375=VERTEX_POINT('',#65973);
#13376=VERTEX_POINT('',#65980);
#13377=VERTEX_POINT('',#65984);
#16437=EDGE_CURVE('',#12931,#12932,#10923,.T.);
#16438=EDGE_CURVE('',#12932,#12933,#10924,.T.);
#16439=EDGE_CURVE('',#12933,#12934,#1398,.T.);
#16440=EDGE_CURVE('',#12934,#12935,#10925,.T.);
#16441=EDGE_CURVE('',#12935,#12931,#1399,.T.);
#16442=EDGE_CURVE('',#12936,#12937,#7613,.T.);
#16443=EDGE_CURVE('',#12937,#12934,#10926,.T.);
#16444=EDGE_CURVE('',#12933,#12938,#7614,.T.);
#16445=EDGE_CURVE('',#12938,#12939,#1400,.T.);
#16446=EDGE_CURVE('',#12939,#12936,#10927,.T.);
#16447=EDGE_CURVE('',#12940,#12931,#7615,.T.);
#16448=EDGE_CURVE('',#12935,#12941,#10928,.T.);
#16449=EDGE_CURVE('',#12941,#12942,#7616,.T.);
#16450=EDGE_CURVE('',#12942,#12943,#10929,.T.);
#16451=EDGE_CURVE('',#12943,#12940,#1401,.T.);
#16452=EDGE_CURVE('',#12938,#12944,#10930,.T.);
#16453=EDGE_CURVE('',#12944,#12940,#10931,.T.);
#16454=EDGE_CURVE('',#12943,#12939,#10932,.T.);
#16455=EDGE_CURVE('',#12945,#12941,#7617,.T.);
#16456=EDGE_CURVE('',#12946,#12945,#7618,.T.);
#16457=EDGE_CURVE('',#12946,#12942,#7619,.T.);
#16458=EDGE_CURVE('',#12937,#12947,#7620,.T.);
#16459=EDGE_CURVE('',#12948,#12947,#7621,.T.);
#16460=EDGE_CURVE('',#12949,#12948,#7622,.T.);
#16461=EDGE_CURVE('',#12950,#12949,#10933,.F.);
#16462=EDGE_CURVE('',#12945,#12950,#7623,.T.);
#16463=EDGE_CURVE('',#12951,#12951,#10934,.T.);
#16464=EDGE_CURVE('',#12951,#12944,#7624,.T.);
#16465=EDGE_CURVE('',#12932,#12952,#7625,.T.);
#16466=EDGE_CURVE('',#12952,#12952,#10935,.T.);
#16467=EDGE_CURVE('',#12953,#12954,#103,.T.);
#16468=EDGE_CURVE('',#12954,#12955,#7626,.T.);
#16469=EDGE_CURVE('',#12955,#12956,#104,.T.);
#16470=EDGE_CURVE('',#12956,#12957,#7627,.T.);
#16471=EDGE_CURVE('',#12957,#12953,#105,.T.);
#16472=EDGE_CURVE('',#12958,#12956,#7628,.T.);
#16473=EDGE_CURVE('',#12958,#12959,#7629,.T.);
#16474=EDGE_CURVE('',#12960,#12959,#7630,.T.);
#16475=EDGE_CURVE('',#12961,#12960,#7631,.T.);
#16476=EDGE_CURVE('',#12957,#12961,#7632,.T.);
#16477=EDGE_CURVE('',#12955,#12962,#7633,.T.);
#16478=EDGE_CURVE('',#12963,#12962,#7634,.T.);
#16479=EDGE_CURVE('',#12963,#12956,#7635,.T.);
#16480=EDGE_CURVE('',#12964,#12954,#7636,.T.);
#16481=EDGE_CURVE('',#12962,#12964,#7637,.T.);
#16482=EDGE_CURVE('',#12965,#12966,#106,.T.);
#16483=EDGE_CURVE('',#12966,#12967,#7638,.T.);
#16484=EDGE_CURVE('',#12967,#12968,#107,.T.);
#16485=EDGE_CURVE('',#12968,#12969,#108,.T.);
#16486=EDGE_CURVE('',#12969,#12965,#7639,.T.);
#16487=EDGE_CURVE('',#12965,#12970,#7640,.T.);
#16488=EDGE_CURVE('',#12970,#12971,#7641,.T.);
#16489=EDGE_CURVE('',#12971,#12966,#7642,.T.);
#16490=EDGE_CURVE('',#12972,#12969,#7643,.T.);
#16491=EDGE_CURVE('',#12973,#12972,#7644,.T.);
#16492=EDGE_CURVE('',#12974,#12973,#7645,.T.);
#16493=EDGE_CURVE('',#12975,#12974,#7646,.T.);
#16494=EDGE_CURVE('',#12965,#12975,#7647,.T.);
#16495=EDGE_CURVE('',#12968,#12976,#109,.T.);
#16496=EDGE_CURVE('',#12976,#12977,#7648,.T.);
#16497=EDGE_CURVE('',#12977,#12972,#10936,.F.);
#16498=EDGE_CURVE('',#12961,#12978,#10937,.F.);
#16499=EDGE_CURVE('',#12979,#12961,#10938,.F.);
#16500=EDGE_CURVE('',#12978,#12979,#10939,.F.);
#16501=EDGE_CURVE('',#12980,#12979,#7649,.T.);
#16502=EDGE_CURVE('',#12960,#12980,#110,.T.);
#16503=EDGE_CURVE('',#12972,#12981,#10940,.F.);
#16504=EDGE_CURVE('',#12981,#12977,#10941,.F.);
#16505=EDGE_CURVE('',#12982,#12983,#7650,.T.);
#16506=EDGE_CURVE('',#12983,#12984,#111,.T.);
#16507=EDGE_CURVE('',#12984,#12985,#7651,.T.);
#16508=EDGE_CURVE('',#12985,#12982,#112,.T.);
#16509=EDGE_CURVE('',#12983,#12981,#7652,.T.);
#16510=EDGE_CURVE('',#12977,#12984,#7653,.T.);
#16511=EDGE_CURVE('',#12981,#12986,#7654,.T.);
#16512=EDGE_CURVE('',#12986,#12973,#113,.T.);
#16513=EDGE_CURVE('',#12987,#12982,#7655,.T.);
#16514=EDGE_CURVE('',#12985,#12988,#7656,.T.);
#16515=EDGE_CURVE('',#12988,#12987,#114,.T.);
#16516=EDGE_CURVE('',#12986,#12989,#7657,.T.);
#16517=EDGE_CURVE('',#12989,#12974,#10942,.T.);
#16518=EDGE_CURVE('',#12990,#12959,#10943,.T.);
#16519=EDGE_CURVE('',#12959,#12974,#10944,.T.);
#16520=EDGE_CURVE('',#12989,#12990,#10945,.T.);
#16521=EDGE_CURVE('',#12990,#12980,#7658,.T.);
#16522=EDGE_CURVE('',#12991,#12987,#7659,.T.);
#16523=EDGE_CURVE('',#12988,#12992,#7660,.T.);
#16524=EDGE_CURVE('',#12992,#12991,#115,.T.);
#16525=EDGE_CURVE('',#12992,#12978,#7661,.T.);
#16526=EDGE_CURVE('',#12979,#12991,#7662,.T.);
#16527=EDGE_CURVE('',#12978,#12993,#7663,.T.);
#16528=EDGE_CURVE('',#12993,#12953,#116,.T.);
#16529=EDGE_CURVE('',#12993,#12994,#7664,.T.);
#16530=EDGE_CURVE('',#12994,#12964,#7665,.T.);
#16531=EDGE_CURVE('',#12995,#12976,#7666,.T.);
#16532=EDGE_CURVE('',#12996,#12995,#10946,.T.);
#16533=EDGE_CURVE('',#12997,#12996,#7667,.T.);
#16534=EDGE_CURVE('',#12998,#12997,#10947,.T.);
#16535=EDGE_CURVE('',#12999,#12998,#7668,.T.);
#16536=EDGE_CURVE('',#13000,#12999,#10948,.T.);
#16537=EDGE_CURVE('',#13001,#13000,#7669,.T.);
#16538=EDGE_CURVE('',#12994,#13001,#10949,.T.);
#16539=EDGE_CURVE('',#13002,#13002,#10950,.T.);
#16540=EDGE_CURVE('',#13003,#13003,#10951,.T.);
#16541=EDGE_CURVE('',#13004,#13004,#10952,.T.);
#16542=EDGE_CURVE('',#13005,#13005,#10953,.T.);
#16543=EDGE_CURVE('',#13006,#12986,#7670,.T.);
#16544=EDGE_CURVE('',#13007,#13006,#7671,.T.);
#16545=EDGE_CURVE('',#13008,#13007,#7672,.T.);
#16546=EDGE_CURVE('',#13009,#13008,#7673,.T.);
#16547=EDGE_CURVE('',#12980,#13009,#7674,.T.);
#16548=EDGE_CURVE('',#13010,#13010,#10954,.T.);
#16549=EDGE_CURVE('',#12983,#13006,#7675,.T.);
#16550=EDGE_CURVE('',#12982,#13007,#7676,.T.);
#16551=EDGE_CURVE('',#13011,#13011,#10955,.T.);
#16552=EDGE_CURVE('',#13011,#13012,#10956,.T.);
#16553=EDGE_CURVE('',#13012,#13012,#10957,.T.);
#16554=EDGE_CURVE('',#13013,#13013,#10958,.T.);
#16555=EDGE_CURVE('',#13013,#13011,#7677,.T.);
#16556=EDGE_CURVE('',#13014,#13014,#10959,.T.);
#16557=EDGE_CURVE('',#13002,#13013,#10960,.T.);
#16558=EDGE_CURVE('',#13015,#13015,#10961,.T.);
#16559=EDGE_CURVE('',#13015,#13016,#10962,.T.);
#16560=EDGE_CURVE('',#13016,#13016,#10963,.T.);
#16561=EDGE_CURVE('',#13017,#13017,#10964,.T.);
#16562=EDGE_CURVE('',#13017,#13015,#7678,.T.);
#16563=EDGE_CURVE('',#13018,#13018,#10965,.T.);
#16564=EDGE_CURVE('',#13005,#13017,#10966,.T.);
#16565=EDGE_CURVE('',#13003,#13019,#10967,.T.);
#16566=EDGE_CURVE('',#13019,#13019,#10968,.T.);
#16567=EDGE_CURVE('',#13019,#13020,#7679,.T.);
#16568=EDGE_CURVE('',#13020,#13020,#10969,.T.);
#16569=EDGE_CURVE('',#13004,#13021,#10970,.T.);
#16570=EDGE_CURVE('',#13021,#13021,#10971,.T.);
#16571=EDGE_CURVE('',#13021,#13022,#7680,.T.);
#16572=EDGE_CURVE('',#13022,#13022,#10972,.T.);
#16573=EDGE_CURVE('',#13023,#13024,#10973,.F.);
#16574=EDGE_CURVE('',#13025,#13023,#10974,.F.);
#16575=EDGE_CURVE('',#13024,#13025,#10975,.F.);
#16576=EDGE_CURVE('',#13026,#13027,#10976,.F.);
#16577=EDGE_CURVE('',#13028,#13026,#10977,.F.);
#16578=EDGE_CURVE('',#13027,#13028,#10978,.F.);
#16579=EDGE_CURVE('',#13023,#13028,#7681,.T.);
#16580=EDGE_CURVE('',#13026,#13025,#7682,.T.);
#16581=EDGE_CURVE('',#13029,#13030,#1402,.F.);
#16582=EDGE_CURVE('',#13030,#13027,#7683,.T.);
#16583=EDGE_CURVE('',#13028,#13029,#7684,.T.);
#16584=EDGE_CURVE('',#13031,#13032,#1403,.T.);
#16585=EDGE_CURVE('',#13032,#13026,#10979,.T.);
#16586=EDGE_CURVE('',#13027,#13031,#10980,.T.);
#16587=EDGE_CURVE('',#13033,#13034,#1404,.T.);
#16588=EDGE_CURVE('',#13034,#13024,#10981,.T.);
#16589=EDGE_CURVE('',#13025,#13033,#10982,.T.);
#16590=EDGE_CURVE('',#13035,#13036,#1405,.F.);
#16591=EDGE_CURVE('',#13036,#13023,#7685,.T.);
#16592=EDGE_CURVE('',#13024,#13035,#7686,.T.);
#16593=EDGE_CURVE('',#13037,#13030,#10983,.T.);
#16594=EDGE_CURVE('',#13038,#13037,#7687,.T.);
#16595=EDGE_CURVE('',#13038,#13039,#10984,.T.);
#16596=EDGE_CURVE('',#13039,#13031,#7688,.T.);
#16597=EDGE_CURVE('',#13029,#13040,#7689,.T.);
#16598=EDGE_CURVE('',#13041,#13036,#7690,.T.);
#16599=EDGE_CURVE('',#13041,#13042,#7691,.T.);
#16600=EDGE_CURVE('',#13043,#13042,#7692,.T.);
#16601=EDGE_CURVE('',#13043,#13040,#7693,.T.);
#16602=EDGE_CURVE('',#13044,#13045,#1406,.T.);
#16603=EDGE_CURVE('',#13045,#13046,#7694,.T.);
#16604=EDGE_CURVE('',#13046,#13047,#10985,.T.);
#16605=EDGE_CURVE('',#13047,#13044,#7695,.T.);
#16606=EDGE_CURVE('',#13048,#13049,#1407,.F.);
#16607=EDGE_CURVE('',#13049,#13050,#7696,.F.);
#16608=EDGE_CURVE('',#13051,#13050,#10986,.T.);
#16609=EDGE_CURVE('',#13051,#13052,#7697,.T.);
#16610=EDGE_CURVE('',#13052,#13046,#10987,.T.);
#16611=EDGE_CURVE('',#13046,#13048,#7698,.T.);
#16612=EDGE_CURVE('',#13052,#13047,#10988,.T.);
#16613=EDGE_CURVE('',#13053,#13044,#10989,.T.);
#16614=EDGE_CURVE('',#13054,#13053,#7699,.T.);
#16615=EDGE_CURVE('',#13055,#13054,#10990,.T.);
#16616=EDGE_CURVE('',#13056,#13055,#1408,.T.);
#16617=EDGE_CURVE('',#13057,#13056,#7700,.T.);
#16618=EDGE_CURVE('',#13058,#13057,#10991,.T.);
#16619=EDGE_CURVE('',#13059,#13058,#7701,.T.);
#16620=EDGE_CURVE('',#13060,#13059,#1409,.T.);
#16621=EDGE_CURVE('',#13061,#13060,#10992,.T.);
#16622=EDGE_CURVE('',#13061,#13045,#7702,.T.);
#16623=EDGE_CURVE('',#13062,#13047,#10993,.T.);
#16624=EDGE_CURVE('',#13063,#13062,#7703,.T.);
#16625=EDGE_CURVE('',#13063,#13064,#7704,.T.);
#16626=EDGE_CURVE('',#13064,#13053,#7705,.T.);
#16627=EDGE_CURVE('',#13052,#13065,#10994,.T.);
#16628=EDGE_CURVE('',#13065,#13062,#10995,.T.);
#16629=EDGE_CURVE('',#13066,#13051,#10996,.T.);
#16630=EDGE_CURVE('',#13067,#13066,#7706,.T.);
#16631=EDGE_CURVE('',#13068,#13067,#10997,.T.);
#16632=EDGE_CURVE('',#13069,#13068,#7707,.T.);
#16633=EDGE_CURVE('',#13070,#13069,#10998,.T.);
#16634=EDGE_CURVE('',#13065,#13070,#7708,.T.);
#16635=EDGE_CURVE('',#13071,#13072,#10999,.T.);
#16636=EDGE_CURVE('',#13073,#13071,#7709,.T.);
#16637=EDGE_CURVE('',#13073,#13074,#11000,.T.);
#16638=EDGE_CURVE('',#13072,#13074,#7710,.T.);
#16639=EDGE_CURVE('',#13075,#13076,#1410,.T.);
#16640=EDGE_CURVE('',#13075,#13077,#7711,.T.);
#16641=EDGE_CURVE('',#13077,#13069,#11001,.T.);
#16642=EDGE_CURVE('',#13068,#13078,#11002,.F.);
#16643=EDGE_CURVE('',#13076,#13078,#7712,.T.);
#16644=EDGE_CURVE('',#13079,#13080,#1411,.T.);
#16645=EDGE_CURVE('',#13080,#13081,#7713,.T.);
#16646=EDGE_CURVE('',#13081,#13077,#11003,.T.);
#16647=EDGE_CURVE('',#13077,#13079,#7714,.T.);
#16648=EDGE_CURVE('',#13081,#13069,#11004,.T.);
#16649=EDGE_CURVE('',#13081,#13082,#11005,.T.);
#16650=EDGE_CURVE('',#13070,#13082,#11006,.T.);
#16651=EDGE_CURVE('',#13080,#13083,#11007,.T.);
#16652=EDGE_CURVE('',#13083,#13084,#7715,.T.);
#16653=EDGE_CURVE('',#13084,#13085,#7716,.T.);
#16654=EDGE_CURVE('',#13082,#13085,#7717,.T.);
#16655=EDGE_CURVE('',#13079,#13086,#7718,.T.);
#16656=EDGE_CURVE('',#13087,#13086,#11008,.T.);
#16657=EDGE_CURVE('',#13088,#13087,#1412,.T.);
#16658=EDGE_CURVE('',#13089,#13088,#7719,.T.);
#16659=EDGE_CURVE('',#13090,#13089,#11009,.T.);
#16660=EDGE_CURVE('',#13091,#13090,#7720,.T.);
#16661=EDGE_CURVE('',#13092,#13091,#1413,.T.);
#16662=EDGE_CURVE('',#13093,#13092,#11010,.T.);
#16663=EDGE_CURVE('',#13083,#13093,#7721,.T.);
#16664=EDGE_CURVE('',#13074,#13094,#1414,.F.);
#16665=EDGE_CURVE('',#13094,#13095,#7722,.T.);
#16666=EDGE_CURVE('',#13095,#13072,#1415,.F.);
#16667=EDGE_CURVE('',#13096,#13094,#1416,.F.);
#16668=EDGE_CURVE('',#13097,#13096,#7723,.T.);
#16669=EDGE_CURVE('',#13098,#13097,#7724,.T.);
#16670=EDGE_CURVE('',#13098,#13099,#7725,.T.);
#16671=EDGE_CURVE('',#13095,#13099,#1417,.F.);
#16672=EDGE_CURVE('',#13100,#13100,#11011,.T.);
#16673=EDGE_CURVE('',#13100,#13101,#11012,.T.);
#16674=EDGE_CURVE('',#13101,#13102,#11013,.T.);
#16675=EDGE_CURVE('',#13102,#13101,#11014,.T.);
#16676=EDGE_CURVE('',#13103,#13104,#11015,.T.);
#16677=EDGE_CURVE('',#13105,#13103,#7726,.T.);
#16678=EDGE_CURVE('',#13106,#13105,#7727,.T.);
#16679=EDGE_CURVE('',#13107,#13106,#7728,.T.);
#16680=EDGE_CURVE('',#13067,#13107,#7729,.T.);
#16681=EDGE_CURVE('',#13108,#13066,#7730,.T.);
#16682=EDGE_CURVE('',#13109,#13108,#7731,.T.);
#16683=EDGE_CURVE('',#13110,#13109,#7732,.T.);
#16684=EDGE_CURVE('',#13111,#13110,#7733,.T.);
#16685=EDGE_CURVE('',#13104,#13111,#11016,.T.);
#16686=EDGE_CURVE('',#13112,#13112,#11017,.T.);
#16687=EDGE_CURVE('',#13113,#13113,#11018,.T.);
#16688=EDGE_CURVE('',#13114,#13114,#11019,.T.);
#16689=EDGE_CURVE('',#13114,#13102,#7734,.T.);
#16690=EDGE_CURVE('',#13112,#13115,#11020,.T.);
#16691=EDGE_CURVE('',#13115,#13116,#11021,.T.);
#16692=EDGE_CURVE('',#13116,#13115,#11022,.T.);
#16693=EDGE_CURVE('',#13117,#13117,#11023,.T.);
#16694=EDGE_CURVE('',#13117,#13116,#7735,.T.);
#16695=EDGE_CURVE('',#13113,#13118,#11024,.T.);
#16696=EDGE_CURVE('',#13118,#13119,#11025,.T.);
#16697=EDGE_CURVE('',#13119,#13118,#11026,.T.);
#16698=EDGE_CURVE('',#13120,#13120,#11027,.T.);
#16699=EDGE_CURVE('',#13120,#13119,#7736,.T.);
#16700=EDGE_CURVE('',#13111,#13103,#1418,.T.);
#16701=EDGE_CURVE('',#13104,#13121,#11028,.T.);
#16702=EDGE_CURVE('',#13121,#13122,#11029,.T.);
#16703=EDGE_CURVE('',#13122,#13121,#11030,.T.);
#16704=EDGE_CURVE('',#13123,#13110,#1419,.T.);
#16705=EDGE_CURVE('',#13124,#13123,#7737,.T.);
#16706=EDGE_CURVE('',#13125,#13124,#117,.T.);
#16707=EDGE_CURVE('',#13126,#13125,#7738,.T.);
#16708=EDGE_CURVE('',#13127,#13126,#118,.T.);
#16709=EDGE_CURVE('',#13128,#13127,#7739,.T.);
#16710=EDGE_CURVE('',#13105,#13128,#1420,.T.);
#16711=EDGE_CURVE('',#13129,#13129,#11031,.T.);
#16712=EDGE_CURVE('',#13129,#13122,#7740,.T.);
#16713=EDGE_CURVE('',#13073,#13130,#1421,.T.);
#16714=EDGE_CURVE('',#13071,#13131,#1422,.F.);
#16715=EDGE_CURVE('',#13131,#13132,#11032,.F.);
#16716=EDGE_CURVE('',#13132,#13133,#7741,.T.);
#16717=EDGE_CURVE('',#13130,#13133,#11033,.T.);
#16718=EDGE_CURVE('',#13134,#13132,#7742,.T.);
#16719=EDGE_CURVE('',#13134,#13135,#7743,.T.);
#16720=EDGE_CURVE('',#13136,#13135,#7744,.F.);
#16721=EDGE_CURVE('',#13137,#13136,#7745,.T.);
#16722=EDGE_CURVE('',#12949,#13137,#7746,.T.);
#16723=EDGE_CURVE('',#12948,#13138,#7747,.T.);
#16724=EDGE_CURVE('',#13138,#13139,#7748,.T.);
#16725=EDGE_CURVE('',#13139,#13133,#7749,.T.);
#16726=EDGE_CURVE('',#13140,#13140,#11034,.T.);
#16727=EDGE_CURVE('',#13141,#13141,#11035,.T.);
#16728=EDGE_CURVE('',#13142,#13142,#11036,.T.);
#16729=EDGE_CURVE('',#13143,#13143,#11037,.T.);
#16730=EDGE_CURVE('',#13010,#13144,#11038,.T.);
#16731=EDGE_CURVE('',#13144,#13144,#11039,.T.);
#16732=EDGE_CURVE('',#13144,#13145,#7750,.T.);
#16733=EDGE_CURVE('',#13146,#13145,#11040,.T.);
#16734=EDGE_CURVE('',#13145,#13146,#11041,.T.);
#16735=EDGE_CURVE('',#13147,#13148,#1423,.T.);
#16736=EDGE_CURVE('',#13148,#13149,#11042,.T.);
#16737=EDGE_CURVE('',#13149,#13150,#1424,.T.);
#16738=EDGE_CURVE('',#13150,#13147,#11043,.T.);
#16739=EDGE_CURVE('',#13151,#13150,#7751,.T.);
#16740=EDGE_CURVE('',#13152,#13151,#11044,.T.);
#16741=EDGE_CURVE('',#13147,#13152,#7752,.T.);
#16742=EDGE_CURVE('',#13153,#13149,#7753,.T.);
#16743=EDGE_CURVE('',#13154,#13153,#7754,.T.);
#16744=EDGE_CURVE('',#13150,#13154,#7755,.T.);
#16745=EDGE_CURVE('',#13151,#13155,#1425,.T.);
#16746=EDGE_CURVE('',#13155,#13156,#11045,.T.);
#16747=EDGE_CURVE('',#13156,#13152,#1426,.T.);
#16748=EDGE_CURVE('',#13155,#13157,#7756,.T.);
#16749=EDGE_CURVE('',#13157,#13158,#11046,.T.);
#16750=EDGE_CURVE('',#13158,#13156,#7757,.T.);
#16751=EDGE_CURVE('',#13159,#13151,#7758,.T.);
#16752=EDGE_CURVE('',#13157,#13159,#7759,.T.);
#16753=EDGE_CURVE('',#13160,#13160,#11047,.T.);
#16754=EDGE_CURVE('',#13160,#13146,#11048,.T.);
#16755=EDGE_CURVE('',#12975,#12958,#11049,.T.);
#16756=EDGE_CURVE('',#13161,#12963,#11050,.T.);
#16757=EDGE_CURVE('',#13162,#13161,#7760,.T.);
#16758=EDGE_CURVE('',#13163,#13162,#11051,.T.);
#16759=EDGE_CURVE('',#13164,#13163,#7761,.T.);
#16760=EDGE_CURVE('',#13165,#13164,#11052,.T.);
#16761=EDGE_CURVE('',#13166,#13165,#7762,.T.);
#16762=EDGE_CURVE('',#12970,#13166,#11053,.T.);
#16763=EDGE_CURVE('',#13167,#13167,#11054,.T.);
#16764=EDGE_CURVE('',#13168,#13168,#11055,.T.);
#16765=EDGE_CURVE('',#13169,#13169,#11056,.T.);
#16766=EDGE_CURVE('',#13170,#13170,#11057,.T.);
#16767=EDGE_CURVE('',#13171,#13172,#7763,.T.);
#16768=EDGE_CURVE('',#13173,#13171,#7764,.T.);
#16769=EDGE_CURVE('',#13173,#13174,#7765,.T.);
#16770=EDGE_CURVE('',#13174,#13042,#7766,.T.);
#16771=EDGE_CURVE('',#13043,#13042,#7767,.T.);
#16772=EDGE_CURVE('',#13043,#13175,#7768,.T.);
#16773=EDGE_CURVE('',#13175,#13176,#7769,.T.);
#16774=EDGE_CURVE('',#13177,#13176,#7770,.T.);
#16775=EDGE_CURVE('',#13178,#13177,#7771,.T.);
#16776=EDGE_CURVE('',#13178,#13043,#7772,.T.);
#16777=EDGE_CURVE('',#13042,#13172,#7773,.T.);
#16778=EDGE_CURVE('',#13179,#13137,#11058,.T.);
#16779=EDGE_CURVE('',#13126,#13179,#119,.T.);
#16780=EDGE_CURVE('',#13125,#12950,#120,.F.);
#16781=EDGE_CURVE('',#13140,#13129,#11059,.T.);
#16782=EDGE_CURVE('',#13143,#13120,#11060,.T.);
#16783=EDGE_CURVE('',#13141,#13117,#11061,.T.);
#16784=EDGE_CURVE('',#13142,#13114,#11062,.T.);
#16785=EDGE_CURVE('',#13180,#13181,#121,.T.);
#16786=EDGE_CURVE('',#13181,#13182,#7774,.T.);
#16787=EDGE_CURVE('',#13182,#13183,#122,.T.);
#16788=EDGE_CURVE('',#13183,#13184,#7775,.T.);
#16789=EDGE_CURVE('',#13184,#13185,#1427,.T.);
#16790=EDGE_CURVE('',#13185,#13186,#7776,.T.);
#16791=EDGE_CURVE('',#13186,#13187,#1428,.T.);
#16792=EDGE_CURVE('',#13187,#13180,#7777,.T.);
#16793=EDGE_CURVE('',#13180,#13063,#11063,.T.);
#16794=EDGE_CURVE('',#13065,#13181,#7778,.T.);
#16795=EDGE_CURVE('',#13187,#13188,#7779,.T.);
#16796=EDGE_CURVE('',#13189,#13188,#7780,.T.);
#16797=EDGE_CURVE('',#13189,#13064,#7781,.T.);
#16798=EDGE_CURVE('',#13186,#13190,#253,.T.);
#16799=EDGE_CURVE('',#13190,#13188,#11064,.T.);
#16800=EDGE_CURVE('',#13191,#13185,#254,.T.);
#16801=EDGE_CURVE('',#13192,#13191,#7782,.T.);
#16802=EDGE_CURVE('',#13193,#13192,#7783,.T.);
#16803=EDGE_CURVE('',#13193,#13043,#7784,.T.);
#16804=EDGE_CURVE('',#13042,#13194,#7785,.T.);
#16805=EDGE_CURVE('',#13195,#13194,#7786,.T.);
#16806=EDGE_CURVE('',#13190,#13195,#7787,.T.);
#16807=EDGE_CURVE('',#13182,#13070,#7788,.T.);
#16808=EDGE_CURVE('',#13099,#13131,#11065,.T.);
#16809=EDGE_CURVE('',#13196,#13098,#7789,.T.);
#16810=EDGE_CURVE('',#13134,#13196,#11066,.T.);
#16811=EDGE_CURVE('',#13130,#13096,#11067,.T.);
#16812=EDGE_CURVE('',#13197,#13139,#11068,.T.);
#16813=EDGE_CURVE('',#13097,#13197,#7790,.T.);
#16814=EDGE_CURVE('',#13085,#13183,#11069,.T.);
#16815=EDGE_CURVE('',#13084,#13198,#7791,.T.);
#16816=EDGE_CURVE('',#13199,#13198,#7792,.T.);
#16817=EDGE_CURVE('',#13184,#13199,#7793,.T.);
#16818=EDGE_CURVE('',#13198,#13093,#7794,.T.);
#16819=EDGE_CURVE('',#13200,#13075,#255,.T.);
#16820=EDGE_CURVE('',#13086,#13200,#7795,.T.);
#16821=EDGE_CURVE('',#13201,#13076,#1429,.F.);
#16822=EDGE_CURVE('',#13201,#13106,#1430,.T.);
#16823=EDGE_CURVE('',#13106,#13202,#7796,.T.);
#16824=EDGE_CURVE('',#13202,#13200,#11070,.T.);
#16825=EDGE_CURVE('',#13087,#13203,#11071,.T.);
#16826=EDGE_CURVE('',#13204,#13203,#7797,.T.);
#16827=EDGE_CURVE('',#13204,#13088,#1431,.T.);
#16828=EDGE_CURVE('',#13205,#13202,#7798,.T.);
#16829=EDGE_CURVE('',#13206,#13205,#11072,.T.);
#16830=EDGE_CURVE('',#13207,#13206,#7799,.T.);
#16831=EDGE_CURVE('',#13208,#13207,#11073,.T.);
#16832=EDGE_CURVE('',#13209,#13208,#7800,.T.);
#16833=EDGE_CURVE('',#13210,#13209,#11074,.T.);
#16834=EDGE_CURVE('',#13192,#13210,#7801,.T.);
#16835=EDGE_CURVE('',#13199,#13191,#11075,.T.);
#16836=EDGE_CURVE('',#13211,#13092,#11076,.T.);
#16837=EDGE_CURVE('',#13212,#13211,#7802,.T.);
#16838=EDGE_CURVE('',#13213,#13212,#11077,.T.);
#16839=EDGE_CURVE('',#13203,#13213,#7803,.T.);
#16840=EDGE_CURVE('',#13214,#13215,#1432,.T.);
#16841=EDGE_CURVE('',#13215,#13216,#1433,.T.);
#16842=EDGE_CURVE('',#13216,#13217,#1434,.T.);
#16843=EDGE_CURVE('',#13217,#13218,#1435,.T.);
#16844=EDGE_CURVE('',#13218,#13219,#1436,.T.);
#16845=EDGE_CURVE('',#13219,#13220,#1437,.T.);
#16846=EDGE_CURVE('',#13220,#13221,#1438,.T.);
#16847=EDGE_CURVE('',#13221,#13222,#1439,.T.);
#16848=EDGE_CURVE('',#13222,#13223,#1440,.T.);
#16849=EDGE_CURVE('',#13223,#13214,#1441,.T.);
#16850=EDGE_CURVE('',#13224,#13225,#7804,.T.);
#16851=EDGE_CURVE('',#13225,#13226,#7805,.T.);
#16852=EDGE_CURVE('',#13226,#13227,#7806,.T.);
#16853=EDGE_CURVE('',#13227,#13224,#7807,.T.);
#16854=EDGE_CURVE('',#13228,#13228,#11078,.T.);
#16855=EDGE_CURVE('',#13229,#13230,#7808,.T.);
#16856=EDGE_CURVE('',#13230,#13231,#7809,.T.);
#16857=EDGE_CURVE('',#13231,#13232,#7810,.T.);
#16858=EDGE_CURVE('',#13232,#13233,#7811,.T.);
#16859=EDGE_CURVE('',#13233,#13234,#7812,.T.);
#16860=EDGE_CURVE('',#13234,#13235,#7813,.T.);
#16861=EDGE_CURVE('',#13235,#13236,#7814,.T.);
#16862=EDGE_CURVE('',#13236,#13237,#7815,.T.);
#16863=EDGE_CURVE('',#13237,#13238,#7816,.T.);
#16864=EDGE_CURVE('',#13238,#13229,#7817,.T.);
#16865=EDGE_CURVE('',#13239,#13240,#7818,.T.);
#16866=EDGE_CURVE('',#13240,#13241,#7819,.T.);
#16867=EDGE_CURVE('',#13241,#13242,#7820,.T.);
#16868=EDGE_CURVE('',#13242,#13243,#1442,.T.);
#16869=EDGE_CURVE('',#13243,#13244,#1443,.T.);
#16870=EDGE_CURVE('',#13244,#13245,#7821,.T.);
#16871=EDGE_CURVE('',#13245,#13246,#1444,.T.);
#16872=EDGE_CURVE('',#13246,#13247,#1445,.T.);
#16873=EDGE_CURVE('',#13247,#13239,#7822,.T.);
#16874=EDGE_CURVE('',#13078,#13107,#11079,.T.);
#16875=EDGE_CURVE('',#13248,#13061,#7823,.T.);
#16876=EDGE_CURVE('',#13048,#13248,#256,.T.);
#16877=EDGE_CURVE('',#13054,#13189,#7824,.T.);
#16878=EDGE_CURVE('',#13249,#13056,#11080,.T.);
#16879=EDGE_CURVE('',#13249,#13250,#7825,.T.);
#16880=EDGE_CURVE('',#13057,#13250,#11081,.T.);
#16881=EDGE_CURVE('',#13055,#13251,#11082,.T.);
#16882=EDGE_CURVE('',#13249,#13251,#7826,.T.);
#16883=EDGE_CURVE('',#13252,#13195,#7827,.T.);
#16884=EDGE_CURVE('',#13253,#13252,#11083,.T.);
#16885=EDGE_CURVE('',#13254,#13253,#7828,.T.);
#16886=EDGE_CURVE('',#13255,#13254,#11084,.T.);
#16887=EDGE_CURVE('',#13256,#13255,#7829,.T.);
#16888=EDGE_CURVE('',#13257,#13256,#11085,.T.);
#16889=EDGE_CURVE('',#13258,#13257,#7830,.T.);
#16890=EDGE_CURVE('',#13248,#13258,#11086,.T.);
#16891=EDGE_CURVE('',#13259,#13060,#11087,.T.);
#16892=EDGE_CURVE('',#13260,#13259,#7831,.T.);
#16893=EDGE_CURVE('',#13261,#13260,#11088,.T.);
#16894=EDGE_CURVE('',#13251,#13261,#7832,.T.);
#16895=EDGE_CURVE('',#13262,#13262,#11089,.T.);
#16896=EDGE_CURVE('',#13109,#13258,#7833,.T.);
#16897=EDGE_CURVE('',#13109,#13263,#1446,.T.);
#16898=EDGE_CURVE('',#13263,#13049,#1447,.T.);
#16899=EDGE_CURVE('',#13050,#13108,#11090,.T.);
#16900=EDGE_CURVE('',#13264,#13196,#7834,.T.);
#16901=EDGE_CURVE('',#13135,#13264,#123,.T.);
#16902=EDGE_CURVE('',#13265,#13138,#124,.T.);
#16903=EDGE_CURVE('',#13197,#13265,#7835,.T.);
#16904=EDGE_CURVE('',#13266,#13193,#7836,.T.);
#16905=EDGE_CURVE('',#13267,#13266,#11091,.T.);
#16906=EDGE_CURVE('',#13268,#13267,#7837,.T.);
#16907=EDGE_CURVE('',#13175,#13268,#11092,.T.);
#16908=EDGE_CURVE('',#13194,#13269,#7838,.T.);
#16909=EDGE_CURVE('',#13270,#13174,#11093,.T.);
#16910=EDGE_CURVE('',#13271,#13270,#7839,.T.);
#16911=EDGE_CURVE('',#13269,#13271,#11094,.T.);
#16912=EDGE_CURVE('',#13172,#13041,#11095,.T.);
#16913=EDGE_CURVE('',#13040,#13178,#11096,.T.);
#16914=EDGE_CURVE('',#13037,#13177,#125,.T.);
#16915=EDGE_CURVE('',#13035,#13272,#11097,.T.);
#16916=EDGE_CURVE('',#13171,#13272,#126,.T.);
#16917=EDGE_CURVE('',#13124,#13273,#7840,.T.);
#16918=EDGE_CURVE('',#13273,#12945,#7841,.T.);
#16919=EDGE_CURVE('',#13110,#13257,#7842,.T.);
#16920=EDGE_CURVE('',#13123,#13256,#7843,.T.);
#16921=EDGE_CURVE('',#13274,#13266,#127,.T.);
#16922=EDGE_CURVE('',#13267,#13274,#257,.T.);
#16923=EDGE_CURVE('',#13269,#13275,#128,.T.);
#16924=EDGE_CURVE('',#13275,#13276,#7844,.T.);
#16925=EDGE_CURVE('',#13276,#13252,#129,.T.);
#16926=EDGE_CURVE('',#13270,#13173,#130,.T.);
#16927=EDGE_CURVE('',#13275,#13271,#258,.T.);
#16928=EDGE_CURVE('',#13277,#13158,#7845,.T.);
#16929=EDGE_CURVE('',#13152,#13277,#7846,.T.);
#16930=EDGE_CURVE('',#13278,#13147,#7847,.T.);
#16931=EDGE_CURVE('',#13279,#13278,#7848,.T.);
#16932=EDGE_CURVE('',#13148,#13279,#7849,.T.);
#16933=EDGE_CURVE('',#13277,#13159,#1448,.T.);
#16934=EDGE_CURVE('',#13154,#13278,#1449,.T.);
#16935=EDGE_CURVE('',#13279,#13153,#11098,.T.);
#16936=EDGE_CURVE('',#13128,#13152,#7850,.T.);
#16937=EDGE_CURVE('',#13280,#13127,#7851,.T.);
#16938=EDGE_CURVE('',#13273,#13280,#7852,.T.);
#16939=EDGE_CURVE('',#13147,#13123,#7853,.T.);
#16940=EDGE_CURVE('',#13159,#13208,#7854,.T.);
#16941=EDGE_CURVE('',#13277,#13207,#7855,.T.);
#16942=EDGE_CURVE('',#13281,#13090,#11099,.T.);
#16943=EDGE_CURVE('',#13281,#13282,#7856,.T.);
#16944=EDGE_CURVE('',#13091,#13282,#11100,.T.);
#16945=EDGE_CURVE('',#13282,#13283,#7857,.T.);
#16946=EDGE_CURVE('',#13284,#13281,#7858,.T.);
#16947=EDGE_CURVE('',#13283,#13284,#7859,.T.);
#16948=EDGE_CURVE('',#13285,#13249,#7860,.T.);
#16949=EDGE_CURVE('',#13286,#13285,#7861,.T.);
#16950=EDGE_CURVE('',#13250,#13286,#7862,.T.);
#16951=EDGE_CURVE('',#13287,#13265,#7863,.T.);
#16952=EDGE_CURVE('',#13288,#13287,#7864,.T.);
#16953=EDGE_CURVE('',#13264,#13288,#7865,.T.);
#16954=EDGE_CURVE('',#13289,#13204,#7866,.T.);
#16955=EDGE_CURVE('',#13290,#13289,#7867,.T.);
#16956=EDGE_CURVE('',#13291,#13290,#7868,.T.);
#16957=EDGE_CURVE('',#13291,#13204,#7869,.T.);
#16958=EDGE_CURVE('',#13292,#13293,#7870,.T.);
#16959=EDGE_CURVE('',#13292,#13294,#7871,.T.);
#16960=EDGE_CURVE('',#13295,#13294,#7872,.T.);
#16961=EDGE_CURVE('',#13293,#13295,#7873,.T.);
#16962=EDGE_CURVE('',#13089,#13291,#11101,.T.);
#16963=EDGE_CURVE('',#13290,#13284,#11102,.T.);
#16964=EDGE_CURVE('',#13294,#13058,#11103,.T.);
#16965=EDGE_CURVE('',#13059,#13292,#1450,.T.);
#16966=EDGE_CURVE('',#13289,#13293,#7874,.T.);
#16967=EDGE_CURVE('',#13286,#13295,#11104,.T.);
#16968=EDGE_CURVE('',#13285,#13283,#7875,.T.);
#16969=EDGE_CURVE('',#13292,#13259,#7876,.T.);
#16970=EDGE_CURVE('',#12947,#13287,#7877,.T.);
#16971=EDGE_CURVE('',#13039,#13296,#7878,.T.);
#16972=EDGE_CURVE('',#13032,#13296,#7879,.T.);
#16973=EDGE_CURVE('',#13297,#13033,#7880,.T.);
#16974=EDGE_CURVE('',#13297,#13298,#7881,.T.);
#16975=EDGE_CURVE('',#13034,#13298,#7882,.T.);
#16976=EDGE_CURVE('',#13299,#13038,#131,.T.);
#16977=EDGE_CURVE('',#13296,#13299,#1451,.T.);
#16978=EDGE_CURVE('',#13300,#13301,#132,.T.);
#16979=EDGE_CURVE('',#13298,#13300,#11105,.T.);
#16980=EDGE_CURVE('',#13301,#13297,#1452,.T.);
#16981=EDGE_CURVE('',#13033,#13032,#7883,.T.);
#16982=EDGE_CURVE('',#13272,#13300,#7884,.T.);
#16983=EDGE_CURVE('',#13302,#13301,#259,.F.);
#16984=EDGE_CURVE('',#13302,#13276,#260,.T.);
#16985=EDGE_CURVE('',#13297,#13253,#7885,.T.);
#16986=EDGE_CURVE('',#13033,#13150,#7886,.T.);
#16987=EDGE_CURVE('',#13151,#13032,#7887,.T.);
#16988=EDGE_CURVE('',#13239,#13303,#7888,.T.);
#16989=EDGE_CURVE('',#13304,#13303,#7889,.T.);
#16990=EDGE_CURVE('',#13240,#13304,#7890,.T.);
#16991=EDGE_CURVE('',#13305,#13304,#7891,.T.);
#16992=EDGE_CURVE('',#13241,#13305,#7892,.T.);
#16993=EDGE_CURVE('',#13306,#13305,#7893,.T.);
#16994=EDGE_CURVE('',#13242,#13306,#7894,.T.);
#16995=EDGE_CURVE('',#13307,#13306,#1453,.T.);
#16996=EDGE_CURVE('',#13243,#13307,#7895,.T.);
#16997=EDGE_CURVE('',#13308,#13307,#1454,.T.);
#16998=EDGE_CURVE('',#13244,#13308,#7896,.T.);
#16999=EDGE_CURVE('',#13309,#13308,#7897,.T.);
#17000=EDGE_CURVE('',#13245,#13309,#7898,.T.);
#17001=EDGE_CURVE('',#13310,#13309,#1455,.T.);
#17002=EDGE_CURVE('',#13246,#13310,#7899,.T.);
#17003=EDGE_CURVE('',#13311,#13310,#1456,.T.);
#17004=EDGE_CURVE('',#13247,#13311,#7900,.T.);
#17005=EDGE_CURVE('',#13303,#13311,#7901,.T.);
#17006=EDGE_CURVE('',#13229,#13312,#7902,.T.);
#17007=EDGE_CURVE('',#13313,#13312,#7903,.T.);
#17008=EDGE_CURVE('',#13230,#13313,#7904,.T.);
#17009=EDGE_CURVE('',#13314,#13313,#7905,.T.);
#17010=EDGE_CURVE('',#13231,#13314,#7906,.T.);
#17011=EDGE_CURVE('',#13315,#13314,#7907,.T.);
#17012=EDGE_CURVE('',#13232,#13315,#7908,.T.);
#17013=EDGE_CURVE('',#13316,#13315,#7909,.T.);
#17014=EDGE_CURVE('',#13233,#13316,#7910,.T.);
#17015=EDGE_CURVE('',#13317,#13316,#7911,.T.);
#17016=EDGE_CURVE('',#13234,#13317,#7912,.T.);
#17017=EDGE_CURVE('',#13318,#13317,#7913,.T.);
#17018=EDGE_CURVE('',#13235,#13318,#7914,.T.);
#17019=EDGE_CURVE('',#13319,#13318,#7915,.T.);
#17020=EDGE_CURVE('',#13236,#13319,#7916,.T.);
#17021=EDGE_CURVE('',#13320,#13319,#7917,.T.);
#17022=EDGE_CURVE('',#13237,#13320,#7918,.T.);
#17023=EDGE_CURVE('',#13321,#13320,#7919,.T.);
#17024=EDGE_CURVE('',#13238,#13321,#7920,.T.);
#17025=EDGE_CURVE('',#13312,#13321,#7921,.T.);
#17026=EDGE_CURVE('',#13322,#13323,#1457,.T.);
#17027=EDGE_CURVE('',#13322,#13324,#7922,.T.);
#17028=EDGE_CURVE('',#13325,#13324,#1458,.T.);
#17029=EDGE_CURVE('',#13323,#13325,#7923,.T.);
#17030=EDGE_CURVE('',#13323,#13326,#1459,.T.);
#17031=EDGE_CURVE('',#13327,#13325,#1460,.T.);
#17032=EDGE_CURVE('',#13326,#13327,#7924,.T.);
#17033=EDGE_CURVE('',#13326,#13328,#1461,.T.);
#17034=EDGE_CURVE('',#13329,#13327,#1462,.T.);
#17035=EDGE_CURVE('',#13328,#13329,#7925,.T.);
#17036=EDGE_CURVE('',#13328,#13330,#1463,.T.);
#17037=EDGE_CURVE('',#13331,#13329,#1464,.T.);
#17038=EDGE_CURVE('',#13330,#13331,#7926,.T.);
#17039=EDGE_CURVE('',#13330,#13332,#1465,.T.);
#17040=EDGE_CURVE('',#13333,#13331,#1466,.T.);
#17041=EDGE_CURVE('',#13332,#13333,#7927,.T.);
#17042=EDGE_CURVE('',#13332,#13334,#1467,.T.);
#17043=EDGE_CURVE('',#13335,#13333,#1468,.T.);
#17044=EDGE_CURVE('',#13334,#13335,#7928,.T.);
#17045=EDGE_CURVE('',#13334,#13336,#1469,.T.);
#17046=EDGE_CURVE('',#13337,#13335,#1470,.T.);
#17047=EDGE_CURVE('',#13336,#13337,#7929,.T.);
#17048=EDGE_CURVE('',#13336,#13322,#1471,.T.);
#17049=EDGE_CURVE('',#13324,#13337,#1472,.T.);
#17050=EDGE_CURVE('',#13214,#13338,#7930,.T.);
#17051=EDGE_CURVE('',#13339,#13338,#1473,.T.);
#17052=EDGE_CURVE('',#13215,#13339,#7931,.T.);
#17053=EDGE_CURVE('',#13340,#13339,#1474,.T.);
#17054=EDGE_CURVE('',#13216,#13340,#7932,.T.);
#17055=EDGE_CURVE('',#13341,#13340,#1475,.T.);
#17056=EDGE_CURVE('',#13217,#13341,#7933,.T.);
#17057=EDGE_CURVE('',#13342,#13341,#1476,.T.);
#17058=EDGE_CURVE('',#13218,#13342,#7934,.T.);
#17059=EDGE_CURVE('',#13343,#13342,#1477,.T.);
#17060=EDGE_CURVE('',#13219,#13343,#7935,.T.);
#17061=EDGE_CURVE('',#13344,#13343,#1478,.T.);
#17062=EDGE_CURVE('',#13220,#13344,#7936,.T.);
#17063=EDGE_CURVE('',#13345,#13344,#1479,.T.);
#17064=EDGE_CURVE('',#13221,#13345,#7937,.T.);
#17065=EDGE_CURVE('',#13346,#13345,#1480,.T.);
#17066=EDGE_CURVE('',#13222,#13346,#7938,.T.);
#17067=EDGE_CURVE('',#13347,#13346,#1481,.T.);
#17068=EDGE_CURVE('',#13223,#13347,#7939,.T.);
#17069=EDGE_CURVE('',#13338,#13347,#1482,.T.);
#17070=EDGE_CURVE('',#13224,#13348,#7940,.T.);
#17071=EDGE_CURVE('',#13349,#13348,#7941,.T.);
#17072=EDGE_CURVE('',#13225,#13349,#7942,.T.);
#17073=EDGE_CURVE('',#13350,#13349,#7943,.T.);
#17074=EDGE_CURVE('',#13226,#13350,#7944,.T.);
#17075=EDGE_CURVE('',#13351,#13350,#7945,.T.);
#17076=EDGE_CURVE('',#13227,#13351,#7946,.T.);
#17077=EDGE_CURVE('',#13348,#13351,#7947,.T.);
#17078=EDGE_CURVE('',#13352,#13352,#11106,.T.);
#17079=EDGE_CURVE('',#13352,#13170,#7948,.T.);
#17080=EDGE_CURVE('',#13353,#13353,#11107,.T.);
#17081=EDGE_CURVE('',#13353,#13168,#7949,.T.);
#17082=EDGE_CURVE('',#13018,#13169,#7950,.T.);
#17083=EDGE_CURVE('',#13014,#13167,#7951,.T.);
#17084=EDGE_CURVE('',#12991,#13009,#7952,.T.);
#17085=EDGE_CURVE('',#12987,#13008,#7953,.T.);
#17086=EDGE_CURVE('',#12967,#13354,#7954,.T.);
#17087=EDGE_CURVE('',#12995,#13354,#7955,.T.);
#17088=EDGE_CURVE('',#13354,#12971,#7956,.T.);
#17089=EDGE_CURVE('',#13280,#12946,#7957,.T.);
#17090=EDGE_CURVE('',#13179,#12946,#7958,.F.);
#17091=EDGE_CURVE('',#13355,#13136,#7959,.T.);
#17092=EDGE_CURVE('',#12936,#13355,#7960,.T.);
#17093=EDGE_CURVE('',#12947,#13355,#7961,.T.);
#17094=EDGE_CURVE('',#13355,#13288,#7962,.T.);
#17095=EDGE_CURVE('',#13356,#13356,#11108,.T.);
#17096=EDGE_CURVE('',#13356,#12952,#7963,.T.);
#17097=EDGE_CURVE('',#13357,#13357,#11109,.T.);
#17098=EDGE_CURVE('',#13358,#13358,#11110,.T.);
#17099=EDGE_CURVE('',#13358,#12951,#7964,.T.);
#17100=EDGE_CURVE('',#13359,#13359,#11111,.T.);
#17101=EDGE_CURVE('',#13228,#13360,#7965,.T.);
#17102=EDGE_CURVE('',#13360,#13360,#11112,.T.);
#17103=EDGE_CURVE('',#13360,#13361,#7966,.T.);
#17104=EDGE_CURVE('',#13361,#13361,#11113,.T.);
#17105=EDGE_CURVE('',#13359,#13361,#7967,.T.);
#17106=EDGE_CURVE('',#13262,#13362,#7968,.T.);
#17107=EDGE_CURVE('',#13362,#13362,#11114,.T.);
#17108=EDGE_CURVE('',#13363,#13363,#11115,.T.);
#17109=EDGE_CURVE('',#13363,#13362,#7969,.T.);
#17110=EDGE_CURVE('',#13357,#13363,#7970,.T.);
#17111=EDGE_CURVE('',#13210,#13364,#133,.T.);
#17112=EDGE_CURVE('',#13364,#13274,#7971,.T.);
#17113=EDGE_CURVE('',#13282,#13211,#7972,.T.);
#17114=EDGE_CURVE('',#13283,#13212,#7973,.T.);
#17115=EDGE_CURVE('',#13289,#13213,#7974,.T.);
#17116=EDGE_CURVE('',#13283,#13289,#11116,.T.);
#17117=EDGE_CURVE('',#13105,#13205,#7975,.T.);
#17118=EDGE_CURVE('',#13128,#13206,#7976,.T.);
#17119=EDGE_CURVE('',#13296,#13209,#7977,.T.);
#17120=EDGE_CURVE('',#13299,#13365,#261,.F.);
#17121=EDGE_CURVE('',#13364,#13365,#262,.T.);
#17122=EDGE_CURVE('',#13293,#13285,#11117,.T.);
#17123=EDGE_CURVE('',#13176,#13268,#134,.T.);
#17124=EDGE_CURVE('',#13154,#13254,#7978,.T.);
#17125=EDGE_CURVE('',#13278,#13255,#7979,.T.);
#17126=EDGE_CURVE('',#13293,#13260,#7980,.T.);
#17127=EDGE_CURVE('',#13285,#13261,#7981,.T.);
#17128=EDGE_CURVE('',#12998,#13366,#7982,.T.);
#17129=EDGE_CURVE('',#13366,#13367,#7983,.T.);
#17130=EDGE_CURVE('',#13367,#12999,#7984,.T.);
#17131=EDGE_CURVE('',#12997,#13368,#7985,.T.);
#17132=EDGE_CURVE('',#13368,#13366,#11118,.T.);
#17133=EDGE_CURVE('',#12996,#13369,#7986,.T.);
#17134=EDGE_CURVE('',#13369,#13368,#7987,.T.);
#17135=EDGE_CURVE('',#13354,#13369,#11119,.T.);
#17136=EDGE_CURVE('',#13001,#13370,#7988,.T.);
#17137=EDGE_CURVE('',#13370,#12964,#11120,.T.);
#17138=EDGE_CURVE('',#13000,#13371,#7989,.T.);
#17139=EDGE_CURVE('',#13371,#13370,#7990,.T.);
#17140=EDGE_CURVE('',#13367,#13371,#11121,.T.);
#17141=EDGE_CURVE('',#13370,#13372,#7991,.T.);
#17142=EDGE_CURVE('',#12962,#13372,#11122,.T.);
#17143=EDGE_CURVE('',#13373,#13371,#7992,.T.);
#17144=EDGE_CURVE('',#13372,#13373,#7993,.T.);
#17145=EDGE_CURVE('',#13367,#13374,#7994,.T.);
#17146=EDGE_CURVE('',#13373,#13374,#11123,.T.);
#17147=EDGE_CURVE('',#13375,#13366,#7995,.T.);
#17148=EDGE_CURVE('',#13374,#13375,#7996,.T.);
#17149=EDGE_CURVE('',#13372,#13161,#7997,.T.);
#17150=EDGE_CURVE('',#13166,#13376,#7998,.T.);
#17151=EDGE_CURVE('',#13376,#12971,#11124,.T.);
#17152=EDGE_CURVE('',#13165,#13377,#7999,.T.);
#17153=EDGE_CURVE('',#13377,#13376,#8000,.T.);
#17154=EDGE_CURVE('',#13164,#13375,#8001,.T.);
#17155=EDGE_CURVE('',#13375,#13377,#11125,.T.);
#17156=EDGE_CURVE('',#13163,#13374,#8002,.T.);
#17157=EDGE_CURVE('',#13162,#13373,#8003,.T.);
#17158=EDGE_CURVE('',#13368,#13377,#8004,.T.);
#17159=EDGE_CURVE('',#13376,#13369,#8005,.T.);
#23168=ORIENTED_EDGE('',*,*,#16437,.T.);
#23169=ORIENTED_EDGE('',*,*,#16438,.T.);
#23170=ORIENTED_EDGE('',*,*,#16439,.T.);
#23171=ORIENTED_EDGE('',*,*,#16440,.T.);
#23172=ORIENTED_EDGE('',*,*,#16441,.T.);
#23173=ORIENTED_EDGE('',*,*,#16442,.T.);
#23174=ORIENTED_EDGE('',*,*,#16443,.T.);
#23175=ORIENTED_EDGE('',*,*,#16439,.F.);
#23176=ORIENTED_EDGE('',*,*,#16444,.T.);
#23177=ORIENTED_EDGE('',*,*,#16445,.T.);
#23178=ORIENTED_EDGE('',*,*,#16446,.T.);
#23179=ORIENTED_EDGE('',*,*,#16447,.T.);
#23180=ORIENTED_EDGE('',*,*,#16441,.F.);
#23181=ORIENTED_EDGE('',*,*,#16448,.T.);
#23182=ORIENTED_EDGE('',*,*,#16449,.T.);
#23183=ORIENTED_EDGE('',*,*,#16450,.T.);
#23184=ORIENTED_EDGE('',*,*,#16451,.T.);
#23185=ORIENTED_EDGE('',*,*,#16452,.T.);
#23186=ORIENTED_EDGE('',*,*,#16453,.T.);
#23187=ORIENTED_EDGE('',*,*,#16451,.F.);
#23188=ORIENTED_EDGE('',*,*,#16454,.T.);
#23189=ORIENTED_EDGE('',*,*,#16445,.F.);
#23190=ORIENTED_EDGE('',*,*,#16449,.F.);
#23191=ORIENTED_EDGE('',*,*,#16455,.F.);
#23192=ORIENTED_EDGE('',*,*,#16456,.F.);
#23193=ORIENTED_EDGE('',*,*,#16457,.T.);
#23194=ORIENTED_EDGE('',*,*,#16440,.F.);
#23195=ORIENTED_EDGE('',*,*,#16443,.F.);
#23196=ORIENTED_EDGE('',*,*,#16458,.T.);
#23197=ORIENTED_EDGE('',*,*,#16459,.F.);
#23198=ORIENTED_EDGE('',*,*,#16460,.F.);
#23199=ORIENTED_EDGE('',*,*,#16461,.F.);
#23200=ORIENTED_EDGE('',*,*,#16462,.F.);
#23201=ORIENTED_EDGE('',*,*,#16455,.T.);
#23202=ORIENTED_EDGE('',*,*,#16448,.F.);
#23203=ORIENTED_EDGE('',*,*,#16463,.F.);
#23204=ORIENTED_EDGE('',*,*,#16464,.T.);
#23205=ORIENTED_EDGE('',*,*,#16452,.F.);
#23206=ORIENTED_EDGE('',*,*,#16444,.F.);
#23207=ORIENTED_EDGE('',*,*,#16438,.F.);
#23208=ORIENTED_EDGE('',*,*,#16465,.T.);
#23209=ORIENTED_EDGE('',*,*,#16466,.F.);
#23210=ORIENTED_EDGE('',*,*,#16465,.F.);
#23211=ORIENTED_EDGE('',*,*,#16437,.F.);
#23212=ORIENTED_EDGE('',*,*,#16447,.F.);
#23213=ORIENTED_EDGE('',*,*,#16453,.F.);
#23214=ORIENTED_EDGE('',*,*,#16464,.F.);
#23215=ORIENTED_EDGE('',*,*,#16467,.T.);
#23216=ORIENTED_EDGE('',*,*,#16468,.T.);
#23217=ORIENTED_EDGE('',*,*,#16469,.T.);
#23218=ORIENTED_EDGE('',*,*,#16470,.T.);
#23219=ORIENTED_EDGE('',*,*,#16471,.T.);
#23220=ORIENTED_EDGE('',*,*,#16470,.F.);
#23221=ORIENTED_EDGE('',*,*,#16472,.F.);
#23222=ORIENTED_EDGE('',*,*,#16473,.T.);
#23223=ORIENTED_EDGE('',*,*,#16474,.F.);
#23224=ORIENTED_EDGE('',*,*,#16475,.F.);
#23225=ORIENTED_EDGE('',*,*,#16476,.F.);
#23226=ORIENTED_EDGE('',*,*,#16469,.F.);
#23227=ORIENTED_EDGE('',*,*,#16477,.T.);
#23228=ORIENTED_EDGE('',*,*,#16478,.F.);
#23229=ORIENTED_EDGE('',*,*,#16479,.T.);
#23230=ORIENTED_EDGE('',*,*,#16468,.F.);
#23231=ORIENTED_EDGE('',*,*,#16480,.F.);
#23232=ORIENTED_EDGE('',*,*,#16481,.F.);
#23233=ORIENTED_EDGE('',*,*,#16477,.F.);
#23234=ORIENTED_EDGE('',*,*,#16482,.T.);
#23235=ORIENTED_EDGE('',*,*,#16483,.T.);
#23236=ORIENTED_EDGE('',*,*,#16484,.T.);
#23237=ORIENTED_EDGE('',*,*,#16485,.T.);
#23238=ORIENTED_EDGE('',*,*,#16486,.T.);
#23239=ORIENTED_EDGE('',*,*,#16482,.F.);
#23240=ORIENTED_EDGE('',*,*,#16487,.T.);
#23241=ORIENTED_EDGE('',*,*,#16488,.T.);
#23242=ORIENTED_EDGE('',*,*,#16489,.T.);
#23243=ORIENTED_EDGE('',*,*,#16486,.F.);
#23244=ORIENTED_EDGE('',*,*,#16490,.F.);
#23245=ORIENTED_EDGE('',*,*,#16491,.F.);
#23246=ORIENTED_EDGE('',*,*,#16492,.F.);
#23247=ORIENTED_EDGE('',*,*,#16493,.F.);
#23248=ORIENTED_EDGE('',*,*,#16494,.F.);
#23249=ORIENTED_EDGE('',*,*,#16485,.F.);
#23250=ORIENTED_EDGE('',*,*,#16495,.T.);
#23251=ORIENTED_EDGE('',*,*,#16496,.T.);
#23252=ORIENTED_EDGE('',*,*,#16497,.T.);
#23253=ORIENTED_EDGE('',*,*,#16490,.T.);
#23254=ORIENTED_EDGE('',*,*,#16498,.F.);
#23255=ORIENTED_EDGE('',*,*,#16499,.F.);
#23256=ORIENTED_EDGE('',*,*,#16500,.F.);
#23257=ORIENTED_EDGE('',*,*,#16501,.T.);
#23258=ORIENTED_EDGE('',*,*,#16499,.T.);
#23259=ORIENTED_EDGE('',*,*,#16475,.T.);
#23260=ORIENTED_EDGE('',*,*,#16502,.T.);
#23261=ORIENTED_EDGE('',*,*,#16503,.F.);
#23262=ORIENTED_EDGE('',*,*,#16497,.F.);
#23263=ORIENTED_EDGE('',*,*,#16504,.F.);
#23264=ORIENTED_EDGE('',*,*,#16505,.T.);
#23265=ORIENTED_EDGE('',*,*,#16506,.T.);
#23266=ORIENTED_EDGE('',*,*,#16507,.T.);
#23267=ORIENTED_EDGE('',*,*,#16508,.T.);
#23268=ORIENTED_EDGE('',*,*,#16509,.T.);
#23269=ORIENTED_EDGE('',*,*,#16504,.T.);
#23270=ORIENTED_EDGE('',*,*,#16510,.T.);
#23271=ORIENTED_EDGE('',*,*,#16506,.F.);
#23272=ORIENTED_EDGE('',*,*,#16491,.T.);
#23273=ORIENTED_EDGE('',*,*,#16503,.T.);
#23274=ORIENTED_EDGE('',*,*,#16511,.T.);
#23275=ORIENTED_EDGE('',*,*,#16512,.T.);
#23276=ORIENTED_EDGE('',*,*,#16513,.T.);
#23277=ORIENTED_EDGE('',*,*,#16508,.F.);
#23278=ORIENTED_EDGE('',*,*,#16514,.T.);
#23279=ORIENTED_EDGE('',*,*,#16515,.T.);
#23280=ORIENTED_EDGE('',*,*,#16516,.T.);
#23281=ORIENTED_EDGE('',*,*,#16517,.T.);
#23282=ORIENTED_EDGE('',*,*,#16492,.T.);
#23283=ORIENTED_EDGE('',*,*,#16512,.F.);
#23284=ORIENTED_EDGE('',*,*,#16518,.T.);
#23285=ORIENTED_EDGE('',*,*,#16519,.T.);
#23286=ORIENTED_EDGE('',*,*,#16517,.F.);
#23287=ORIENTED_EDGE('',*,*,#16520,.T.);
#23288=ORIENTED_EDGE('',*,*,#16474,.T.);
#23289=ORIENTED_EDGE('',*,*,#16518,.F.);
#23290=ORIENTED_EDGE('',*,*,#16521,.T.);
#23291=ORIENTED_EDGE('',*,*,#16502,.F.);
#23292=ORIENTED_EDGE('',*,*,#16522,.T.);
#23293=ORIENTED_EDGE('',*,*,#16515,.F.);
#23294=ORIENTED_EDGE('',*,*,#16523,.T.);
#23295=ORIENTED_EDGE('',*,*,#16524,.T.);
#23296=ORIENTED_EDGE('',*,*,#16525,.T.);
#23297=ORIENTED_EDGE('',*,*,#16500,.T.);
#23298=ORIENTED_EDGE('',*,*,#16526,.T.);
#23299=ORIENTED_EDGE('',*,*,#16524,.F.);
#23300=ORIENTED_EDGE('',*,*,#16471,.F.);
#23301=ORIENTED_EDGE('',*,*,#16476,.T.);
#23302=ORIENTED_EDGE('',*,*,#16498,.T.);
#23303=ORIENTED_EDGE('',*,*,#16527,.T.);
#23304=ORIENTED_EDGE('',*,*,#16528,.T.);
#23305=ORIENTED_EDGE('',*,*,#16467,.F.);
#23306=ORIENTED_EDGE('',*,*,#16528,.F.);
#23307=ORIENTED_EDGE('',*,*,#16529,.T.);
#23308=ORIENTED_EDGE('',*,*,#16530,.T.);
#23309=ORIENTED_EDGE('',*,*,#16480,.T.);
#23310=ORIENTED_EDGE('',*,*,#16527,.F.);
#23311=ORIENTED_EDGE('',*,*,#16525,.F.);
#23312=ORIENTED_EDGE('',*,*,#16523,.F.);
#23313=ORIENTED_EDGE('',*,*,#16514,.F.);
#23314=ORIENTED_EDGE('',*,*,#16507,.F.);
#23315=ORIENTED_EDGE('',*,*,#16510,.F.);
#23316=ORIENTED_EDGE('',*,*,#16496,.F.);
#23317=ORIENTED_EDGE('',*,*,#16531,.F.);
#23318=ORIENTED_EDGE('',*,*,#16532,.F.);
#23319=ORIENTED_EDGE('',*,*,#16533,.F.);
#23320=ORIENTED_EDGE('',*,*,#16534,.F.);
#23321=ORIENTED_EDGE('',*,*,#16535,.F.);
#23322=ORIENTED_EDGE('',*,*,#16536,.F.);
#23323=ORIENTED_EDGE('',*,*,#16537,.F.);
#23324=ORIENTED_EDGE('',*,*,#16538,.F.);
#23325=ORIENTED_EDGE('',*,*,#16529,.F.);
#23326=ORIENTED_EDGE('',*,*,#16539,.F.);
#23327=ORIENTED_EDGE('',*,*,#16540,.F.);
#23328=ORIENTED_EDGE('',*,*,#16541,.F.);
#23329=ORIENTED_EDGE('',*,*,#16542,.F.);
#23330=ORIENTED_EDGE('',*,*,#16521,.F.);
#23331=ORIENTED_EDGE('',*,*,#16520,.F.);
#23332=ORIENTED_EDGE('',*,*,#16516,.F.);
#23333=ORIENTED_EDGE('',*,*,#16543,.F.);
#23334=ORIENTED_EDGE('',*,*,#16544,.F.);
#23335=ORIENTED_EDGE('',*,*,#16545,.F.);
#23336=ORIENTED_EDGE('',*,*,#16546,.F.);
#23337=ORIENTED_EDGE('',*,*,#16547,.F.);
#23338=ORIENTED_EDGE('',*,*,#16548,.F.);
#23339=ORIENTED_EDGE('',*,*,#16511,.F.);
#23340=ORIENTED_EDGE('',*,*,#16509,.F.);
#23341=ORIENTED_EDGE('',*,*,#16549,.T.);
#23342=ORIENTED_EDGE('',*,*,#16543,.T.);
#23343=ORIENTED_EDGE('',*,*,#16505,.F.);
#23344=ORIENTED_EDGE('',*,*,#16550,.T.);
#23345=ORIENTED_EDGE('',*,*,#16544,.T.);
#23346=ORIENTED_EDGE('',*,*,#16549,.F.);
#23347=ORIENTED_EDGE('',*,*,#16551,.T.);
#23348=ORIENTED_EDGE('',*,*,#16552,.T.);
#23349=ORIENTED_EDGE('',*,*,#16553,.T.);
#23350=ORIENTED_EDGE('',*,*,#16552,.F.);
#23351=ORIENTED_EDGE('',*,*,#16554,.F.);
#23352=ORIENTED_EDGE('',*,*,#16555,.T.);
#23353=ORIENTED_EDGE('',*,*,#16551,.F.);
#23354=ORIENTED_EDGE('',*,*,#16555,.F.);
#23355=ORIENTED_EDGE('',*,*,#16556,.T.);
#23356=ORIENTED_EDGE('',*,*,#16553,.F.);
#23357=ORIENTED_EDGE('',*,*,#16539,.T.);
#23358=ORIENTED_EDGE('',*,*,#16557,.T.);
#23359=ORIENTED_EDGE('',*,*,#16554,.T.);
#23360=ORIENTED_EDGE('',*,*,#16557,.F.);
#23361=ORIENTED_EDGE('',*,*,#16558,.T.);
#23362=ORIENTED_EDGE('',*,*,#16559,.T.);
#23363=ORIENTED_EDGE('',*,*,#16560,.T.);
#23364=ORIENTED_EDGE('',*,*,#16559,.F.);
#23365=ORIENTED_EDGE('',*,*,#16561,.F.);
#23366=ORIENTED_EDGE('',*,*,#16562,.T.);
#23367=ORIENTED_EDGE('',*,*,#16558,.F.);
#23368=ORIENTED_EDGE('',*,*,#16562,.F.);
#23369=ORIENTED_EDGE('',*,*,#16563,.T.);
#23370=ORIENTED_EDGE('',*,*,#16560,.F.);
#23371=ORIENTED_EDGE('',*,*,#16542,.T.);
#23372=ORIENTED_EDGE('',*,*,#16564,.T.);
#23373=ORIENTED_EDGE('',*,*,#16561,.T.);
#23374=ORIENTED_EDGE('',*,*,#16564,.F.);
#23375=ORIENTED_EDGE('',*,*,#16540,.T.);
#23376=ORIENTED_EDGE('',*,*,#16565,.T.);
#23377=ORIENTED_EDGE('',*,*,#16566,.T.);
#23378=ORIENTED_EDGE('',*,*,#16565,.F.);
#23379=ORIENTED_EDGE('',*,*,#16566,.F.);
#23380=ORIENTED_EDGE('',*,*,#16567,.T.);
#23381=ORIENTED_EDGE('',*,*,#16568,.T.);
#23382=ORIENTED_EDGE('',*,*,#16567,.F.);
#23383=ORIENTED_EDGE('',*,*,#16541,.T.);
#23384=ORIENTED_EDGE('',*,*,#16569,.T.);
#23385=ORIENTED_EDGE('',*,*,#16570,.T.);
#23386=ORIENTED_EDGE('',*,*,#16569,.F.);
#23387=ORIENTED_EDGE('',*,*,#16570,.F.);
#23388=ORIENTED_EDGE('',*,*,#16571,.T.);
#23389=ORIENTED_EDGE('',*,*,#16572,.T.);
#23390=ORIENTED_EDGE('',*,*,#16571,.F.);
#23391=ORIENTED_EDGE('',*,*,#16573,.F.);
#23392=ORIENTED_EDGE('',*,*,#16574,.F.);
#23393=ORIENTED_EDGE('',*,*,#16575,.F.);
#23394=ORIENTED_EDGE('',*,*,#16576,.F.);
#23395=ORIENTED_EDGE('',*,*,#16577,.F.);
#23396=ORIENTED_EDGE('',*,*,#16578,.F.);
#23397=ORIENTED_EDGE('',*,*,#16574,.T.);
#23398=ORIENTED_EDGE('',*,*,#16579,.T.);
#23399=ORIENTED_EDGE('',*,*,#16577,.T.);
#23400=ORIENTED_EDGE('',*,*,#16580,.T.);
#23401=ORIENTED_EDGE('',*,*,#16581,.T.);
#23402=ORIENTED_EDGE('',*,*,#16582,.T.);
#23403=ORIENTED_EDGE('',*,*,#16578,.T.);
#23404=ORIENTED_EDGE('',*,*,#16583,.T.);
#23405=ORIENTED_EDGE('',*,*,#16584,.T.);
#23406=ORIENTED_EDGE('',*,*,#16585,.T.);
#23407=ORIENTED_EDGE('',*,*,#16576,.T.);
#23408=ORIENTED_EDGE('',*,*,#16586,.T.);
#23409=ORIENTED_EDGE('',*,*,#16587,.T.);
#23410=ORIENTED_EDGE('',*,*,#16588,.T.);
#23411=ORIENTED_EDGE('',*,*,#16575,.T.);
#23412=ORIENTED_EDGE('',*,*,#16589,.T.);
#23413=ORIENTED_EDGE('',*,*,#16590,.T.);
#23414=ORIENTED_EDGE('',*,*,#16591,.T.);
#23415=ORIENTED_EDGE('',*,*,#16573,.T.);
#23416=ORIENTED_EDGE('',*,*,#16592,.T.);
#23417=ORIENTED_EDGE('',*,*,#16586,.F.);
#23418=ORIENTED_EDGE('',*,*,#16582,.F.);
#23419=ORIENTED_EDGE('',*,*,#16593,.F.);
#23420=ORIENTED_EDGE('',*,*,#16594,.F.);
#23421=ORIENTED_EDGE('',*,*,#16595,.T.);
#23422=ORIENTED_EDGE('',*,*,#16596,.T.);
#23423=ORIENTED_EDGE('',*,*,#16597,.F.);
#23424=ORIENTED_EDGE('',*,*,#16583,.F.);
#23425=ORIENTED_EDGE('',*,*,#16579,.F.);
#23426=ORIENTED_EDGE('',*,*,#16591,.F.);
#23427=ORIENTED_EDGE('',*,*,#16598,.F.);
#23428=ORIENTED_EDGE('',*,*,#16599,.T.);
#23429=ORIENTED_EDGE('',*,*,#16600,.F.);
#23430=ORIENTED_EDGE('',*,*,#16601,.T.);
#23431=ORIENTED_EDGE('',*,*,#16602,.T.);
#23432=ORIENTED_EDGE('',*,*,#16603,.T.);
#23433=ORIENTED_EDGE('',*,*,#16604,.T.);
#23434=ORIENTED_EDGE('',*,*,#16605,.T.);
#23435=ORIENTED_EDGE('',*,*,#16606,.T.);
#23436=ORIENTED_EDGE('',*,*,#16607,.T.);
#23437=ORIENTED_EDGE('',*,*,#16608,.F.);
#23438=ORIENTED_EDGE('',*,*,#16609,.T.);
#23439=ORIENTED_EDGE('',*,*,#16610,.T.);
#23440=ORIENTED_EDGE('',*,*,#16611,.T.);
#23441=ORIENTED_EDGE('',*,*,#16610,.F.);
#23442=ORIENTED_EDGE('',*,*,#16612,.T.);
#23443=ORIENTED_EDGE('',*,*,#16604,.F.);
#23444=ORIENTED_EDGE('',*,*,#16602,.F.);
#23445=ORIENTED_EDGE('',*,*,#16613,.F.);
#23446=ORIENTED_EDGE('',*,*,#16614,.F.);
#23447=ORIENTED_EDGE('',*,*,#16615,.F.);
#23448=ORIENTED_EDGE('',*,*,#16616,.F.);
#23449=ORIENTED_EDGE('',*,*,#16617,.F.);
#23450=ORIENTED_EDGE('',*,*,#16618,.F.);
#23451=ORIENTED_EDGE('',*,*,#16619,.F.);
#23452=ORIENTED_EDGE('',*,*,#16620,.F.);
#23453=ORIENTED_EDGE('',*,*,#16621,.F.);
#23454=ORIENTED_EDGE('',*,*,#16622,.T.);
#23455=ORIENTED_EDGE('',*,*,#16605,.F.);
#23456=ORIENTED_EDGE('',*,*,#16623,.F.);
#23457=ORIENTED_EDGE('',*,*,#16624,.F.);
#23458=ORIENTED_EDGE('',*,*,#16625,.T.);
#23459=ORIENTED_EDGE('',*,*,#16626,.T.);
#23460=ORIENTED_EDGE('',*,*,#16613,.T.);
#23461=ORIENTED_EDGE('',*,*,#16612,.F.);
#23462=ORIENTED_EDGE('',*,*,#16627,.T.);
#23463=ORIENTED_EDGE('',*,*,#16628,.T.);
#23464=ORIENTED_EDGE('',*,*,#16623,.T.);
#23465=ORIENTED_EDGE('',*,*,#16609,.F.);
#23466=ORIENTED_EDGE('',*,*,#16629,.F.);
#23467=ORIENTED_EDGE('',*,*,#16630,.F.);
#23468=ORIENTED_EDGE('',*,*,#16631,.F.);
#23469=ORIENTED_EDGE('',*,*,#16632,.F.);
#23470=ORIENTED_EDGE('',*,*,#16633,.F.);
#23471=ORIENTED_EDGE('',*,*,#16634,.F.);
#23472=ORIENTED_EDGE('',*,*,#16627,.F.);
#23473=ORIENTED_EDGE('',*,*,#16635,.F.);
#23474=ORIENTED_EDGE('',*,*,#16636,.F.);
#23475=ORIENTED_EDGE('',*,*,#16637,.T.);
#23476=ORIENTED_EDGE('',*,*,#16638,.F.);
#23477=ORIENTED_EDGE('',*,*,#16639,.F.);
#23478=ORIENTED_EDGE('',*,*,#16640,.T.);
#23479=ORIENTED_EDGE('',*,*,#16641,.T.);
#23480=ORIENTED_EDGE('',*,*,#16632,.T.);
#23481=ORIENTED_EDGE('',*,*,#16642,.T.);
#23482=ORIENTED_EDGE('',*,*,#16643,.F.);
#23483=ORIENTED_EDGE('',*,*,#16644,.T.);
#23484=ORIENTED_EDGE('',*,*,#16645,.T.);
#23485=ORIENTED_EDGE('',*,*,#16646,.T.);
#23486=ORIENTED_EDGE('',*,*,#16647,.T.);
#23487=ORIENTED_EDGE('',*,*,#16646,.F.);
#23488=ORIENTED_EDGE('',*,*,#16648,.T.);
#23489=ORIENTED_EDGE('',*,*,#16641,.F.);
#23490=ORIENTED_EDGE('',*,*,#16648,.F.);
#23491=ORIENTED_EDGE('',*,*,#16649,.T.);
#23492=ORIENTED_EDGE('',*,*,#16650,.F.);
#23493=ORIENTED_EDGE('',*,*,#16633,.T.);
#23494=ORIENTED_EDGE('',*,*,#16645,.F.);
#23495=ORIENTED_EDGE('',*,*,#16651,.T.);
#23496=ORIENTED_EDGE('',*,*,#16652,.T.);
#23497=ORIENTED_EDGE('',*,*,#16653,.T.);
#23498=ORIENTED_EDGE('',*,*,#16654,.F.);
#23499=ORIENTED_EDGE('',*,*,#16649,.F.);
#23500=ORIENTED_EDGE('',*,*,#16644,.F.);
#23501=ORIENTED_EDGE('',*,*,#16655,.T.);
#23502=ORIENTED_EDGE('',*,*,#16656,.F.);
#23503=ORIENTED_EDGE('',*,*,#16657,.F.);
#23504=ORIENTED_EDGE('',*,*,#16658,.F.);
#23505=ORIENTED_EDGE('',*,*,#16659,.F.);
#23506=ORIENTED_EDGE('',*,*,#16660,.F.);
#23507=ORIENTED_EDGE('',*,*,#16661,.F.);
#23508=ORIENTED_EDGE('',*,*,#16662,.F.);
#23509=ORIENTED_EDGE('',*,*,#16663,.F.);
#23510=ORIENTED_EDGE('',*,*,#16651,.F.);
#23511=ORIENTED_EDGE('',*,*,#16664,.T.);
#23512=ORIENTED_EDGE('',*,*,#16665,.T.);
#23513=ORIENTED_EDGE('',*,*,#16666,.T.);
#23514=ORIENTED_EDGE('',*,*,#16638,.T.);
#23515=ORIENTED_EDGE('',*,*,#16665,.F.);
#23516=ORIENTED_EDGE('',*,*,#16667,.F.);
#23517=ORIENTED_EDGE('',*,*,#16668,.F.);
#23518=ORIENTED_EDGE('',*,*,#16669,.F.);
#23519=ORIENTED_EDGE('',*,*,#16670,.T.);
#23520=ORIENTED_EDGE('',*,*,#16671,.F.);
#23521=ORIENTED_EDGE('',*,*,#16672,.T.);
#23522=ORIENTED_EDGE('',*,*,#16673,.T.);
#23523=ORIENTED_EDGE('',*,*,#16674,.T.);
#23524=ORIENTED_EDGE('',*,*,#16675,.T.);
#23525=ORIENTED_EDGE('',*,*,#16673,.F.);
#23526=ORIENTED_EDGE('',*,*,#16676,.F.);
#23527=ORIENTED_EDGE('',*,*,#16677,.F.);
#23528=ORIENTED_EDGE('',*,*,#16678,.F.);
#23529=ORIENTED_EDGE('',*,*,#16679,.F.);
#23530=ORIENTED_EDGE('',*,*,#16680,.F.);
#23531=ORIENTED_EDGE('',*,*,#16630,.T.);
#23532=ORIENTED_EDGE('',*,*,#16681,.F.);
#23533=ORIENTED_EDGE('',*,*,#16682,.F.);
#23534=ORIENTED_EDGE('',*,*,#16683,.F.);
#23535=ORIENTED_EDGE('',*,*,#16684,.F.);
#23536=ORIENTED_EDGE('',*,*,#16685,.F.);
#23537=ORIENTED_EDGE('',*,*,#16686,.F.);
#23538=ORIENTED_EDGE('',*,*,#16687,.F.);
#23539=ORIENTED_EDGE('',*,*,#16672,.F.);
#23540=ORIENTED_EDGE('',*,*,#16688,.F.);
#23541=ORIENTED_EDGE('',*,*,#16689,.T.);
#23542=ORIENTED_EDGE('',*,*,#16674,.F.);
#23543=ORIENTED_EDGE('',*,*,#16675,.F.);
#23544=ORIENTED_EDGE('',*,*,#16689,.F.);
#23545=ORIENTED_EDGE('',*,*,#16686,.T.);
#23546=ORIENTED_EDGE('',*,*,#16690,.T.);
#23547=ORIENTED_EDGE('',*,*,#16691,.T.);
#23548=ORIENTED_EDGE('',*,*,#16692,.T.);
#23549=ORIENTED_EDGE('',*,*,#16690,.F.);
#23550=ORIENTED_EDGE('',*,*,#16693,.F.);
#23551=ORIENTED_EDGE('',*,*,#16694,.T.);
#23552=ORIENTED_EDGE('',*,*,#16691,.F.);
#23553=ORIENTED_EDGE('',*,*,#16692,.F.);
#23554=ORIENTED_EDGE('',*,*,#16694,.F.);
#23555=ORIENTED_EDGE('',*,*,#16687,.T.);
#23556=ORIENTED_EDGE('',*,*,#16695,.T.);
#23557=ORIENTED_EDGE('',*,*,#16696,.T.);
#23558=ORIENTED_EDGE('',*,*,#16697,.T.);
#23559=ORIENTED_EDGE('',*,*,#16695,.F.);
#23560=ORIENTED_EDGE('',*,*,#16698,.F.);
#23561=ORIENTED_EDGE('',*,*,#16699,.T.);
#23562=ORIENTED_EDGE('',*,*,#16696,.F.);
#23563=ORIENTED_EDGE('',*,*,#16697,.F.);
#23564=ORIENTED_EDGE('',*,*,#16699,.F.);
#23565=ORIENTED_EDGE('',*,*,#16700,.T.);
#23566=ORIENTED_EDGE('',*,*,#16676,.T.);
#23567=ORIENTED_EDGE('',*,*,#16701,.T.);
#23568=ORIENTED_EDGE('',*,*,#16702,.T.);
#23569=ORIENTED_EDGE('',*,*,#16703,.T.);
#23570=ORIENTED_EDGE('',*,*,#16701,.F.);
#23571=ORIENTED_EDGE('',*,*,#16685,.T.);
#23572=ORIENTED_EDGE('',*,*,#16700,.F.);
#23573=ORIENTED_EDGE('',*,*,#16684,.T.);
#23574=ORIENTED_EDGE('',*,*,#16704,.F.);
#23575=ORIENTED_EDGE('',*,*,#16705,.F.);
#23576=ORIENTED_EDGE('',*,*,#16706,.F.);
#23577=ORIENTED_EDGE('',*,*,#16707,.F.);
#23578=ORIENTED_EDGE('',*,*,#16708,.F.);
#23579=ORIENTED_EDGE('',*,*,#16709,.F.);
#23580=ORIENTED_EDGE('',*,*,#16710,.F.);
#23581=ORIENTED_EDGE('',*,*,#16677,.T.);
#23582=ORIENTED_EDGE('',*,*,#16711,.F.);
#23583=ORIENTED_EDGE('',*,*,#16712,.T.);
#23584=ORIENTED_EDGE('',*,*,#16702,.F.);
#23585=ORIENTED_EDGE('',*,*,#16703,.F.);
#23586=ORIENTED_EDGE('',*,*,#16712,.F.);
#23587=ORIENTED_EDGE('',*,*,#16713,.F.);
#23588=ORIENTED_EDGE('',*,*,#16636,.T.);
#23589=ORIENTED_EDGE('',*,*,#16714,.T.);
#23590=ORIENTED_EDGE('',*,*,#16715,.T.);
#23591=ORIENTED_EDGE('',*,*,#16716,.T.);
#23592=ORIENTED_EDGE('',*,*,#16717,.F.);
#23593=ORIENTED_EDGE('',*,*,#16716,.F.);
#23594=ORIENTED_EDGE('',*,*,#16718,.F.);
#23595=ORIENTED_EDGE('',*,*,#16719,.T.);
#23596=ORIENTED_EDGE('',*,*,#16720,.F.);
#23597=ORIENTED_EDGE('',*,*,#16721,.F.);
#23598=ORIENTED_EDGE('',*,*,#16722,.F.);
#23599=ORIENTED_EDGE('',*,*,#16460,.T.);
#23600=ORIENTED_EDGE('',*,*,#16723,.T.);
#23601=ORIENTED_EDGE('',*,*,#16724,.T.);
#23602=ORIENTED_EDGE('',*,*,#16725,.T.);
#23603=ORIENTED_EDGE('',*,*,#16726,.F.);
#23604=ORIENTED_EDGE('',*,*,#16727,.F.);
#23605=ORIENTED_EDGE('',*,*,#16728,.F.);
#23606=ORIENTED_EDGE('',*,*,#16729,.F.);
#23607=ORIENTED_EDGE('',*,*,#16548,.T.);
#23608=ORIENTED_EDGE('',*,*,#16730,.T.);
#23609=ORIENTED_EDGE('',*,*,#16731,.T.);
#23610=ORIENTED_EDGE('',*,*,#16730,.F.);
#23611=ORIENTED_EDGE('',*,*,#16731,.F.);
#23612=ORIENTED_EDGE('',*,*,#16732,.T.);
#23613=ORIENTED_EDGE('',*,*,#16733,.F.);
#23614=ORIENTED_EDGE('',*,*,#16734,.F.);
#23615=ORIENTED_EDGE('',*,*,#16732,.F.);
#23616=ORIENTED_EDGE('',*,*,#16735,.T.);
#23617=ORIENTED_EDGE('',*,*,#16736,.T.);
#23618=ORIENTED_EDGE('',*,*,#16737,.T.);
#23619=ORIENTED_EDGE('',*,*,#16738,.T.);
#23620=ORIENTED_EDGE('',*,*,#16738,.F.);
#23621=ORIENTED_EDGE('',*,*,#16739,.F.);
#23622=ORIENTED_EDGE('',*,*,#16740,.F.);
#23623=ORIENTED_EDGE('',*,*,#16741,.F.);
#23624=ORIENTED_EDGE('',*,*,#16737,.F.);
#23625=ORIENTED_EDGE('',*,*,#16742,.F.);
#23626=ORIENTED_EDGE('',*,*,#16743,.F.);
#23627=ORIENTED_EDGE('',*,*,#16744,.F.);
#23628=ORIENTED_EDGE('',*,*,#16745,.T.);
#23629=ORIENTED_EDGE('',*,*,#16746,.T.);
#23630=ORIENTED_EDGE('',*,*,#16747,.T.);
#23631=ORIENTED_EDGE('',*,*,#16740,.T.);
#23632=ORIENTED_EDGE('',*,*,#16746,.F.);
#23633=ORIENTED_EDGE('',*,*,#16748,.T.);
#23634=ORIENTED_EDGE('',*,*,#16749,.T.);
#23635=ORIENTED_EDGE('',*,*,#16750,.T.);
#23636=ORIENTED_EDGE('',*,*,#16745,.F.);
#23637=ORIENTED_EDGE('',*,*,#16751,.F.);
#23638=ORIENTED_EDGE('',*,*,#16752,.F.);
#23639=ORIENTED_EDGE('',*,*,#16748,.F.);
#23640=ORIENTED_EDGE('',*,*,#16753,.T.);
#23641=ORIENTED_EDGE('',*,*,#16754,.T.);
#23642=ORIENTED_EDGE('',*,*,#16733,.T.);
#23643=ORIENTED_EDGE('',*,*,#16734,.T.);
#23644=ORIENTED_EDGE('',*,*,#16754,.F.);
#23645=ORIENTED_EDGE('',*,*,#16487,.F.);
#23646=ORIENTED_EDGE('',*,*,#16494,.T.);
#23647=ORIENTED_EDGE('',*,*,#16755,.T.);
#23648=ORIENTED_EDGE('',*,*,#16472,.T.);
#23649=ORIENTED_EDGE('',*,*,#16479,.F.);
#23650=ORIENTED_EDGE('',*,*,#16756,.F.);
#23651=ORIENTED_EDGE('',*,*,#16757,.F.);
#23652=ORIENTED_EDGE('',*,*,#16758,.F.);
#23653=ORIENTED_EDGE('',*,*,#16759,.F.);
#23654=ORIENTED_EDGE('',*,*,#16760,.F.);
#23655=ORIENTED_EDGE('',*,*,#16761,.F.);
#23656=ORIENTED_EDGE('',*,*,#16762,.F.);
#23657=ORIENTED_EDGE('',*,*,#16763,.T.);
#23658=ORIENTED_EDGE('',*,*,#16764,.T.);
#23659=ORIENTED_EDGE('',*,*,#16765,.T.);
#23660=ORIENTED_EDGE('',*,*,#16766,.T.);
#23661=ORIENTED_EDGE('',*,*,#16767,.F.);
#23662=ORIENTED_EDGE('',*,*,#16768,.F.);
#23663=ORIENTED_EDGE('',*,*,#16769,.T.);
#23664=ORIENTED_EDGE('',*,*,#16770,.T.);
#23665=ORIENTED_EDGE('',*,*,#16771,.F.);
#23666=ORIENTED_EDGE('',*,*,#16772,.T.);
#23667=ORIENTED_EDGE('',*,*,#16773,.T.);
#23668=ORIENTED_EDGE('',*,*,#16774,.F.);
#23669=ORIENTED_EDGE('',*,*,#16775,.F.);
#23670=ORIENTED_EDGE('',*,*,#16776,.T.);
#23671=ORIENTED_EDGE('',*,*,#16771,.T.);
#23672=ORIENTED_EDGE('',*,*,#16777,.T.);
#23673=ORIENTED_EDGE('',*,*,#16753,.F.);
#23674=ORIENTED_EDGE('',*,*,#16461,.T.);
#23675=ORIENTED_EDGE('',*,*,#16722,.T.);
#23676=ORIENTED_EDGE('',*,*,#16778,.F.);
#23677=ORIENTED_EDGE('',*,*,#16779,.F.);
#23678=ORIENTED_EDGE('',*,*,#16707,.T.);
#23679=ORIENTED_EDGE('',*,*,#16780,.T.);
#23680=ORIENTED_EDGE('',*,*,#16726,.T.);
#23681=ORIENTED_EDGE('',*,*,#16781,.T.);
#23682=ORIENTED_EDGE('',*,*,#16711,.T.);
#23683=ORIENTED_EDGE('',*,*,#16781,.F.);
#23684=ORIENTED_EDGE('',*,*,#16729,.T.);
#23685=ORIENTED_EDGE('',*,*,#16782,.T.);
#23686=ORIENTED_EDGE('',*,*,#16698,.T.);
#23687=ORIENTED_EDGE('',*,*,#16782,.F.);
#23688=ORIENTED_EDGE('',*,*,#16727,.T.);
#23689=ORIENTED_EDGE('',*,*,#16783,.T.);
#23690=ORIENTED_EDGE('',*,*,#16693,.T.);
#23691=ORIENTED_EDGE('',*,*,#16783,.F.);
#23692=ORIENTED_EDGE('',*,*,#16728,.T.);
#23693=ORIENTED_EDGE('',*,*,#16784,.T.);
#23694=ORIENTED_EDGE('',*,*,#16688,.T.);
#23695=ORIENTED_EDGE('',*,*,#16784,.F.);
#23696=ORIENTED_EDGE('',*,*,#16785,.T.);
#23697=ORIENTED_EDGE('',*,*,#16786,.T.);
#23698=ORIENTED_EDGE('',*,*,#16787,.T.);
#23699=ORIENTED_EDGE('',*,*,#16788,.T.);
#23700=ORIENTED_EDGE('',*,*,#16789,.T.);
#23701=ORIENTED_EDGE('',*,*,#16790,.T.);
#23702=ORIENTED_EDGE('',*,*,#16791,.T.);
#23703=ORIENTED_EDGE('',*,*,#16792,.T.);
#23704=ORIENTED_EDGE('',*,*,#16785,.F.);
#23705=ORIENTED_EDGE('',*,*,#16793,.T.);
#23706=ORIENTED_EDGE('',*,*,#16624,.T.);
#23707=ORIENTED_EDGE('',*,*,#16628,.F.);
#23708=ORIENTED_EDGE('',*,*,#16794,.T.);
#23709=ORIENTED_EDGE('',*,*,#16792,.F.);
#23710=ORIENTED_EDGE('',*,*,#16795,.T.);
#23711=ORIENTED_EDGE('',*,*,#16796,.F.);
#23712=ORIENTED_EDGE('',*,*,#16797,.T.);
#23713=ORIENTED_EDGE('',*,*,#16625,.F.);
#23714=ORIENTED_EDGE('',*,*,#16793,.F.);
#23715=ORIENTED_EDGE('',*,*,#16791,.F.);
#23716=ORIENTED_EDGE('',*,*,#16798,.T.);
#23717=ORIENTED_EDGE('',*,*,#16799,.T.);
#23718=ORIENTED_EDGE('',*,*,#16795,.F.);
#23719=ORIENTED_EDGE('',*,*,#16790,.F.);
#23720=ORIENTED_EDGE('',*,*,#16800,.F.);
#23721=ORIENTED_EDGE('',*,*,#16801,.F.);
#23722=ORIENTED_EDGE('',*,*,#16802,.F.);
#23723=ORIENTED_EDGE('',*,*,#16803,.T.);
#23724=ORIENTED_EDGE('',*,*,#16600,.T.);
#23725=ORIENTED_EDGE('',*,*,#16804,.T.);
#23726=ORIENTED_EDGE('',*,*,#16805,.F.);
#23727=ORIENTED_EDGE('',*,*,#16806,.F.);
#23728=ORIENTED_EDGE('',*,*,#16798,.F.);
#23729=ORIENTED_EDGE('',*,*,#16786,.F.);
#23730=ORIENTED_EDGE('',*,*,#16794,.F.);
#23731=ORIENTED_EDGE('',*,*,#16634,.T.);
#23732=ORIENTED_EDGE('',*,*,#16807,.F.);
#23733=ORIENTED_EDGE('',*,*,#16671,.T.);
#23734=ORIENTED_EDGE('',*,*,#16808,.T.);
#23735=ORIENTED_EDGE('',*,*,#16714,.F.);
#23736=ORIENTED_EDGE('',*,*,#16635,.T.);
#23737=ORIENTED_EDGE('',*,*,#16666,.F.);
#23738=ORIENTED_EDGE('',*,*,#16808,.F.);
#23739=ORIENTED_EDGE('',*,*,#16670,.F.);
#23740=ORIENTED_EDGE('',*,*,#16809,.F.);
#23741=ORIENTED_EDGE('',*,*,#16810,.F.);
#23742=ORIENTED_EDGE('',*,*,#16718,.T.);
#23743=ORIENTED_EDGE('',*,*,#16715,.F.);
#23744=ORIENTED_EDGE('',*,*,#16811,.T.);
#23745=ORIENTED_EDGE('',*,*,#16667,.T.);
#23746=ORIENTED_EDGE('',*,*,#16664,.F.);
#23747=ORIENTED_EDGE('',*,*,#16637,.F.);
#23748=ORIENTED_EDGE('',*,*,#16713,.T.);
#23749=ORIENTED_EDGE('',*,*,#16811,.F.);
#23750=ORIENTED_EDGE('',*,*,#16717,.T.);
#23751=ORIENTED_EDGE('',*,*,#16725,.F.);
#23752=ORIENTED_EDGE('',*,*,#16812,.F.);
#23753=ORIENTED_EDGE('',*,*,#16813,.F.);
#23754=ORIENTED_EDGE('',*,*,#16668,.T.);
#23755=ORIENTED_EDGE('',*,*,#16787,.F.);
#23756=ORIENTED_EDGE('',*,*,#16807,.T.);
#23757=ORIENTED_EDGE('',*,*,#16650,.T.);
#23758=ORIENTED_EDGE('',*,*,#16654,.T.);
#23759=ORIENTED_EDGE('',*,*,#16814,.T.);
#23760=ORIENTED_EDGE('',*,*,#16788,.F.);
#23761=ORIENTED_EDGE('',*,*,#16814,.F.);
#23762=ORIENTED_EDGE('',*,*,#16653,.F.);
#23763=ORIENTED_EDGE('',*,*,#16815,.T.);
#23764=ORIENTED_EDGE('',*,*,#16816,.F.);
#23765=ORIENTED_EDGE('',*,*,#16817,.F.);
#23766=ORIENTED_EDGE('',*,*,#16818,.F.);
#23767=ORIENTED_EDGE('',*,*,#16815,.F.);
#23768=ORIENTED_EDGE('',*,*,#16652,.F.);
#23769=ORIENTED_EDGE('',*,*,#16663,.T.);
#23770=ORIENTED_EDGE('',*,*,#16640,.F.);
#23771=ORIENTED_EDGE('',*,*,#16819,.F.);
#23772=ORIENTED_EDGE('',*,*,#16820,.F.);
#23773=ORIENTED_EDGE('',*,*,#16655,.F.);
#23774=ORIENTED_EDGE('',*,*,#16647,.F.);
#23775=ORIENTED_EDGE('',*,*,#16819,.T.);
#23776=ORIENTED_EDGE('',*,*,#16639,.T.);
#23777=ORIENTED_EDGE('',*,*,#16821,.F.);
#23778=ORIENTED_EDGE('',*,*,#16822,.T.);
#23779=ORIENTED_EDGE('',*,*,#16823,.T.);
#23780=ORIENTED_EDGE('',*,*,#16824,.T.);
#23781=ORIENTED_EDGE('',*,*,#16657,.T.);
#23782=ORIENTED_EDGE('',*,*,#16825,.T.);
#23783=ORIENTED_EDGE('',*,*,#16826,.F.);
#23784=ORIENTED_EDGE('',*,*,#16827,.T.);
#23785=ORIENTED_EDGE('',*,*,#16656,.T.);
#23786=ORIENTED_EDGE('',*,*,#16820,.T.);
#23787=ORIENTED_EDGE('',*,*,#16824,.F.);
#23788=ORIENTED_EDGE('',*,*,#16828,.F.);
#23789=ORIENTED_EDGE('',*,*,#16829,.F.);
#23790=ORIENTED_EDGE('',*,*,#16830,.F.);
#23791=ORIENTED_EDGE('',*,*,#16831,.F.);
#23792=ORIENTED_EDGE('',*,*,#16832,.F.);
#23793=ORIENTED_EDGE('',*,*,#16833,.F.);
#23794=ORIENTED_EDGE('',*,*,#16834,.F.);
#23795=ORIENTED_EDGE('',*,*,#16801,.T.);
#23796=ORIENTED_EDGE('',*,*,#16835,.F.);
#23797=ORIENTED_EDGE('',*,*,#16816,.T.);
#23798=ORIENTED_EDGE('',*,*,#16818,.T.);
#23799=ORIENTED_EDGE('',*,*,#16662,.T.);
#23800=ORIENTED_EDGE('',*,*,#16836,.F.);
#23801=ORIENTED_EDGE('',*,*,#16837,.F.);
#23802=ORIENTED_EDGE('',*,*,#16838,.F.);
#23803=ORIENTED_EDGE('',*,*,#16839,.F.);
#23804=ORIENTED_EDGE('',*,*,#16825,.F.);
#23805=ORIENTED_EDGE('',*,*,#16840,.T.);
#23806=ORIENTED_EDGE('',*,*,#16841,.T.);
#23807=ORIENTED_EDGE('',*,*,#16842,.T.);
#23808=ORIENTED_EDGE('',*,*,#16843,.T.);
#23809=ORIENTED_EDGE('',*,*,#16844,.T.);
#23810=ORIENTED_EDGE('',*,*,#16845,.T.);
#23811=ORIENTED_EDGE('',*,*,#16846,.T.);
#23812=ORIENTED_EDGE('',*,*,#16847,.T.);
#23813=ORIENTED_EDGE('',*,*,#16848,.T.);
#23814=ORIENTED_EDGE('',*,*,#16849,.T.);
#23815=ORIENTED_EDGE('',*,*,#16850,.T.);
#23816=ORIENTED_EDGE('',*,*,#16851,.T.);
#23817=ORIENTED_EDGE('',*,*,#16852,.T.);
#23818=ORIENTED_EDGE('',*,*,#16853,.T.);
#23819=ORIENTED_EDGE('',*,*,#16854,.F.);
#23820=ORIENTED_EDGE('',*,*,#16855,.T.);
#23821=ORIENTED_EDGE('',*,*,#16856,.T.);
#23822=ORIENTED_EDGE('',*,*,#16857,.T.);
#23823=ORIENTED_EDGE('',*,*,#16858,.T.);
#23824=ORIENTED_EDGE('',*,*,#16859,.T.);
#23825=ORIENTED_EDGE('',*,*,#16860,.T.);
#23826=ORIENTED_EDGE('',*,*,#16861,.T.);
#23827=ORIENTED_EDGE('',*,*,#16862,.T.);
#23828=ORIENTED_EDGE('',*,*,#16863,.T.);
#23829=ORIENTED_EDGE('',*,*,#16864,.T.);
#23830=ORIENTED_EDGE('',*,*,#16865,.T.);
#23831=ORIENTED_EDGE('',*,*,#16866,.T.);
#23832=ORIENTED_EDGE('',*,*,#16867,.T.);
#23833=ORIENTED_EDGE('',*,*,#16868,.T.);
#23834=ORIENTED_EDGE('',*,*,#16869,.T.);
#23835=ORIENTED_EDGE('',*,*,#16870,.T.);
#23836=ORIENTED_EDGE('',*,*,#16871,.T.);
#23837=ORIENTED_EDGE('',*,*,#16872,.T.);
#23838=ORIENTED_EDGE('',*,*,#16873,.T.);
#23839=ORIENTED_EDGE('',*,*,#16874,.T.);
#23840=ORIENTED_EDGE('',*,*,#16679,.T.);
#23841=ORIENTED_EDGE('',*,*,#16822,.F.);
#23842=ORIENTED_EDGE('',*,*,#16821,.T.);
#23843=ORIENTED_EDGE('',*,*,#16643,.T.);
#23844=ORIENTED_EDGE('',*,*,#16680,.T.);
#23845=ORIENTED_EDGE('',*,*,#16874,.F.);
#23846=ORIENTED_EDGE('',*,*,#16642,.F.);
#23847=ORIENTED_EDGE('',*,*,#16631,.T.);
#23848=ORIENTED_EDGE('',*,*,#16603,.F.);
#23849=ORIENTED_EDGE('',*,*,#16622,.F.);
#23850=ORIENTED_EDGE('',*,*,#16875,.F.);
#23851=ORIENTED_EDGE('',*,*,#16876,.F.);
#23852=ORIENTED_EDGE('',*,*,#16611,.F.);
#23853=ORIENTED_EDGE('',*,*,#16877,.F.);
#23854=ORIENTED_EDGE('',*,*,#16614,.T.);
#23855=ORIENTED_EDGE('',*,*,#16626,.F.);
#23856=ORIENTED_EDGE('',*,*,#16797,.F.);
#23857=ORIENTED_EDGE('',*,*,#16617,.T.);
#23858=ORIENTED_EDGE('',*,*,#16878,.F.);
#23859=ORIENTED_EDGE('',*,*,#16879,.T.);
#23860=ORIENTED_EDGE('',*,*,#16880,.F.);
#23861=ORIENTED_EDGE('',*,*,#16616,.T.);
#23862=ORIENTED_EDGE('',*,*,#16881,.T.);
#23863=ORIENTED_EDGE('',*,*,#16882,.F.);
#23864=ORIENTED_EDGE('',*,*,#16878,.T.);
#23865=ORIENTED_EDGE('',*,*,#16615,.T.);
#23866=ORIENTED_EDGE('',*,*,#16877,.T.);
#23867=ORIENTED_EDGE('',*,*,#16796,.T.);
#23868=ORIENTED_EDGE('',*,*,#16799,.F.);
#23869=ORIENTED_EDGE('',*,*,#16806,.T.);
#23870=ORIENTED_EDGE('',*,*,#16883,.F.);
#23871=ORIENTED_EDGE('',*,*,#16884,.F.);
#23872=ORIENTED_EDGE('',*,*,#16885,.F.);
#23873=ORIENTED_EDGE('',*,*,#16886,.F.);
#23874=ORIENTED_EDGE('',*,*,#16887,.F.);
#23875=ORIENTED_EDGE('',*,*,#16888,.F.);
#23876=ORIENTED_EDGE('',*,*,#16889,.F.);
#23877=ORIENTED_EDGE('',*,*,#16890,.F.);
#23878=ORIENTED_EDGE('',*,*,#16875,.T.);
#23879=ORIENTED_EDGE('',*,*,#16621,.T.);
#23880=ORIENTED_EDGE('',*,*,#16891,.F.);
#23881=ORIENTED_EDGE('',*,*,#16892,.F.);
#23882=ORIENTED_EDGE('',*,*,#16893,.F.);
#23883=ORIENTED_EDGE('',*,*,#16894,.F.);
#23884=ORIENTED_EDGE('',*,*,#16881,.F.);
#23885=ORIENTED_EDGE('',*,*,#16895,.F.);
#23886=ORIENTED_EDGE('',*,*,#16876,.T.);
#23887=ORIENTED_EDGE('',*,*,#16890,.T.);
#23888=ORIENTED_EDGE('',*,*,#16896,.F.);
#23889=ORIENTED_EDGE('',*,*,#16897,.T.);
#23890=ORIENTED_EDGE('',*,*,#16898,.T.);
#23891=ORIENTED_EDGE('',*,*,#16606,.F.);
#23892=ORIENTED_EDGE('',*,*,#16897,.F.);
#23893=ORIENTED_EDGE('',*,*,#16682,.T.);
#23894=ORIENTED_EDGE('',*,*,#16899,.F.);
#23895=ORIENTED_EDGE('',*,*,#16607,.F.);
#23896=ORIENTED_EDGE('',*,*,#16898,.F.);
#23897=ORIENTED_EDGE('',*,*,#16899,.T.);
#23898=ORIENTED_EDGE('',*,*,#16681,.T.);
#23899=ORIENTED_EDGE('',*,*,#16629,.T.);
#23900=ORIENTED_EDGE('',*,*,#16608,.T.);
#23901=ORIENTED_EDGE('',*,*,#16810,.T.);
#23902=ORIENTED_EDGE('',*,*,#16900,.F.);
#23903=ORIENTED_EDGE('',*,*,#16901,.F.);
#23904=ORIENTED_EDGE('',*,*,#16719,.F.);
#23905=ORIENTED_EDGE('',*,*,#16812,.T.);
#23906=ORIENTED_EDGE('',*,*,#16724,.F.);
#23907=ORIENTED_EDGE('',*,*,#16902,.F.);
#23908=ORIENTED_EDGE('',*,*,#16903,.F.);
#23909=ORIENTED_EDGE('',*,*,#16904,.F.);
#23910=ORIENTED_EDGE('',*,*,#16905,.F.);
#23911=ORIENTED_EDGE('',*,*,#16906,.F.);
#23912=ORIENTED_EDGE('',*,*,#16907,.F.);
#23913=ORIENTED_EDGE('',*,*,#16772,.F.);
#23914=ORIENTED_EDGE('',*,*,#16803,.F.);
#23915=ORIENTED_EDGE('',*,*,#16908,.F.);
#23916=ORIENTED_EDGE('',*,*,#16804,.F.);
#23917=ORIENTED_EDGE('',*,*,#16770,.F.);
#23918=ORIENTED_EDGE('',*,*,#16909,.F.);
#23919=ORIENTED_EDGE('',*,*,#16910,.F.);
#23920=ORIENTED_EDGE('',*,*,#16911,.F.);
#23921=ORIENTED_EDGE('',*,*,#16912,.F.);
#23922=ORIENTED_EDGE('',*,*,#16777,.F.);
#23923=ORIENTED_EDGE('',*,*,#16599,.F.);
#23924=ORIENTED_EDGE('',*,*,#16913,.F.);
#23925=ORIENTED_EDGE('',*,*,#16601,.F.);
#23926=ORIENTED_EDGE('',*,*,#16776,.F.);
#23927=ORIENTED_EDGE('',*,*,#16913,.T.);
#23928=ORIENTED_EDGE('',*,*,#16775,.T.);
#23929=ORIENTED_EDGE('',*,*,#16914,.F.);
#23930=ORIENTED_EDGE('',*,*,#16593,.T.);
#23931=ORIENTED_EDGE('',*,*,#16581,.F.);
#23932=ORIENTED_EDGE('',*,*,#16597,.T.);
#23933=ORIENTED_EDGE('',*,*,#16912,.T.);
#23934=ORIENTED_EDGE('',*,*,#16598,.T.);
#23935=ORIENTED_EDGE('',*,*,#16590,.F.);
#23936=ORIENTED_EDGE('',*,*,#16915,.T.);
#23937=ORIENTED_EDGE('',*,*,#16916,.F.);
#23938=ORIENTED_EDGE('',*,*,#16767,.T.);
#23939=ORIENTED_EDGE('',*,*,#16706,.T.);
#23940=ORIENTED_EDGE('',*,*,#16917,.T.);
#23941=ORIENTED_EDGE('',*,*,#16918,.T.);
#23942=ORIENTED_EDGE('',*,*,#16462,.T.);
#23943=ORIENTED_EDGE('',*,*,#16780,.F.);
#23944=ORIENTED_EDGE('',*,*,#16704,.T.);
#23945=ORIENTED_EDGE('',*,*,#16919,.T.);
#23946=ORIENTED_EDGE('',*,*,#16888,.T.);
#23947=ORIENTED_EDGE('',*,*,#16920,.F.);
#23948=ORIENTED_EDGE('',*,*,#16905,.T.);
#23949=ORIENTED_EDGE('',*,*,#16921,.F.);
#23950=ORIENTED_EDGE('',*,*,#16922,.F.);
#23951=ORIENTED_EDGE('',*,*,#16789,.F.);
#23952=ORIENTED_EDGE('',*,*,#16817,.T.);
#23953=ORIENTED_EDGE('',*,*,#16835,.T.);
#23954=ORIENTED_EDGE('',*,*,#16800,.T.);
#23955=ORIENTED_EDGE('',*,*,#16805,.T.);
#23956=ORIENTED_EDGE('',*,*,#16908,.T.);
#23957=ORIENTED_EDGE('',*,*,#16923,.T.);
#23958=ORIENTED_EDGE('',*,*,#16924,.T.);
#23959=ORIENTED_EDGE('',*,*,#16925,.T.);
#23960=ORIENTED_EDGE('',*,*,#16883,.T.);
#23961=ORIENTED_EDGE('',*,*,#16909,.T.);
#23962=ORIENTED_EDGE('',*,*,#16769,.F.);
#23963=ORIENTED_EDGE('',*,*,#16926,.F.);
#23964=ORIENTED_EDGE('',*,*,#16911,.T.);
#23965=ORIENTED_EDGE('',*,*,#16927,.F.);
#23966=ORIENTED_EDGE('',*,*,#16923,.F.);
#23967=ORIENTED_EDGE('',*,*,#16747,.F.);
#23968=ORIENTED_EDGE('',*,*,#16750,.F.);
#23969=ORIENTED_EDGE('',*,*,#16928,.F.);
#23970=ORIENTED_EDGE('',*,*,#16929,.F.);
#23971=ORIENTED_EDGE('',*,*,#16735,.F.);
#23972=ORIENTED_EDGE('',*,*,#16930,.F.);
#23973=ORIENTED_EDGE('',*,*,#16931,.F.);
#23974=ORIENTED_EDGE('',*,*,#16932,.F.);
#23975=ORIENTED_EDGE('',*,*,#16933,.F.);
#23976=ORIENTED_EDGE('',*,*,#16928,.T.);
#23977=ORIENTED_EDGE('',*,*,#16749,.F.);
#23978=ORIENTED_EDGE('',*,*,#16752,.T.);
#23979=ORIENTED_EDGE('',*,*,#16934,.F.);
#23980=ORIENTED_EDGE('',*,*,#16743,.T.);
#23981=ORIENTED_EDGE('',*,*,#16935,.F.);
#23982=ORIENTED_EDGE('',*,*,#16931,.T.);
#23983=ORIENTED_EDGE('',*,*,#16736,.F.);
#23984=ORIENTED_EDGE('',*,*,#16932,.T.);
#23985=ORIENTED_EDGE('',*,*,#16935,.T.);
#23986=ORIENTED_EDGE('',*,*,#16742,.T.);
#23987=ORIENTED_EDGE('',*,*,#16741,.T.);
#23988=ORIENTED_EDGE('',*,*,#16936,.F.);
#23989=ORIENTED_EDGE('',*,*,#16709,.T.);
#23990=ORIENTED_EDGE('',*,*,#16937,.F.);
#23991=ORIENTED_EDGE('',*,*,#16938,.F.);
#23992=ORIENTED_EDGE('',*,*,#16917,.F.);
#23993=ORIENTED_EDGE('',*,*,#16705,.T.);
#23994=ORIENTED_EDGE('',*,*,#16939,.F.);
#23995=ORIENTED_EDGE('',*,*,#16933,.T.);
#23996=ORIENTED_EDGE('',*,*,#16940,.T.);
#23997=ORIENTED_EDGE('',*,*,#16831,.T.);
#23998=ORIENTED_EDGE('',*,*,#16941,.F.);
#23999=ORIENTED_EDGE('',*,*,#16660,.T.);
#24000=ORIENTED_EDGE('',*,*,#16942,.F.);
#24001=ORIENTED_EDGE('',*,*,#16943,.T.);
#24002=ORIENTED_EDGE('',*,*,#16944,.F.);
#24003=ORIENTED_EDGE('',*,*,#16945,.F.);
#24004=ORIENTED_EDGE('',*,*,#16943,.F.);
#24005=ORIENTED_EDGE('',*,*,#16946,.F.);
#24006=ORIENTED_EDGE('',*,*,#16947,.F.);
#24007=ORIENTED_EDGE('',*,*,#16948,.F.);
#24008=ORIENTED_EDGE('',*,*,#16949,.F.);
#24009=ORIENTED_EDGE('',*,*,#16950,.F.);
#24010=ORIENTED_EDGE('',*,*,#16879,.F.);
#24011=ORIENTED_EDGE('',*,*,#16813,.T.);
#24012=ORIENTED_EDGE('',*,*,#16903,.T.);
#24013=ORIENTED_EDGE('',*,*,#16951,.F.);
#24014=ORIENTED_EDGE('',*,*,#16952,.F.);
#24015=ORIENTED_EDGE('',*,*,#16953,.F.);
#24016=ORIENTED_EDGE('',*,*,#16900,.T.);
#24017=ORIENTED_EDGE('',*,*,#16809,.T.);
#24018=ORIENTED_EDGE('',*,*,#16669,.T.);
#24019=ORIENTED_EDGE('',*,*,#16954,.F.);
#24020=ORIENTED_EDGE('',*,*,#16955,.F.);
#24021=ORIENTED_EDGE('',*,*,#16956,.F.);
#24022=ORIENTED_EDGE('',*,*,#16957,.T.);
#24023=ORIENTED_EDGE('',*,*,#16958,.F.);
#24024=ORIENTED_EDGE('',*,*,#16959,.T.);
#24025=ORIENTED_EDGE('',*,*,#16960,.F.);
#24026=ORIENTED_EDGE('',*,*,#16961,.F.);
#24027=ORIENTED_EDGE('',*,*,#16658,.T.);
#24028=ORIENTED_EDGE('',*,*,#16827,.F.);
#24029=ORIENTED_EDGE('',*,*,#16957,.F.);
#24030=ORIENTED_EDGE('',*,*,#16962,.F.);
#24031=ORIENTED_EDGE('',*,*,#16659,.T.);
#24032=ORIENTED_EDGE('',*,*,#16962,.T.);
#24033=ORIENTED_EDGE('',*,*,#16956,.T.);
#24034=ORIENTED_EDGE('',*,*,#16963,.T.);
#24035=ORIENTED_EDGE('',*,*,#16946,.T.);
#24036=ORIENTED_EDGE('',*,*,#16942,.T.);
#24037=ORIENTED_EDGE('',*,*,#16619,.T.);
#24038=ORIENTED_EDGE('',*,*,#16964,.F.);
#24039=ORIENTED_EDGE('',*,*,#16959,.F.);
#24040=ORIENTED_EDGE('',*,*,#16965,.F.);
#24041=ORIENTED_EDGE('',*,*,#16955,.T.);
#24042=ORIENTED_EDGE('',*,*,#16966,.T.);
#24043=ORIENTED_EDGE('',*,*,#16961,.T.);
#24044=ORIENTED_EDGE('',*,*,#16967,.F.);
#24045=ORIENTED_EDGE('',*,*,#16949,.T.);
#24046=ORIENTED_EDGE('',*,*,#16968,.T.);
#24047=ORIENTED_EDGE('',*,*,#16947,.T.);
#24048=ORIENTED_EDGE('',*,*,#16963,.F.);
#24049=ORIENTED_EDGE('',*,*,#16618,.T.);
#24050=ORIENTED_EDGE('',*,*,#16880,.T.);
#24051=ORIENTED_EDGE('',*,*,#16950,.T.);
#24052=ORIENTED_EDGE('',*,*,#16967,.T.);
#24053=ORIENTED_EDGE('',*,*,#16960,.T.);
#24054=ORIENTED_EDGE('',*,*,#16964,.T.);
#24055=ORIENTED_EDGE('',*,*,#16620,.T.);
#24056=ORIENTED_EDGE('',*,*,#16965,.T.);
#24057=ORIENTED_EDGE('',*,*,#16969,.T.);
#24058=ORIENTED_EDGE('',*,*,#16891,.T.);
#24059=ORIENTED_EDGE('',*,*,#16902,.T.);
#24060=ORIENTED_EDGE('',*,*,#16723,.F.);
#24061=ORIENTED_EDGE('',*,*,#16459,.T.);
#24062=ORIENTED_EDGE('',*,*,#16970,.T.);
#24063=ORIENTED_EDGE('',*,*,#16951,.T.);
#24064=ORIENTED_EDGE('',*,*,#16584,.F.);
#24065=ORIENTED_EDGE('',*,*,#16596,.F.);
#24066=ORIENTED_EDGE('',*,*,#16971,.T.);
#24067=ORIENTED_EDGE('',*,*,#16972,.F.);
#24068=ORIENTED_EDGE('',*,*,#16587,.F.);
#24069=ORIENTED_EDGE('',*,*,#16973,.F.);
#24070=ORIENTED_EDGE('',*,*,#16974,.T.);
#24071=ORIENTED_EDGE('',*,*,#16975,.F.);
#24072=ORIENTED_EDGE('',*,*,#16976,.F.);
#24073=ORIENTED_EDGE('',*,*,#16977,.F.);
#24074=ORIENTED_EDGE('',*,*,#16971,.F.);
#24075=ORIENTED_EDGE('',*,*,#16595,.F.);
#24076=ORIENTED_EDGE('',*,*,#16978,.F.);
#24077=ORIENTED_EDGE('',*,*,#16979,.F.);
#24078=ORIENTED_EDGE('',*,*,#16974,.F.);
#24079=ORIENTED_EDGE('',*,*,#16980,.F.);
#24080=ORIENTED_EDGE('',*,*,#16585,.F.);
#24081=ORIENTED_EDGE('',*,*,#16981,.F.);
#24082=ORIENTED_EDGE('',*,*,#16589,.F.);
#24083=ORIENTED_EDGE('',*,*,#16580,.F.);
#24084=ORIENTED_EDGE('',*,*,#16588,.F.);
#24085=ORIENTED_EDGE('',*,*,#16975,.T.);
#24086=ORIENTED_EDGE('',*,*,#16979,.T.);
#24087=ORIENTED_EDGE('',*,*,#16982,.F.);
#24088=ORIENTED_EDGE('',*,*,#16915,.F.);
#24089=ORIENTED_EDGE('',*,*,#16592,.F.);
#24090=ORIENTED_EDGE('',*,*,#16910,.T.);
#24091=ORIENTED_EDGE('',*,*,#16926,.T.);
#24092=ORIENTED_EDGE('',*,*,#16768,.T.);
#24093=ORIENTED_EDGE('',*,*,#16916,.T.);
#24094=ORIENTED_EDGE('',*,*,#16982,.T.);
#24095=ORIENTED_EDGE('',*,*,#16978,.T.);
#24096=ORIENTED_EDGE('',*,*,#16983,.F.);
#24097=ORIENTED_EDGE('',*,*,#16984,.T.);
#24098=ORIENTED_EDGE('',*,*,#16924,.F.);
#24099=ORIENTED_EDGE('',*,*,#16927,.T.);
#24100=ORIENTED_EDGE('',*,*,#16980,.T.);
#24101=ORIENTED_EDGE('',*,*,#16985,.T.);
#24102=ORIENTED_EDGE('',*,*,#16884,.T.);
#24103=ORIENTED_EDGE('',*,*,#16925,.F.);
#24104=ORIENTED_EDGE('',*,*,#16984,.F.);
#24105=ORIENTED_EDGE('',*,*,#16983,.T.);
#24106=ORIENTED_EDGE('',*,*,#16739,.T.);
#24107=ORIENTED_EDGE('',*,*,#16986,.F.);
#24108=ORIENTED_EDGE('',*,*,#16981,.T.);
#24109=ORIENTED_EDGE('',*,*,#16987,.F.);
#24110=ORIENTED_EDGE('',*,*,#16865,.F.);
#24111=ORIENTED_EDGE('',*,*,#16988,.T.);
#24112=ORIENTED_EDGE('',*,*,#16989,.F.);
#24113=ORIENTED_EDGE('',*,*,#16990,.F.);
#24114=ORIENTED_EDGE('',*,*,#16866,.F.);
#24115=ORIENTED_EDGE('',*,*,#16990,.T.);
#24116=ORIENTED_EDGE('',*,*,#16991,.F.);
#24117=ORIENTED_EDGE('',*,*,#16992,.F.);
#24118=ORIENTED_EDGE('',*,*,#16867,.F.);
#24119=ORIENTED_EDGE('',*,*,#16992,.T.);
#24120=ORIENTED_EDGE('',*,*,#16993,.F.);
#24121=ORIENTED_EDGE('',*,*,#16994,.F.);
#24122=ORIENTED_EDGE('',*,*,#16868,.F.);
#24123=ORIENTED_EDGE('',*,*,#16994,.T.);
#24124=ORIENTED_EDGE('',*,*,#16995,.F.);
#24125=ORIENTED_EDGE('',*,*,#16996,.F.);
#24126=ORIENTED_EDGE('',*,*,#16869,.F.);
#24127=ORIENTED_EDGE('',*,*,#16996,.T.);
#24128=ORIENTED_EDGE('',*,*,#16997,.F.);
#24129=ORIENTED_EDGE('',*,*,#16998,.F.);
#24130=ORIENTED_EDGE('',*,*,#16870,.F.);
#24131=ORIENTED_EDGE('',*,*,#16998,.T.);
#24132=ORIENTED_EDGE('',*,*,#16999,.F.);
#24133=ORIENTED_EDGE('',*,*,#17000,.F.);
#24134=ORIENTED_EDGE('',*,*,#16871,.F.);
#24135=ORIENTED_EDGE('',*,*,#17000,.T.);
#24136=ORIENTED_EDGE('',*,*,#17001,.F.);
#24137=ORIENTED_EDGE('',*,*,#17002,.F.);
#24138=ORIENTED_EDGE('',*,*,#16872,.F.);
#24139=ORIENTED_EDGE('',*,*,#17002,.T.);
#24140=ORIENTED_EDGE('',*,*,#17003,.F.);
#24141=ORIENTED_EDGE('',*,*,#17004,.F.);
#24142=ORIENTED_EDGE('',*,*,#16873,.F.);
#24143=ORIENTED_EDGE('',*,*,#17004,.T.);
#24144=ORIENTED_EDGE('',*,*,#17005,.F.);
#24145=ORIENTED_EDGE('',*,*,#16988,.F.);
#24146=ORIENTED_EDGE('',*,*,#17005,.T.);
#24147=ORIENTED_EDGE('',*,*,#17003,.T.);
#24148=ORIENTED_EDGE('',*,*,#17001,.T.);
#24149=ORIENTED_EDGE('',*,*,#16999,.T.);
#24150=ORIENTED_EDGE('',*,*,#16997,.T.);
#24151=ORIENTED_EDGE('',*,*,#16995,.T.);
#24152=ORIENTED_EDGE('',*,*,#16993,.T.);
#24153=ORIENTED_EDGE('',*,*,#16991,.T.);
#24154=ORIENTED_EDGE('',*,*,#16989,.T.);
#24155=ORIENTED_EDGE('',*,*,#16855,.F.);
#24156=ORIENTED_EDGE('',*,*,#17006,.T.);
#24157=ORIENTED_EDGE('',*,*,#17007,.F.);
#24158=ORIENTED_EDGE('',*,*,#17008,.F.);
#24159=ORIENTED_EDGE('',*,*,#16856,.F.);
#24160=ORIENTED_EDGE('',*,*,#17008,.T.);
#24161=ORIENTED_EDGE('',*,*,#17009,.F.);
#24162=ORIENTED_EDGE('',*,*,#17010,.F.);
#24163=ORIENTED_EDGE('',*,*,#16857,.F.);
#24164=ORIENTED_EDGE('',*,*,#17010,.T.);
#24165=ORIENTED_EDGE('',*,*,#17011,.F.);
#24166=ORIENTED_EDGE('',*,*,#17012,.F.);
#24167=ORIENTED_EDGE('',*,*,#16858,.F.);
#24168=ORIENTED_EDGE('',*,*,#17012,.T.);
#24169=ORIENTED_EDGE('',*,*,#17013,.F.);
#24170=ORIENTED_EDGE('',*,*,#17014,.F.);
#24171=ORIENTED_EDGE('',*,*,#16859,.F.);
#24172=ORIENTED_EDGE('',*,*,#17014,.T.);
#24173=ORIENTED_EDGE('',*,*,#17015,.F.);
#24174=ORIENTED_EDGE('',*,*,#17016,.F.);
#24175=ORIENTED_EDGE('',*,*,#16860,.F.);
#24176=ORIENTED_EDGE('',*,*,#17016,.T.);
#24177=ORIENTED_EDGE('',*,*,#17017,.F.);
#24178=ORIENTED_EDGE('',*,*,#17018,.F.);
#24179=ORIENTED_EDGE('',*,*,#16861,.F.);
#24180=ORIENTED_EDGE('',*,*,#17018,.T.);
#24181=ORIENTED_EDGE('',*,*,#17019,.F.);
#24182=ORIENTED_EDGE('',*,*,#17020,.F.);
#24183=ORIENTED_EDGE('',*,*,#16862,.F.);
#24184=ORIENTED_EDGE('',*,*,#17020,.T.);
#24185=ORIENTED_EDGE('',*,*,#17021,.F.);
#24186=ORIENTED_EDGE('',*,*,#17022,.F.);
#24187=ORIENTED_EDGE('',*,*,#16863,.F.);
#24188=ORIENTED_EDGE('',*,*,#17022,.T.);
#24189=ORIENTED_EDGE('',*,*,#17023,.F.);
#24190=ORIENTED_EDGE('',*,*,#17024,.F.);
#24191=ORIENTED_EDGE('',*,*,#16864,.F.);
#24192=ORIENTED_EDGE('',*,*,#17024,.T.);
#24193=ORIENTED_EDGE('',*,*,#17025,.F.);
#24194=ORIENTED_EDGE('',*,*,#17006,.F.);
#24195=ORIENTED_EDGE('',*,*,#17025,.T.);
#24196=ORIENTED_EDGE('',*,*,#17023,.T.);
#24197=ORIENTED_EDGE('',*,*,#17021,.T.);
#24198=ORIENTED_EDGE('',*,*,#17019,.T.);
#24199=ORIENTED_EDGE('',*,*,#17017,.T.);
#24200=ORIENTED_EDGE('',*,*,#17015,.T.);
#24201=ORIENTED_EDGE('',*,*,#17013,.T.);
#24202=ORIENTED_EDGE('',*,*,#17011,.T.);
#24203=ORIENTED_EDGE('',*,*,#17009,.T.);
#24204=ORIENTED_EDGE('',*,*,#17007,.T.);
#24205=ORIENTED_EDGE('',*,*,#17026,.F.);
#24206=ORIENTED_EDGE('',*,*,#17027,.T.);
#24207=ORIENTED_EDGE('',*,*,#17028,.F.);
#24208=ORIENTED_EDGE('',*,*,#17029,.F.);
#24209=ORIENTED_EDGE('',*,*,#17030,.F.);
#24210=ORIENTED_EDGE('',*,*,#17029,.T.);
#24211=ORIENTED_EDGE('',*,*,#17031,.F.);
#24212=ORIENTED_EDGE('',*,*,#17032,.F.);
#24213=ORIENTED_EDGE('',*,*,#17033,.F.);
#24214=ORIENTED_EDGE('',*,*,#17032,.T.);
#24215=ORIENTED_EDGE('',*,*,#17034,.F.);
#24216=ORIENTED_EDGE('',*,*,#17035,.F.);
#24217=ORIENTED_EDGE('',*,*,#17036,.F.);
#24218=ORIENTED_EDGE('',*,*,#17035,.T.);
#24219=ORIENTED_EDGE('',*,*,#17037,.F.);
#24220=ORIENTED_EDGE('',*,*,#17038,.F.);
#24221=ORIENTED_EDGE('',*,*,#17039,.F.);
#24222=ORIENTED_EDGE('',*,*,#17038,.T.);
#24223=ORIENTED_EDGE('',*,*,#17040,.F.);
#24224=ORIENTED_EDGE('',*,*,#17041,.F.);
#24225=ORIENTED_EDGE('',*,*,#17042,.F.);
#24226=ORIENTED_EDGE('',*,*,#17041,.T.);
#24227=ORIENTED_EDGE('',*,*,#17043,.F.);
#24228=ORIENTED_EDGE('',*,*,#17044,.F.);
#24229=ORIENTED_EDGE('',*,*,#17045,.F.);
#24230=ORIENTED_EDGE('',*,*,#17044,.T.);
#24231=ORIENTED_EDGE('',*,*,#17046,.F.);
#24232=ORIENTED_EDGE('',*,*,#17047,.F.);
#24233=ORIENTED_EDGE('',*,*,#17048,.F.);
#24234=ORIENTED_EDGE('',*,*,#17047,.T.);
#24235=ORIENTED_EDGE('',*,*,#17049,.F.);
#24236=ORIENTED_EDGE('',*,*,#17027,.F.);
#24237=ORIENTED_EDGE('',*,*,#16840,.F.);
#24238=ORIENTED_EDGE('',*,*,#17050,.T.);
#24239=ORIENTED_EDGE('',*,*,#17051,.F.);
#24240=ORIENTED_EDGE('',*,*,#17052,.F.);
#24241=ORIENTED_EDGE('',*,*,#16841,.F.);
#24242=ORIENTED_EDGE('',*,*,#17052,.T.);
#24243=ORIENTED_EDGE('',*,*,#17053,.F.);
#24244=ORIENTED_EDGE('',*,*,#17054,.F.);
#24245=ORIENTED_EDGE('',*,*,#16842,.F.);
#24246=ORIENTED_EDGE('',*,*,#17054,.T.);
#24247=ORIENTED_EDGE('',*,*,#17055,.F.);
#24248=ORIENTED_EDGE('',*,*,#17056,.F.);
#24249=ORIENTED_EDGE('',*,*,#16843,.F.);
#24250=ORIENTED_EDGE('',*,*,#17056,.T.);
#24251=ORIENTED_EDGE('',*,*,#17057,.F.);
#24252=ORIENTED_EDGE('',*,*,#17058,.F.);
#24253=ORIENTED_EDGE('',*,*,#16844,.F.);
#24254=ORIENTED_EDGE('',*,*,#17058,.T.);
#24255=ORIENTED_EDGE('',*,*,#17059,.F.);
#24256=ORIENTED_EDGE('',*,*,#17060,.F.);
#24257=ORIENTED_EDGE('',*,*,#16845,.F.);
#24258=ORIENTED_EDGE('',*,*,#17060,.T.);
#24259=ORIENTED_EDGE('',*,*,#17061,.F.);
#24260=ORIENTED_EDGE('',*,*,#17062,.F.);
#24261=ORIENTED_EDGE('',*,*,#16846,.F.);
#24262=ORIENTED_EDGE('',*,*,#17062,.T.);
#24263=ORIENTED_EDGE('',*,*,#17063,.F.);
#24264=ORIENTED_EDGE('',*,*,#17064,.F.);
#24265=ORIENTED_EDGE('',*,*,#16847,.F.);
#24266=ORIENTED_EDGE('',*,*,#17064,.T.);
#24267=ORIENTED_EDGE('',*,*,#17065,.F.);
#24268=ORIENTED_EDGE('',*,*,#17066,.F.);
#24269=ORIENTED_EDGE('',*,*,#16848,.F.);
#24270=ORIENTED_EDGE('',*,*,#17066,.T.);
#24271=ORIENTED_EDGE('',*,*,#17067,.F.);
#24272=ORIENTED_EDGE('',*,*,#17068,.F.);
#24273=ORIENTED_EDGE('',*,*,#16849,.F.);
#24274=ORIENTED_EDGE('',*,*,#17068,.T.);
#24275=ORIENTED_EDGE('',*,*,#17069,.F.);
#24276=ORIENTED_EDGE('',*,*,#17050,.F.);
#24277=ORIENTED_EDGE('',*,*,#17069,.T.);
#24278=ORIENTED_EDGE('',*,*,#17067,.T.);
#24279=ORIENTED_EDGE('',*,*,#17065,.T.);
#24280=ORIENTED_EDGE('',*,*,#17063,.T.);
#24281=ORIENTED_EDGE('',*,*,#17061,.T.);
#24282=ORIENTED_EDGE('',*,*,#17059,.T.);
#24283=ORIENTED_EDGE('',*,*,#17057,.T.);
#24284=ORIENTED_EDGE('',*,*,#17055,.T.);
#24285=ORIENTED_EDGE('',*,*,#17053,.T.);
#24286=ORIENTED_EDGE('',*,*,#17051,.T.);
#24287=ORIENTED_EDGE('',*,*,#17049,.T.);
#24288=ORIENTED_EDGE('',*,*,#17046,.T.);
#24289=ORIENTED_EDGE('',*,*,#17043,.T.);
#24290=ORIENTED_EDGE('',*,*,#17040,.T.);
#24291=ORIENTED_EDGE('',*,*,#17037,.T.);
#24292=ORIENTED_EDGE('',*,*,#17034,.T.);
#24293=ORIENTED_EDGE('',*,*,#17031,.T.);
#24294=ORIENTED_EDGE('',*,*,#17028,.T.);
#24295=ORIENTED_EDGE('',*,*,#16850,.F.);
#24296=ORIENTED_EDGE('',*,*,#17070,.T.);
#24297=ORIENTED_EDGE('',*,*,#17071,.F.);
#24298=ORIENTED_EDGE('',*,*,#17072,.F.);
#24299=ORIENTED_EDGE('',*,*,#16851,.F.);
#24300=ORIENTED_EDGE('',*,*,#17072,.T.);
#24301=ORIENTED_EDGE('',*,*,#17073,.F.);
#24302=ORIENTED_EDGE('',*,*,#17074,.F.);
#24303=ORIENTED_EDGE('',*,*,#16852,.F.);
#24304=ORIENTED_EDGE('',*,*,#17074,.T.);
#24305=ORIENTED_EDGE('',*,*,#17075,.F.);
#24306=ORIENTED_EDGE('',*,*,#17076,.F.);
#24307=ORIENTED_EDGE('',*,*,#16853,.F.);
#24308=ORIENTED_EDGE('',*,*,#17076,.T.);
#24309=ORIENTED_EDGE('',*,*,#17077,.F.);
#24310=ORIENTED_EDGE('',*,*,#17070,.F.);
#24311=ORIENTED_EDGE('',*,*,#17077,.T.);
#24312=ORIENTED_EDGE('',*,*,#17075,.T.);
#24313=ORIENTED_EDGE('',*,*,#17073,.T.);
#24314=ORIENTED_EDGE('',*,*,#17071,.T.);
#24315=ORIENTED_EDGE('',*,*,#17078,.T.);
#24316=ORIENTED_EDGE('',*,*,#16572,.F.);
#24317=ORIENTED_EDGE('',*,*,#17078,.F.);
#24318=ORIENTED_EDGE('',*,*,#17079,.T.);
#24319=ORIENTED_EDGE('',*,*,#16766,.F.);
#24320=ORIENTED_EDGE('',*,*,#17079,.F.);
#24321=ORIENTED_EDGE('',*,*,#17080,.T.);
#24322=ORIENTED_EDGE('',*,*,#16568,.F.);
#24323=ORIENTED_EDGE('',*,*,#17080,.F.);
#24324=ORIENTED_EDGE('',*,*,#17081,.T.);
#24325=ORIENTED_EDGE('',*,*,#16764,.F.);
#24326=ORIENTED_EDGE('',*,*,#17081,.F.);
#24327=ORIENTED_EDGE('',*,*,#16563,.F.);
#24328=ORIENTED_EDGE('',*,*,#17082,.T.);
#24329=ORIENTED_EDGE('',*,*,#16765,.F.);
#24330=ORIENTED_EDGE('',*,*,#17082,.F.);
#24331=ORIENTED_EDGE('',*,*,#16556,.F.);
#24332=ORIENTED_EDGE('',*,*,#17083,.T.);
#24333=ORIENTED_EDGE('',*,*,#16763,.F.);
#24334=ORIENTED_EDGE('',*,*,#17083,.F.);
#24335=ORIENTED_EDGE('',*,*,#16501,.F.);
#24336=ORIENTED_EDGE('',*,*,#16547,.T.);
#24337=ORIENTED_EDGE('',*,*,#17084,.F.);
#24338=ORIENTED_EDGE('',*,*,#16526,.F.);
#24339=ORIENTED_EDGE('',*,*,#16513,.F.);
#24340=ORIENTED_EDGE('',*,*,#17085,.T.);
#24341=ORIENTED_EDGE('',*,*,#16545,.T.);
#24342=ORIENTED_EDGE('',*,*,#16550,.F.);
#24343=ORIENTED_EDGE('',*,*,#16522,.F.);
#24344=ORIENTED_EDGE('',*,*,#17084,.T.);
#24345=ORIENTED_EDGE('',*,*,#16546,.T.);
#24346=ORIENTED_EDGE('',*,*,#17085,.F.);
#24347=ORIENTED_EDGE('',*,*,#16519,.F.);
#24348=ORIENTED_EDGE('',*,*,#16473,.F.);
#24349=ORIENTED_EDGE('',*,*,#16755,.F.);
#24350=ORIENTED_EDGE('',*,*,#16493,.T.);
#24351=ORIENTED_EDGE('',*,*,#16484,.F.);
#24352=ORIENTED_EDGE('',*,*,#17086,.T.);
#24353=ORIENTED_EDGE('',*,*,#17087,.F.);
#24354=ORIENTED_EDGE('',*,*,#16531,.T.);
#24355=ORIENTED_EDGE('',*,*,#16495,.F.);
#24356=ORIENTED_EDGE('',*,*,#16483,.F.);
#24357=ORIENTED_EDGE('',*,*,#16489,.F.);
#24358=ORIENTED_EDGE('',*,*,#17088,.F.);
#24359=ORIENTED_EDGE('',*,*,#17086,.F.);
#24360=ORIENTED_EDGE('',*,*,#16938,.T.);
#24361=ORIENTED_EDGE('',*,*,#17089,.T.);
#24362=ORIENTED_EDGE('',*,*,#16456,.T.);
#24363=ORIENTED_EDGE('',*,*,#16918,.F.);
#24364=ORIENTED_EDGE('',*,*,#16708,.T.);
#24365=ORIENTED_EDGE('',*,*,#16779,.T.);
#24366=ORIENTED_EDGE('',*,*,#17090,.T.);
#24367=ORIENTED_EDGE('',*,*,#17089,.F.);
#24368=ORIENTED_EDGE('',*,*,#16937,.T.);
#24369=ORIENTED_EDGE('',*,*,#16454,.F.);
#24370=ORIENTED_EDGE('',*,*,#16450,.F.);
#24371=ORIENTED_EDGE('',*,*,#16457,.F.);
#24372=ORIENTED_EDGE('',*,*,#17090,.F.);
#24373=ORIENTED_EDGE('',*,*,#16778,.T.);
#24374=ORIENTED_EDGE('',*,*,#16721,.T.);
#24375=ORIENTED_EDGE('',*,*,#17091,.F.);
#24376=ORIENTED_EDGE('',*,*,#17092,.F.);
#24377=ORIENTED_EDGE('',*,*,#16446,.F.);
#24378=ORIENTED_EDGE('',*,*,#16952,.T.);
#24379=ORIENTED_EDGE('',*,*,#16970,.F.);
#24380=ORIENTED_EDGE('',*,*,#17093,.T.);
#24381=ORIENTED_EDGE('',*,*,#17094,.T.);
#24382=ORIENTED_EDGE('',*,*,#16901,.T.);
#24383=ORIENTED_EDGE('',*,*,#16953,.T.);
#24384=ORIENTED_EDGE('',*,*,#17094,.F.);
#24385=ORIENTED_EDGE('',*,*,#17091,.T.);
#24386=ORIENTED_EDGE('',*,*,#16720,.T.);
#24387=ORIENTED_EDGE('',*,*,#16442,.F.);
#24388=ORIENTED_EDGE('',*,*,#17092,.T.);
#24389=ORIENTED_EDGE('',*,*,#17093,.F.);
#24390=ORIENTED_EDGE('',*,*,#16458,.F.);
#24391=ORIENTED_EDGE('',*,*,#17095,.T.);
#24392=ORIENTED_EDGE('',*,*,#17096,.T.);
#24393=ORIENTED_EDGE('',*,*,#16466,.T.);
#24394=ORIENTED_EDGE('',*,*,#17096,.F.);
#24395=ORIENTED_EDGE('',*,*,#17097,.F.);
#24396=ORIENTED_EDGE('',*,*,#17095,.F.);
#24397=ORIENTED_EDGE('',*,*,#17098,.T.);
#24398=ORIENTED_EDGE('',*,*,#17099,.T.);
#24399=ORIENTED_EDGE('',*,*,#16463,.T.);
#24400=ORIENTED_EDGE('',*,*,#17099,.F.);
#24401=ORIENTED_EDGE('',*,*,#17100,.F.);
#24402=ORIENTED_EDGE('',*,*,#17098,.F.);
#24403=ORIENTED_EDGE('',*,*,#16854,.T.);
#24404=ORIENTED_EDGE('',*,*,#17101,.T.);
#24405=ORIENTED_EDGE('',*,*,#17102,.T.);
#24406=ORIENTED_EDGE('',*,*,#17101,.F.);
#24407=ORIENTED_EDGE('',*,*,#17102,.F.);
#24408=ORIENTED_EDGE('',*,*,#17103,.T.);
#24409=ORIENTED_EDGE('',*,*,#17104,.F.);
#24410=ORIENTED_EDGE('',*,*,#17103,.F.);
#24411=ORIENTED_EDGE('',*,*,#17026,.T.);
#24412=ORIENTED_EDGE('',*,*,#17030,.T.);
#24413=ORIENTED_EDGE('',*,*,#17033,.T.);
#24414=ORIENTED_EDGE('',*,*,#17036,.T.);
#24415=ORIENTED_EDGE('',*,*,#17039,.T.);
#24416=ORIENTED_EDGE('',*,*,#17042,.T.);
#24417=ORIENTED_EDGE('',*,*,#17045,.T.);
#24418=ORIENTED_EDGE('',*,*,#17048,.T.);
#24419=ORIENTED_EDGE('',*,*,#17100,.T.);
#24420=ORIENTED_EDGE('',*,*,#17105,.T.);
#24421=ORIENTED_EDGE('',*,*,#17104,.T.);
#24422=ORIENTED_EDGE('',*,*,#17105,.F.);
#24423=ORIENTED_EDGE('',*,*,#16895,.T.);
#24424=ORIENTED_EDGE('',*,*,#17106,.T.);
#24425=ORIENTED_EDGE('',*,*,#17107,.T.);
#24426=ORIENTED_EDGE('',*,*,#17106,.F.);
#24427=ORIENTED_EDGE('',*,*,#17108,.F.);
#24428=ORIENTED_EDGE('',*,*,#17109,.T.);
#24429=ORIENTED_EDGE('',*,*,#17107,.F.);
#24430=ORIENTED_EDGE('',*,*,#17109,.F.);
#24431=ORIENTED_EDGE('',*,*,#17097,.T.);
#24432=ORIENTED_EDGE('',*,*,#17110,.T.);
#24433=ORIENTED_EDGE('',*,*,#17108,.T.);
#24434=ORIENTED_EDGE('',*,*,#17110,.F.);
#24435=ORIENTED_EDGE('',*,*,#16802,.T.);
#24436=ORIENTED_EDGE('',*,*,#16834,.T.);
#24437=ORIENTED_EDGE('',*,*,#17111,.T.);
#24438=ORIENTED_EDGE('',*,*,#17112,.T.);
#24439=ORIENTED_EDGE('',*,*,#16921,.T.);
#24440=ORIENTED_EDGE('',*,*,#16904,.T.);
#24441=ORIENTED_EDGE('',*,*,#16661,.T.);
#24442=ORIENTED_EDGE('',*,*,#16944,.T.);
#24443=ORIENTED_EDGE('',*,*,#17113,.T.);
#24444=ORIENTED_EDGE('',*,*,#16836,.T.);
#24445=ORIENTED_EDGE('',*,*,#17114,.T.);
#24446=ORIENTED_EDGE('',*,*,#16837,.T.);
#24447=ORIENTED_EDGE('',*,*,#17113,.F.);
#24448=ORIENTED_EDGE('',*,*,#16945,.T.);
#24449=ORIENTED_EDGE('',*,*,#17115,.T.);
#24450=ORIENTED_EDGE('',*,*,#16838,.T.);
#24451=ORIENTED_EDGE('',*,*,#17114,.F.);
#24452=ORIENTED_EDGE('',*,*,#17116,.T.);
#24453=ORIENTED_EDGE('',*,*,#16826,.T.);
#24454=ORIENTED_EDGE('',*,*,#16839,.T.);
#24455=ORIENTED_EDGE('',*,*,#17115,.F.);
#24456=ORIENTED_EDGE('',*,*,#16954,.T.);
#24457=ORIENTED_EDGE('',*,*,#17117,.T.);
#24458=ORIENTED_EDGE('',*,*,#16828,.T.);
#24459=ORIENTED_EDGE('',*,*,#16823,.F.);
#24460=ORIENTED_EDGE('',*,*,#16678,.T.);
#24461=ORIENTED_EDGE('',*,*,#16710,.T.);
#24462=ORIENTED_EDGE('',*,*,#17118,.T.);
#24463=ORIENTED_EDGE('',*,*,#16829,.T.);
#24464=ORIENTED_EDGE('',*,*,#17117,.F.);
#24465=ORIENTED_EDGE('',*,*,#16941,.T.);
#24466=ORIENTED_EDGE('',*,*,#16830,.T.);
#24467=ORIENTED_EDGE('',*,*,#17118,.F.);
#24468=ORIENTED_EDGE('',*,*,#16936,.T.);
#24469=ORIENTED_EDGE('',*,*,#16929,.T.);
#24470=ORIENTED_EDGE('',*,*,#17119,.T.);
#24471=ORIENTED_EDGE('',*,*,#16832,.T.);
#24472=ORIENTED_EDGE('',*,*,#16940,.F.);
#24473=ORIENTED_EDGE('',*,*,#16751,.T.);
#24474=ORIENTED_EDGE('',*,*,#16987,.T.);
#24475=ORIENTED_EDGE('',*,*,#16972,.T.);
#24476=ORIENTED_EDGE('',*,*,#16977,.T.);
#24477=ORIENTED_EDGE('',*,*,#17120,.T.);
#24478=ORIENTED_EDGE('',*,*,#17121,.F.);
#24479=ORIENTED_EDGE('',*,*,#17111,.F.);
#24480=ORIENTED_EDGE('',*,*,#16833,.T.);
#24481=ORIENTED_EDGE('',*,*,#17119,.F.);
#24482=ORIENTED_EDGE('',*,*,#17116,.F.);
#24483=ORIENTED_EDGE('',*,*,#16968,.F.);
#24484=ORIENTED_EDGE('',*,*,#17122,.F.);
#24485=ORIENTED_EDGE('',*,*,#16966,.F.);
#24486=ORIENTED_EDGE('',*,*,#16907,.T.);
#24487=ORIENTED_EDGE('',*,*,#17123,.F.);
#24488=ORIENTED_EDGE('',*,*,#16773,.F.);
#24489=ORIENTED_EDGE('',*,*,#17124,.T.);
#24490=ORIENTED_EDGE('',*,*,#16885,.T.);
#24491=ORIENTED_EDGE('',*,*,#16985,.F.);
#24492=ORIENTED_EDGE('',*,*,#16973,.T.);
#24493=ORIENTED_EDGE('',*,*,#16986,.T.);
#24494=ORIENTED_EDGE('',*,*,#16744,.T.);
#24495=ORIENTED_EDGE('',*,*,#16934,.T.);
#24496=ORIENTED_EDGE('',*,*,#17125,.T.);
#24497=ORIENTED_EDGE('',*,*,#16886,.T.);
#24498=ORIENTED_EDGE('',*,*,#17124,.F.);
#24499=ORIENTED_EDGE('',*,*,#16920,.T.);
#24500=ORIENTED_EDGE('',*,*,#16887,.T.);
#24501=ORIENTED_EDGE('',*,*,#17125,.F.);
#24502=ORIENTED_EDGE('',*,*,#16930,.T.);
#24503=ORIENTED_EDGE('',*,*,#16939,.T.);
#24504=ORIENTED_EDGE('',*,*,#16896,.T.);
#24505=ORIENTED_EDGE('',*,*,#16889,.T.);
#24506=ORIENTED_EDGE('',*,*,#16919,.F.);
#24507=ORIENTED_EDGE('',*,*,#16683,.T.);
#24508=ORIENTED_EDGE('',*,*,#17126,.T.);
#24509=ORIENTED_EDGE('',*,*,#16892,.T.);
#24510=ORIENTED_EDGE('',*,*,#16969,.F.);
#24511=ORIENTED_EDGE('',*,*,#16958,.T.);
#24512=ORIENTED_EDGE('',*,*,#17127,.T.);
#24513=ORIENTED_EDGE('',*,*,#16893,.T.);
#24514=ORIENTED_EDGE('',*,*,#17126,.F.);
#24515=ORIENTED_EDGE('',*,*,#17122,.T.);
#24516=ORIENTED_EDGE('',*,*,#16882,.T.);
#24517=ORIENTED_EDGE('',*,*,#16894,.T.);
#24518=ORIENTED_EDGE('',*,*,#17127,.F.);
#24519=ORIENTED_EDGE('',*,*,#16948,.T.);
#24520=ORIENTED_EDGE('',*,*,#17128,.T.);
#24521=ORIENTED_EDGE('',*,*,#17129,.T.);
#24522=ORIENTED_EDGE('',*,*,#17130,.T.);
#24523=ORIENTED_EDGE('',*,*,#16535,.T.);
#24524=ORIENTED_EDGE('',*,*,#17131,.T.);
#24525=ORIENTED_EDGE('',*,*,#17132,.T.);
#24526=ORIENTED_EDGE('',*,*,#17128,.F.);
#24527=ORIENTED_EDGE('',*,*,#16534,.T.);
#24528=ORIENTED_EDGE('',*,*,#17133,.T.);
#24529=ORIENTED_EDGE('',*,*,#17134,.T.);
#24530=ORIENTED_EDGE('',*,*,#17131,.F.);
#24531=ORIENTED_EDGE('',*,*,#16533,.T.);
#24532=ORIENTED_EDGE('',*,*,#17087,.T.);
#24533=ORIENTED_EDGE('',*,*,#17135,.T.);
#24534=ORIENTED_EDGE('',*,*,#17133,.F.);
#24535=ORIENTED_EDGE('',*,*,#16532,.T.);
#24536=ORIENTED_EDGE('',*,*,#17136,.T.);
#24537=ORIENTED_EDGE('',*,*,#17137,.T.);
#24538=ORIENTED_EDGE('',*,*,#16530,.F.);
#24539=ORIENTED_EDGE('',*,*,#16538,.T.);
#24540=ORIENTED_EDGE('',*,*,#17138,.T.);
#24541=ORIENTED_EDGE('',*,*,#17139,.T.);
#24542=ORIENTED_EDGE('',*,*,#17136,.F.);
#24543=ORIENTED_EDGE('',*,*,#16537,.T.);
#24544=ORIENTED_EDGE('',*,*,#17130,.F.);
#24545=ORIENTED_EDGE('',*,*,#17140,.T.);
#24546=ORIENTED_EDGE('',*,*,#17138,.F.);
#24547=ORIENTED_EDGE('',*,*,#16536,.T.);
#24548=ORIENTED_EDGE('',*,*,#17137,.F.);
#24549=ORIENTED_EDGE('',*,*,#17141,.T.);
#24550=ORIENTED_EDGE('',*,*,#17142,.F.);
#24551=ORIENTED_EDGE('',*,*,#16481,.T.);
#24552=ORIENTED_EDGE('',*,*,#17139,.F.);
#24553=ORIENTED_EDGE('',*,*,#17143,.F.);
#24554=ORIENTED_EDGE('',*,*,#17144,.F.);
#24555=ORIENTED_EDGE('',*,*,#17141,.F.);
#24556=ORIENTED_EDGE('',*,*,#17140,.F.);
#24557=ORIENTED_EDGE('',*,*,#17145,.T.);
#24558=ORIENTED_EDGE('',*,*,#17146,.F.);
#24559=ORIENTED_EDGE('',*,*,#17143,.T.);
#24560=ORIENTED_EDGE('',*,*,#17129,.F.);
#24561=ORIENTED_EDGE('',*,*,#17147,.F.);
#24562=ORIENTED_EDGE('',*,*,#17148,.F.);
#24563=ORIENTED_EDGE('',*,*,#17145,.F.);
#24564=ORIENTED_EDGE('',*,*,#16906,.T.);
#24565=ORIENTED_EDGE('',*,*,#16922,.T.);
#24566=ORIENTED_EDGE('',*,*,#17112,.F.);
#24567=ORIENTED_EDGE('',*,*,#17121,.T.);
#24568=ORIENTED_EDGE('',*,*,#17120,.F.);
#24569=ORIENTED_EDGE('',*,*,#16976,.T.);
#24570=ORIENTED_EDGE('',*,*,#16594,.T.);
#24571=ORIENTED_EDGE('',*,*,#16914,.T.);
#24572=ORIENTED_EDGE('',*,*,#16774,.T.);
#24573=ORIENTED_EDGE('',*,*,#17123,.T.);
#24574=ORIENTED_EDGE('',*,*,#16478,.T.);
#24575=ORIENTED_EDGE('',*,*,#17142,.T.);
#24576=ORIENTED_EDGE('',*,*,#17149,.T.);
#24577=ORIENTED_EDGE('',*,*,#16756,.T.);
#24578=ORIENTED_EDGE('',*,*,#17150,.T.);
#24579=ORIENTED_EDGE('',*,*,#17151,.T.);
#24580=ORIENTED_EDGE('',*,*,#16488,.F.);
#24581=ORIENTED_EDGE('',*,*,#16762,.T.);
#24582=ORIENTED_EDGE('',*,*,#17150,.F.);
#24583=ORIENTED_EDGE('',*,*,#16761,.T.);
#24584=ORIENTED_EDGE('',*,*,#17152,.T.);
#24585=ORIENTED_EDGE('',*,*,#17153,.T.);
#24586=ORIENTED_EDGE('',*,*,#17154,.T.);
#24587=ORIENTED_EDGE('',*,*,#17155,.T.);
#24588=ORIENTED_EDGE('',*,*,#17152,.F.);
#24589=ORIENTED_EDGE('',*,*,#16760,.T.);
#24590=ORIENTED_EDGE('',*,*,#17154,.F.);
#24591=ORIENTED_EDGE('',*,*,#16759,.T.);
#24592=ORIENTED_EDGE('',*,*,#17156,.T.);
#24593=ORIENTED_EDGE('',*,*,#17148,.T.);
#24594=ORIENTED_EDGE('',*,*,#17157,.T.);
#24595=ORIENTED_EDGE('',*,*,#17146,.T.);
#24596=ORIENTED_EDGE('',*,*,#17156,.F.);
#24597=ORIENTED_EDGE('',*,*,#16758,.T.);
#24598=ORIENTED_EDGE('',*,*,#17157,.F.);
#24599=ORIENTED_EDGE('',*,*,#16757,.T.);
#24600=ORIENTED_EDGE('',*,*,#17149,.F.);
#24601=ORIENTED_EDGE('',*,*,#17144,.T.);
#24602=ORIENTED_EDGE('',*,*,#17132,.F.);
#24603=ORIENTED_EDGE('',*,*,#17158,.T.);
#24604=ORIENTED_EDGE('',*,*,#17155,.F.);
#24605=ORIENTED_EDGE('',*,*,#17147,.T.);
#24606=ORIENTED_EDGE('',*,*,#17135,.F.);
#24607=ORIENTED_EDGE('',*,*,#17088,.T.);
#24608=ORIENTED_EDGE('',*,*,#17151,.F.);
#24609=ORIENTED_EDGE('',*,*,#17159,.T.);
#24610=ORIENTED_EDGE('',*,*,#17134,.F.);
#24611=ORIENTED_EDGE('',*,*,#17159,.F.);
#24612=ORIENTED_EDGE('',*,*,#17153,.F.);
#24613=ORIENTED_EDGE('',*,*,#17158,.F.);
#25349=CONICAL_SURFACE('',#28657,2.65,0.785398163397453);
#25350=CONICAL_SURFACE('',#28674,3.85000000000001,0.78539816339744);
#25351=CONICAL_SURFACE('',#28676,3.85000000000001,0.78539816339744);
#25352=CONICAL_SURFACE('',#28694,11.85,0.785398163397442);
#25353=CONICAL_SURFACE('',#28704,3.85000000000001,0.78539816339744);
#25354=CONICAL_SURFACE('',#28728,3.85000000000002,0.785398163397439);
#25355=CONICAL_SURFACE('',#28729,2.65,0.785398163397453);
#25356=CONICAL_SURFACE('',#28731,2.65,0.785398163397453);
#25357=CONICAL_SURFACE('',#28737,2.65,0.785398163397453);
#25358=CONICAL_SURFACE('',#28745,8.15,0.785398163397451);
#25359=CONICAL_SURFACE('',#28763,3.85000000000001,0.78539816339744);
#25360=CONICAL_SURFACE('',#28775,8.15,0.785398163397448);
#25361=CONICAL_SURFACE('',#28820,6.355,0.785398163397448);
#25362=CONICAL_SURFACE('',#28824,6.355,0.785398163397448);
#25363=CONICAL_SURFACE('',#28828,10.15,0.785398163397448);
#25364=CONICAL_SURFACE('',#28833,9.85,0.785398163397448);
#25365=CONICAL_SURFACE('',#28834,10.15,0.785398163397448);
#25366=CONICAL_SURFACE('',#28838,9.85,0.785398163397448);
#25367=CONICAL_SURFACE('',#28841,11.85,0.785398163397442);
#25368=CONICAL_SURFACE('',#28843,5.15,0.785398163397438);
#25369=CONICAL_SURFACE('',#28847,3.85000000000002,0.785398163397439);
#25370=CONICAL_SURFACE('',#28850,8.15,0.785398163397448);
#25371=CONICAL_SURFACE('',#28856,8.15,0.785398163397451);
#25372=CONICAL_SURFACE('',#28860,5.15,0.785398163397438);
#25373=CONICAL_SURFACE('',#28863,1.4,0.785398163397447);
#25374=CONICAL_SURFACE('',#28866,1.4,0.785398163397447);
#25375=CONICAL_SURFACE('',#28868,1.4,0.785398163397447);
#25376=CONICAL_SURFACE('',#28871,1.4,0.785398163397447);
#25377=CONICAL_SURFACE('',#28880,1.35,0.785398163397446);
#25378=CONICAL_SURFACE('',#28881,1.35,0.785398163397446);
#25379=CONICAL_SURFACE('',#28884,1.35,0.785398163397455);
#25380=CONICAL_SURFACE('',#28887,1.35,0.785398163397455);
#26466=ADVANCED_FACE('',(#3653),#143,.T.);
#26467=ADVANCED_FACE('',(#3654),#741,.T.);
#26468=ADVANCED_FACE('',(#3655),#742,.T.);
#26469=ADVANCED_FACE('',(#3656),#144,.T.);
#26470=ADVANCED_FACE('',(#3657),#2426,.F.);
#26471=ADVANCED_FACE('',(#3658),#2427,.F.);
#26472=ADVANCED_FACE('',(#3659),#743,.F.);
#26473=ADVANCED_FACE('',(#3660),#744,.T.);
#26474=ADVANCED_FACE('',(#3661),#2428,.F.);
#26475=ADVANCED_FACE('',(#3662),#2429,.T.);
#26476=ADVANCED_FACE('',(#3663),#2430,.T.);
#26477=ADVANCED_FACE('',(#3664),#745,.T.);
#26478=ADVANCED_FACE('',(#3665),#2431,.T.);
#26479=ADVANCED_FACE('',(#3666),#2432,.F.);
#26480=ADVANCED_FACE('',(#3667),#746,.T.);
#26481=ADVANCED_FACE('',(#3668),#136,.T.);
#26482=ADVANCED_FACE('',(#3669),#747,.T.);
#26483=ADVANCED_FACE('',(#3670),#137,.T.);
#26484=ADVANCED_FACE('',(#3671),#748,.T.);
#26485=ADVANCED_FACE('',(#3672),#749,.T.);
#26486=ADVANCED_FACE('',(#3673),#750,.T.);
#26487=ADVANCED_FACE('',(#3674),#751,.T.);
#26488=ADVANCED_FACE('',(#3675),#752,.T.);
#26489=ADVANCED_FACE('',(#3676),#145,.T.);
#26490=ADVANCED_FACE('',(#3677),#753,.T.);
#26491=ADVANCED_FACE('',(#3678),#754,.T.);
#26492=ADVANCED_FACE('',(#3679),#755,.T.);
#26493=ADVANCED_FACE('',(#3680),#756,.T.);
#26494=ADVANCED_FACE('',(#3681),#2433,.T.);
#26495=ADVANCED_FACE('',(#3682,#887,#888,#889,#890),#2434,.F.);
#26496=ADVANCED_FACE('',(#3683,#891),#2435,.F.);
#26497=ADVANCED_FACE('',(#3684),#2436,.F.);
#26498=ADVANCED_FACE('',(#3685),#2437,.F.);
#26499=ADVANCED_FACE('',(#3686),#146,.T.);
#26500=ADVANCED_FACE('',(#3687),#757,.F.);
#26501=ADVANCED_FACE('',(#3688,#892),#2438,.F.);
#26502=ADVANCED_FACE('',(#3689),#147,.T.);
#26503=ADVANCED_FACE('',(#3690),#148,.T.);
#26504=ADVANCED_FACE('',(#3691),#758,.F.);
#26505=ADVANCED_FACE('',(#3692,#893),#2439,.F.);
#26506=ADVANCED_FACE('',(#3693),#149,.T.);
#26507=ADVANCED_FACE('',(#3694),#150,.T.);
#26508=ADVANCED_FACE('',(#3695),#759,.F.);
#26509=ADVANCED_FACE('',(#3696),#151,.T.);
#26510=ADVANCED_FACE('',(#3697),#760,.F.);
#26511=ADVANCED_FACE('',(#3698),#138,.T.);
#26512=ADVANCED_FACE('',(#3699),#139,.T.);
#26513=ADVANCED_FACE('',(#3700),#761,.T.);
#26514=ADVANCED_FACE('',(#3701),#762,.T.);
#26515=ADVANCED_FACE('',(#3702),#152,.T.);
#26516=ADVANCED_FACE('',(#3703),#153,.T.);
#26517=ADVANCED_FACE('',(#3704),#763,.T.);
#26518=ADVANCED_FACE('',(#3705),#2440,.F.);
#26519=ADVANCED_FACE('',(#3706),#2441,.T.);
#26520=ADVANCED_FACE('',(#3707),#764,.T.);
#26521=ADVANCED_FACE('',(#3708),#765,.T.);
#26522=ADVANCED_FACE('',(#3709),#140,.T.);
#26523=ADVANCED_FACE('',(#3710),#766,.F.);
#26524=ADVANCED_FACE('',(#3711),#2442,.T.);
#26525=ADVANCED_FACE('',(#3712),#154,.T.);
#26526=ADVANCED_FACE('',(#3713,#894),#767,.T.);
#26527=ADVANCED_FACE('',(#3714),#768,.T.);
#26528=ADVANCED_FACE('',(#3715),#769,.T.);
#26529=ADVANCED_FACE('',(#3716),#141,.T.);
#26530=ADVANCED_FACE('',(#3717),#155,.T.);
#26531=ADVANCED_FACE('',(#3718),#2443,.F.);
#26532=ADVANCED_FACE('',(#3719),#770,.F.);
#26533=ADVANCED_FACE('',(#3720),#771,.T.);
#26534=ADVANCED_FACE('',(#3721),#2444,.F.);
#26535=ADVANCED_FACE('',(#3722),#156,.T.);
#26536=ADVANCED_FACE('',(#3723,#895,#896,#897),#2445,.T.);
#26537=ADVANCED_FACE('',(#3724),#772,.F.);
#26538=ADVANCED_FACE('',(#3725),#157,.T.);
#26539=ADVANCED_FACE('',(#3726),#773,.F.);
#26540=ADVANCED_FACE('',(#3727),#158,.T.);
#26541=ADVANCED_FACE('',(#3728),#774,.F.);
#26542=ADVANCED_FACE('',(#3729),#159,.T.);
#26543=ADVANCED_FACE('',(#3730),#775,.T.);
#26544=ADVANCED_FACE('',(#3731),#776,.F.);
#26545=ADVANCED_FACE('',(#3732),#777,.T.);
#26546=ADVANCED_FACE('',(#3733,#898,#899,#900,#901),#2446,.F.);
#26547=ADVANCED_FACE('',(#3734),#160,.T.);
#26548=ADVANCED_FACE('',(#3735),#778,.F.);
#26549=ADVANCED_FACE('',(#3736),#161,.T.);
#26550=ADVANCED_FACE('',(#3737),#779,.F.);
#26551=ADVANCED_FACE('',(#3738),#2447,.T.);
#26552=ADVANCED_FACE('',(#3739),#162,.T.);
#26553=ADVANCED_FACE('',(#3740),#2448,.F.);
#26554=ADVANCED_FACE('',(#3741),#2449,.T.);
#26555=ADVANCED_FACE('',(#3742),#163,.T.);
#26556=ADVANCED_FACE('',(#3743,#902,#903,#904,#905,#906,#907),#2450,.T.);
#26557=ADVANCED_FACE('',(#3744),#780,.T.);
#26558=ADVANCED_FACE('',(#3745),#164,.T.);
#26559=ADVANCED_FACE('',(#3746),#165,.T.);
#26560=ADVANCED_FACE('',(#3747),#166,.T.);
#26561=ADVANCED_FACE('',(#3748),#167,.T.);
#26562=ADVANCED_FACE('',(#3749),#781,.T.);
#26563=ADVANCED_FACE('',(#3750),#782,.T.);
#26564=ADVANCED_FACE('',(#3751),#2451,.T.);
#26565=ADVANCED_FACE('',(#3752),#25349,.F.);
#26566=ADVANCED_FACE('',(#3753),#2452,.F.);
#26567=ADVANCED_FACE('',(#3754),#2453,.T.);
#26568=ADVANCED_FACE('',(#3755),#168,.T.);
#26569=ADVANCED_FACE('',(#3756),#2454,.F.);
#26570=ADVANCED_FACE('',(#3757),#169,.T.);
#26571=ADVANCED_FACE('',(#3758),#2455,.F.);
#26572=ADVANCED_FACE('',(#3759),#783,.T.);
#26573=ADVANCED_FACE('',(#3760),#2456,.T.);
#26574=ADVANCED_FACE('',(#3761),#2457,.T.);
#26575=ADVANCED_FACE('',(#3762),#2458,.T.);
#26576=ADVANCED_FACE('',(#3763),#25350,.T.);
#26577=ADVANCED_FACE('',(#3764),#25351,.T.);
#26578=ADVANCED_FACE('',(#3765,#908,#909,#910,#911,#912),#2459,.F.);
#26579=ADVANCED_FACE('',(#3766),#784,.F.);
#26580=ADVANCED_FACE('',(#3767),#2460,.F.);
#26581=ADVANCED_FACE('',(#3768),#2461,.T.);
#26582=ADVANCED_FACE('',(#3769),#2462,.T.);
#26583=ADVANCED_FACE('',(#3770),#785,.F.);
#26584=ADVANCED_FACE('',(#3771),#25352,.T.);
#26585=ADVANCED_FACE('',(#3772,#913),#2463,.T.);
#26586=ADVANCED_FACE('',(#3773),#25353,.T.);
#26587=ADVANCED_FACE('',(#3774),#786,.F.);
#26588=ADVANCED_FACE('',(#3775),#2464,.T.);
#26589=ADVANCED_FACE('',(#3776),#787,.F.);
#26590=ADVANCED_FACE('',(#3777),#788,.F.);
#26591=ADVANCED_FACE('',(#3778),#2465,.T.);
#26592=ADVANCED_FACE('',(#3779),#2466,.F.);
#26593=ADVANCED_FACE('',(#3780),#2467,.F.);
#26594=ADVANCED_FACE('',(#3781),#2468,.T.);
#26595=ADVANCED_FACE('',(#3782),#789,.F.);
#26596=ADVANCED_FACE('',(#3783),#790,.F.);
#26597=ADVANCED_FACE('',(#3784),#2469,.T.);
#26598=ADVANCED_FACE('',(#3785),#25354,.T.);
#26599=ADVANCED_FACE('',(#3786),#25355,.F.);
#26600=ADVANCED_FACE('',(#3787),#25356,.F.);
#26601=ADVANCED_FACE('',(#3788),#2470,.T.);
#26602=ADVANCED_FACE('',(#3789),#791,.F.);
#26603=ADVANCED_FACE('',(#3790),#25357,.F.);
#26604=ADVANCED_FACE('',(#3791),#2471,.T.);
#26605=ADVANCED_FACE('',(#3792),#2472,.T.);
#26606=ADVANCED_FACE('',(#3793),#792,.T.);
#26607=ADVANCED_FACE('',(#3794),#793,.T.);
#26608=ADVANCED_FACE('',(#3795),#2473,.T.);
#26609=ADVANCED_FACE('',(#3796),#2474,.T.);
#26610=ADVANCED_FACE('',(#3797),#25358,.F.);
#26611=ADVANCED_FACE('',(#3798),#794,.F.);
#26612=ADVANCED_FACE('',(#3799),#2475,.T.);
#26613=ADVANCED_FACE('',(#3800),#2476,.T.);
#26614=ADVANCED_FACE('',(#3801),#2477,.T.);
#26615=ADVANCED_FACE('',(#3802),#2478,.T.);
#26616=ADVANCED_FACE('',(#3803),#2479,.T.);
#26617=ADVANCED_FACE('',(#3804),#795,.F.);
#26618=ADVANCED_FACE('',(#3805),#2480,.F.);
#26619=ADVANCED_FACE('',(#3806),#796,.F.);
#26620=ADVANCED_FACE('',(#3807),#797,.T.);
#26621=ADVANCED_FACE('',(#3808),#2481,.T.);
#26622=ADVANCED_FACE('',(#3809),#25359,.T.);
#26623=ADVANCED_FACE('',(#3810),#2482,.T.);
#26624=ADVANCED_FACE('',(#3811),#2483,.T.);
#26625=ADVANCED_FACE('',(#3812),#2484,.T.);
#26626=ADVANCED_FACE('',(#3813),#798,.T.);
#26627=ADVANCED_FACE('',(#3814),#799,.T.);
#26628=ADVANCED_FACE('',(#3815),#800,.F.);
#26629=ADVANCED_FACE('',(#3816),#2485,.T.);
#26630=ADVANCED_FACE('',(#3817),#2486,.T.);
#26631=ADVANCED_FACE('',(#3818),#25360,.F.);
#26632=ADVANCED_FACE('',(#3819),#2487,.T.);
#26633=ADVANCED_FACE('',(#3820),#2488,.T.);
#26634=ADVANCED_FACE('',(#3821),#2489,.T.);
#26635=ADVANCED_FACE('',(#3822),#2490,.T.);
#26636=ADVANCED_FACE('',(#3823),#287,.T.);
#26637=ADVANCED_FACE('',(#3824),#288,.T.);
#26638=ADVANCED_FACE('',(#3825),#2491,.T.);
#26639=ADVANCED_FACE('',(#3826),#289,.T.);
#26640=ADVANCED_FACE('',(#3827),#290,.T.);
#26641=ADVANCED_FACE('',(#3828),#2492,.T.);
#26642=ADVANCED_FACE('',(#3829),#2493,.F.);
#26643=ADVANCED_FACE('',(#3830),#2494,.T.);
#26644=ADVANCED_FACE('',(#3831),#2495,.T.);
#26645=ADVANCED_FACE('',(#3832),#2496,.T.);
#26646=ADVANCED_FACE('',(#3833),#2497,.T.);
#26647=ADVANCED_FACE('',(#3834),#2498,.T.);
#26648=ADVANCED_FACE('',(#3835),#2499,.T.);
#26649=ADVANCED_FACE('',(#3836),#2500,.T.);
#26650=ADVANCED_FACE('',(#3837),#2501,.T.);
#26651=ADVANCED_FACE('',(#3838),#2502,.T.);
#26652=ADVANCED_FACE('',(#3839),#2503,.T.);
#26653=ADVANCED_FACE('',(#3840),#2504,.T.);
#26654=ADVANCED_FACE('',(#3841),#291,.T.);
#26655=ADVANCED_FACE('',(#3842),#292,.T.);
#26656=ADVANCED_FACE('',(#3843),#293,.T.);
#26657=ADVANCED_FACE('',(#3844),#294,.T.);
#26658=ADVANCED_FACE('',(#3845),#295,.T.);
#26659=ADVANCED_FACE('',(#3846),#296,.T.);
#26660=ADVANCED_FACE('',(#3847),#297,.T.);
#26661=ADVANCED_FACE('',(#3848),#298,.T.);
#26662=ADVANCED_FACE('',(#3849),#299,.T.);
#26663=ADVANCED_FACE('',(#3850),#300,.T.);
#26664=ADVANCED_FACE('',(#3851),#301,.T.);
#26665=ADVANCED_FACE('',(#3852),#302,.T.);
#26666=ADVANCED_FACE('',(#3853),#303,.T.);
#26667=ADVANCED_FACE('',(#3854),#304,.T.);
#26668=ADVANCED_FACE('',(#3855),#305,.T.);
#26669=ADVANCED_FACE('',(#3856),#306,.T.);
#26670=ADVANCED_FACE('',(#3857),#307,.T.);
#26671=ADVANCED_FACE('',(#3858),#308,.T.);
#26672=ADVANCED_FACE('',(#3859,#914),#2505,.F.);
#26673=ADVANCED_FACE('',(#3860),#2506,.T.);
#26674=ADVANCED_FACE('',(#3861),#2507,.T.);
#26675=ADVANCED_FACE('',(#3862),#2508,.T.);
#26676=ADVANCED_FACE('',(#3863),#2509,.T.);
#26677=ADVANCED_FACE('',(#3864),#2510,.T.);
#26678=ADVANCED_FACE('',(#3865,#915),#2511,.F.);
#26679=ADVANCED_FACE('',(#3866),#801,.F.);
#26680=ADVANCED_FACE('',(#3867,#916),#2512,.F.);
#26681=ADVANCED_FACE('',(#3868),#802,.F.);
#26682=ADVANCED_FACE('',(#3869),#803,.F.);
#26683=ADVANCED_FACE('',(#3870),#804,.F.);
#26684=ADVANCED_FACE('',(#3871),#2513,.F.);
#26685=ADVANCED_FACE('',(#3872),#2514,.F.);
#26686=ADVANCED_FACE('',(#3873),#2515,.F.);
#26687=ADVANCED_FACE('',(#3874),#805,.F.);
#26688=ADVANCED_FACE('',(#3875),#2516,.T.);
#26689=ADVANCED_FACE('',(#3876),#2517,.T.);
#26690=ADVANCED_FACE('',(#3877),#2518,.T.);
#26691=ADVANCED_FACE('',(#3878),#2519,.T.);
#26692=ADVANCED_FACE('',(#3879),#2520,.F.);
#26693=ADVANCED_FACE('',(#3880),#2521,.T.);
#26694=ADVANCED_FACE('',(#3881),#2522,.T.);
#26695=ADVANCED_FACE('',(#3882),#2523,.F.);
#26696=ADVANCED_FACE('',(#3883),#25361,.F.);
#26697=ADVANCED_FACE('',(#3884,#917),#2524,.T.);
#26698=ADVANCED_FACE('',(#3885),#25362,.F.);
#26699=ADVANCED_FACE('',(#3886,#918),#2525,.F.);
#26700=ADVANCED_FACE('',(#3887),#25363,.T.);
#26701=ADVANCED_FACE('',(#3888),#806,.T.);
#26702=ADVANCED_FACE('',(#3889),#2526,.F.);
#26703=ADVANCED_FACE('',(#3890),#25364,.T.);
#26704=ADVANCED_FACE('',(#3891),#25365,.T.);
#26705=ADVANCED_FACE('',(#3892),#807,.T.);
#26706=ADVANCED_FACE('',(#3893),#25366,.T.);
#26707=ADVANCED_FACE('',(#3894),#2527,.T.);
#26708=ADVANCED_FACE('',(#3895),#25367,.T.);
#26709=ADVANCED_FACE('',(#3896),#2528,.T.);
#26710=ADVANCED_FACE('',(#3897),#25368,.F.);
#26711=ADVANCED_FACE('',(#3898),#2529,.T.);
#26712=ADVANCED_FACE('',(#3899),#2530,.T.);
#26713=ADVANCED_FACE('',(#3900),#25369,.T.);
#26714=ADVANCED_FACE('',(#3901),#2531,.T.);
#26715=ADVANCED_FACE('',(#3902),#2532,.T.);
#26716=ADVANCED_FACE('',(#3903),#25370,.F.);
#26717=ADVANCED_FACE('',(#3904),#808,.F.);
#26718=ADVANCED_FACE('',(#3905),#809,.F.);
#26719=ADVANCED_FACE('',(#3906),#2533,.T.);
#26720=ADVANCED_FACE('',(#3907),#25371,.F.);
#26721=ADVANCED_FACE('',(#3908),#2534,.T.);
#26722=ADVANCED_FACE('',(#3909),#2535,.T.);
#26723=ADVANCED_FACE('',(#3910),#2536,.T.);
#26724=ADVANCED_FACE('',(#3911),#25372,.F.);
#26725=ADVANCED_FACE('',(#3912),#2537,.T.);
#26726=ADVANCED_FACE('',(#3913),#2538,.T.);
#26727=ADVANCED_FACE('',(#3914),#25373,.T.);
#26728=ADVANCED_FACE('',(#3915),#2539,.T.);
#26729=ADVANCED_FACE('',(#3916),#25374,.T.);
#26730=ADVANCED_FACE('',(#3917),#25375,.T.);
#26731=ADVANCED_FACE('',(#3918),#2540,.T.);
#26732=ADVANCED_FACE('',(#3919),#25376,.T.);
#26733=ADVANCED_FACE('',(#3920),#810,.T.);
#26734=ADVANCED_FACE('',(#3921),#2541,.T.);
#26735=ADVANCED_FACE('',(#3922),#811,.T.);
#26736=ADVANCED_FACE('',(#3923),#2542,.T.);
#26737=ADVANCED_FACE('',(#3924),#2543,.T.);
#26738=ADVANCED_FACE('',(#3925),#25377,.T.);
#26739=ADVANCED_FACE('',(#3926),#25378,.T.);
#26740=ADVANCED_FACE('',(#3927),#2544,.T.);
#26741=ADVANCED_FACE('',(#3928),#25379,.T.);
#26742=ADVANCED_FACE('',(#3929),#2545,.T.);
#26743=ADVANCED_FACE('',(#3930),#25380,.T.);
#26744=ADVANCED_FACE('',(#3931),#2546,.T.);
#26745=ADVANCED_FACE('',(#3932),#812,.T.);
#26746=ADVANCED_FACE('',(#3933),#813,.T.);
#26747=ADVANCED_FACE('',(#3934),#2547,.T.);
#26885=CLOSED_SHELL('',(#26466,#26467,#26468,#26469,#26470,#26471,#26472,
#26473,#26474,#26475,#26476,#26477,#26478,#26479,#26480,#26481,#26482,#26483,
#26484,#26485,#26486,#26487,#26488,#26489,#26490,#26491,#26492,#26493,#26494,
#26495,#26496,#26497,#26498,#26499,#26500,#26501,#26502,#26503,#26504,#26505,
#26506,#26507,#26508,#26509,#26510,#26511,#26512,#26513,#26514,#26515,#26516,
#26517,#26518,#26519,#26520,#26521,#26522,#26523,#26524,#26525,#26526,#26527,
#26528,#26529,#26530,#26531,#26532,#26533,#26534,#26535,#26536,#26537,#26538,
#26539,#26540,#26541,#26542,#26543,#26544,#26545,#26546,#26547,#26548,#26549,
#26550,#26551,#26552,#26553,#26554,#26555,#26556,#26557,#26558,#26559,#26560,
#26561,#26562,#26563,#26564,#26565,#26566,#26567,#26568,#26569,#26570,#26571,
#26572,#26573,#26574,#26575,#26576,#26577,#26578,#26579,#26580,#26581,#26582,
#26583,#26584,#26585,#26586,#26587,#26588,#26589,#26590,#26591,#26592,#26593,
#26594,#26595,#26596,#26597,#26598,#26599,#26600,#26601,#26602,#26603,#26604,
#26605,#26606,#26607,#26608,#26609,#26610,#26611,#26612,#26613,#26614,#26615,
#26616,#26617,#26618,#26619,#26620,#26621,#26622,#26623,#26624,#26625,#26626,
#26627,#26628,#26629,#26630,#26631,#26632,#26633,#26634,#26635,#26636,#26637,
#26638,#26639,#26640,#26641,#26642,#26643,#26644,#26645,#26646,#26647,#26648,
#26649,#26650,#26651,#26652,#26653,#26654,#26655,#26656,#26657,#26658,#26659,
#26660,#26661,#26662,#26663,#26664,#26665,#26666,#26667,#26668,#26669,#26670,
#26671,#26672,#26673,#26674,#26675,#26676,#26677,#26678,#26679,#26680,#26681,
#26682,#26683,#26684,#26685,#26686,#26687,#26688,#26689,#26690,#26691,#26692,
#26693,#26694,#26695,#26696,#26697,#26698,#26699,#26700,#26701,#26702,#26703,
#26704,#26705,#26706,#26707,#26708,#26709,#26710,#26711,#26712,#26713,#26714,
#26715,#26716,#26717,#26718,#26719,#26720,#26721,#26722,#26723,#26724,#26725,
#26726,#26727,#26728,#26729,#26730,#26731,#26732,#26733,#26734,#26735,#26736,
#26737,#26738,#26739,#26740,#26741,#26742,#26743,#26744,#26745,#26746,#26747));
#28396=AXIS2_PLACEMENT_3D('',#63930,#33654,#33655);
#28397=AXIS2_PLACEMENT_3D('',#63931,#33656,#33657);
#28398=AXIS2_PLACEMENT_3D('',#63934,#33658,#33659);
#28399=AXIS2_PLACEMENT_3D('',#63936,#33660,#33661);
#28400=AXIS2_PLACEMENT_3D('',#63951,#33662,#33663);
#28401=AXIS2_PLACEMENT_3D('',#63966,#33664,#33665);
#28402=AXIS2_PLACEMENT_3D('',#63970,#33667,#33668);
#28403=AXIS2_PLACEMENT_3D('',#63986,#33670,#33671);
#28404=AXIS2_PLACEMENT_3D('',#63987,#33672,#33673);
#28405=AXIS2_PLACEMENT_3D('',#63991,#33675,#33676);
#28406=AXIS2_PLACEMENT_3D('',#63995,#33678,#33679);
#28407=AXIS2_PLACEMENT_3D('',#64010,#33680,#33681);
#28408=AXIS2_PLACEMENT_3D('',#64012,#33682,#33683);
#28409=AXIS2_PLACEMENT_3D('',#64013,#33684,#33685);
#28410=AXIS2_PLACEMENT_3D('',#64014,#33686,#33687);
#28411=AXIS2_PLACEMENT_3D('',#64015,#33688,#33689);
#28412=AXIS2_PLACEMENT_3D('',#64021,#33693,#33694);
#28413=AXIS2_PLACEMENT_3D('',#64029,#33698,#33699);
#28414=AXIS2_PLACEMENT_3D('',#64031,#33701,#33702);
#28415=AXIS2_PLACEMENT_3D('',#64033,#33703,#33704);
#28416=AXIS2_PLACEMENT_3D('',#64037,#33707,#33708);
#28417=AXIS2_PLACEMENT_3D('',#64038,#33709,#33710);
#28418=AXIS2_PLACEMENT_3D('',#64041,#33711,#33712);
#28419=AXIS2_PLACEMENT_3D('',#64045,#33714,#33715);
#28420=AXIS2_PLACEMENT_3D('',#64048,#33717,#33718);
#28421=AXIS2_PLACEMENT_3D('',#64049,#33719,#33720);
#28422=AXIS2_PLACEMENT_3D('',#64059,#33726,#33727);
#28423=AXIS2_PLACEMENT_3D('',#64065,#33731,#33732);
#28424=AXIS2_PLACEMENT_3D('',#64069,#33735,#33736);
#28425=AXIS2_PLACEMENT_3D('',#64072,#33737,#33738);
#28426=AXIS2_PLACEMENT_3D('',#64076,#33740,#33741);
#28427=AXIS2_PLACEMENT_3D('',#64078,#33742,#33743);
#28428=AXIS2_PLACEMENT_3D('',#64080,#33745,#33746);
#28429=AXIS2_PLACEMENT_3D('',#64086,#33750,#33751);
#28430=AXIS2_PLACEMENT_3D('',#64096,#33757,#33758);
#28431=AXIS2_PLACEMENT_3D('',#64098,#33759,#33760);
#28432=AXIS2_PLACEMENT_3D('',#64101,#33762,#33763);
#28433=AXIS2_PLACEMENT_3D('',#64102,#33764,#33765);
#28434=AXIS2_PLACEMENT_3D('',#64104,#33766,#33767);
#28435=AXIS2_PLACEMENT_3D('',#64106,#33768,#33769);
#28436=AXIS2_PLACEMENT_3D('',#64107,#33770,#33771);
#28437=AXIS2_PLACEMENT_3D('',#64108,#33772,#33773);
#28438=AXIS2_PLACEMENT_3D('',#64111,#33775,#33776);
#28439=AXIS2_PLACEMENT_3D('',#64112,#33777,#33778);
#28440=AXIS2_PLACEMENT_3D('',#64114,#33779,#33780);
#28441=AXIS2_PLACEMENT_3D('',#64115,#33781,#33782);
#28442=AXIS2_PLACEMENT_3D('',#64116,#33783,#33784);
#28443=AXIS2_PLACEMENT_3D('',#64121,#33786,#33787);
#28444=AXIS2_PLACEMENT_3D('',#64124,#33789,#33790);
#28445=AXIS2_PLACEMENT_3D('',#64125,#33791,#33792);
#28446=AXIS2_PLACEMENT_3D('',#64128,#33795,#33796);
#28447=AXIS2_PLACEMENT_3D('',#64131,#33798,#33799);
#28448=AXIS2_PLACEMENT_3D('',#64132,#33800,#33801);
#28449=AXIS2_PLACEMENT_3D('',#64137,#33804,#33805);
#28450=AXIS2_PLACEMENT_3D('',#64138,#33806,#33807);
#28451=AXIS2_PLACEMENT_3D('',#64141,#33809,#33810);
#28452=AXIS2_PLACEMENT_3D('',#64142,#33811,#33812);
#28453=AXIS2_PLACEMENT_3D('',#64144,#33813,#33814);
#28454=AXIS2_PLACEMENT_3D('',#64145,#33815,#33816);
#28455=AXIS2_PLACEMENT_3D('',#64146,#33817,#33818);
#28456=AXIS2_PLACEMENT_3D('',#64147,#33819,#33820);
#28457=AXIS2_PLACEMENT_3D('',#64149,#33822,#33823);
#28458=AXIS2_PLACEMENT_3D('',#64154,#33826,#33827);
#28459=AXIS2_PLACEMENT_3D('',#64155,#33828,#33829);
#28460=AXIS2_PLACEMENT_3D('',#64158,#33832,#33833);
#28461=AXIS2_PLACEMENT_3D('',#64161,#33835,#33836);
#28462=AXIS2_PLACEMENT_3D('',#64162,#33837,#33838);
#28463=AXIS2_PLACEMENT_3D('',#64166,#33841,#33842);
#28464=AXIS2_PLACEMENT_3D('',#64170,#33844,#33845);
#28465=AXIS2_PLACEMENT_3D('',#64174,#33847,#33848);
#28466=AXIS2_PLACEMENT_3D('',#64178,#33850,#33851);
#28467=AXIS2_PLACEMENT_3D('',#64181,#33853,#33854);
#28468=AXIS2_PLACEMENT_3D('',#64183,#33855,#33856);
#28469=AXIS2_PLACEMENT_3D('',#64185,#33857,#33858);
#28470=AXIS2_PLACEMENT_3D('',#64187,#33859,#33860);
#28471=AXIS2_PLACEMENT_3D('',#64189,#33861,#33862);
#28472=AXIS2_PLACEMENT_3D('',#64190,#33863,#33864);
#28473=AXIS2_PLACEMENT_3D('',#64201,#33870,#33871);
#28474=AXIS2_PLACEMENT_3D('',#64202,#33872,#33873);
#28475=AXIS2_PLACEMENT_3D('',#64204,#33875,#33876);
#28476=AXIS2_PLACEMENT_3D('',#64206,#33878,#33879);
#28477=AXIS2_PLACEMENT_3D('',#64208,#33880,#33881);
#28478=AXIS2_PLACEMENT_3D('',#64210,#33882,#33883);
#28479=AXIS2_PLACEMENT_3D('',#64211,#33884,#33885);
#28480=AXIS2_PLACEMENT_3D('',#64212,#33886,#33887);
#28481=AXIS2_PLACEMENT_3D('',#64214,#33888,#33889);
#28482=AXIS2_PLACEMENT_3D('',#64216,#33891,#33892);
#28483=AXIS2_PLACEMENT_3D('',#64218,#33893,#33894);
#28484=AXIS2_PLACEMENT_3D('',#64219,#33895,#33896);
#28485=AXIS2_PLACEMENT_3D('',#64220,#33897,#33898);
#28486=AXIS2_PLACEMENT_3D('',#64221,#33899,#33900);
#28487=AXIS2_PLACEMENT_3D('',#64223,#33901,#33902);
#28488=AXIS2_PLACEMENT_3D('',#64225,#33903,#33904);
#28489=AXIS2_PLACEMENT_3D('',#64226,#33905,#33906);
#28490=AXIS2_PLACEMENT_3D('',#64227,#33907,#33908);
#28491=AXIS2_PLACEMENT_3D('',#64229,#33909,#33910);
#28492=AXIS2_PLACEMENT_3D('',#64231,#33912,#33913);
#28493=AXIS2_PLACEMENT_3D('',#64233,#33914,#33915);
#28494=AXIS2_PLACEMENT_3D('',#64234,#33916,#33917);
#28495=AXIS2_PLACEMENT_3D('',#64235,#33918,#33919);
#28496=AXIS2_PLACEMENT_3D('',#64236,#33920,#33921);
#28497=AXIS2_PLACEMENT_3D('',#64238,#33922,#33923);
#28498=AXIS2_PLACEMENT_3D('',#64239,#33924,#33925);
#28499=AXIS2_PLACEMENT_3D('',#64240,#33926,#33927);
#28500=AXIS2_PLACEMENT_3D('',#64243,#33929,#33930);
#28501=AXIS2_PLACEMENT_3D('',#64244,#33931,#33932);
#28502=AXIS2_PLACEMENT_3D('',#64246,#33933,#33934);
#28503=AXIS2_PLACEMENT_3D('',#64247,#33935,#33936);
#28504=AXIS2_PLACEMENT_3D('',#64248,#33937,#33938);
#28505=AXIS2_PLACEMENT_3D('',#64251,#33940,#33941);
#28506=AXIS2_PLACEMENT_3D('',#64252,#33942,#33943);
#28507=AXIS2_PLACEMENT_3D('',#64255,#33944,#33945);
#28508=AXIS2_PLACEMENT_3D('',#64257,#33946,#33947);
#28509=AXIS2_PLACEMENT_3D('',#64258,#33948,#33949);
#28510=AXIS2_PLACEMENT_3D('',#64259,#33950,#33951);
#28511=AXIS2_PLACEMENT_3D('',#64262,#33952,#33953);
#28512=AXIS2_PLACEMENT_3D('',#64264,#33954,#33955);
#28513=AXIS2_PLACEMENT_3D('',#64265,#33956,#33957);
#28514=AXIS2_PLACEMENT_3D('',#64266,#33958,#33959);
#28515=AXIS2_PLACEMENT_3D('',#64269,#33962,#33963);
#28516=AXIS2_PLACEMENT_3D('',#64284,#33966,#33967);
#28517=AXIS2_PLACEMENT_3D('',#64301,#33968,#33969);
#28518=AXIS2_PLACEMENT_3D('',#64302,#33970,#33971);
#28519=AXIS2_PLACEMENT_3D('',#64303,#33972,#33973);
#28520=AXIS2_PLACEMENT_3D('',#64320,#33974,#33975);
#28521=AXIS2_PLACEMENT_3D('',#64321,#33976,#33977);
#28522=AXIS2_PLACEMENT_3D('',#64322,#33978,#33979);
#28523=AXIS2_PLACEMENT_3D('',#64337,#33982,#33983);
#28524=AXIS2_PLACEMENT_3D('',#64339,#33984,#33985);
#28525=AXIS2_PLACEMENT_3D('',#64343,#33987,#33988);
#28526=AXIS2_PLACEMENT_3D('',#64345,#33990,#33991);
#28527=AXIS2_PLACEMENT_3D('',#64355,#33997,#33998);
#28528=AXIS2_PLACEMENT_3D('',#64371,#34000,#34001);
#28529=AXIS2_PLACEMENT_3D('',#64373,#34003,#34004);
#28530=AXIS2_PLACEMENT_3D('',#64385,#34006,#34007);
#28531=AXIS2_PLACEMENT_3D('',#64388,#34009,#34010);
#28532=AXIS2_PLACEMENT_3D('',#64390,#34012,#34013);
#28533=AXIS2_PLACEMENT_3D('',#64391,#34014,#34015);
#28534=AXIS2_PLACEMENT_3D('',#64392,#34016,#34017);
#28535=AXIS2_PLACEMENT_3D('',#64394,#34018,#34019);
#28536=AXIS2_PLACEMENT_3D('',#64398,#34021,#34022);
#28537=AXIS2_PLACEMENT_3D('',#64409,#34024,#34025);
#28538=AXIS2_PLACEMENT_3D('',#64420,#34027,#34028);
#28539=AXIS2_PLACEMENT_3D('',#64422,#34030,#34031);
#28540=AXIS2_PLACEMENT_3D('',#64424,#34032,#34033);
#28541=AXIS2_PLACEMENT_3D('',#64430,#34037,#34038);
#28542=AXIS2_PLACEMENT_3D('',#64432,#34039,#34040);
#28543=AXIS2_PLACEMENT_3D('',#64433,#34041,#34042);
#28544=AXIS2_PLACEMENT_3D('',#64434,#34043,#34044);
#28545=AXIS2_PLACEMENT_3D('',#64436,#34045,#34046);
#28546=AXIS2_PLACEMENT_3D('',#64440,#34048,#34049);
#28547=AXIS2_PLACEMENT_3D('',#64444,#34051,#34052);
#28548=AXIS2_PLACEMENT_3D('',#64448,#34054,#34055);
#28549=AXIS2_PLACEMENT_3D('',#64452,#34057,#34058);
#28550=AXIS2_PLACEMENT_3D('',#64454,#34060,#34061);
#28551=AXIS2_PLACEMENT_3D('',#64465,#34063,#34064);
#28552=AXIS2_PLACEMENT_3D('',#64467,#34065,#34066);
#28553=AXIS2_PLACEMENT_3D('',#64469,#34068,#34069);
#28554=AXIS2_PLACEMENT_3D('',#64484,#34071,#34072);
#28555=AXIS2_PLACEMENT_3D('',#64486,#34074,#34075);
#28556=AXIS2_PLACEMENT_3D('',#64487,#34076,#34077);
#28557=AXIS2_PLACEMENT_3D('',#64488,#34078,#34079);
#28558=AXIS2_PLACEMENT_3D('',#64490,#34080,#34081);
#28559=AXIS2_PLACEMENT_3D('',#64491,#34082,#34083);
#28560=AXIS2_PLACEMENT_3D('',#64492,#34084,#34085);
#28561=AXIS2_PLACEMENT_3D('',#64494,#34086,#34087);
#28562=AXIS2_PLACEMENT_3D('',#64500,#34091,#34092);
#28563=AXIS2_PLACEMENT_3D('',#64504,#34094,#34095);
#28564=AXIS2_PLACEMENT_3D('',#64515,#34097,#34098);
#28565=AXIS2_PLACEMENT_3D('',#64526,#34100,#34101);
#28566=AXIS2_PLACEMENT_3D('',#64528,#34103,#34104);
#28567=AXIS2_PLACEMENT_3D('',#64552,#34106,#34107);
#28568=AXIS2_PLACEMENT_3D('',#64572,#34111,#34112);
#28569=AXIS2_PLACEMENT_3D('',#64574,#34113,#34114);
#28570=AXIS2_PLACEMENT_3D('',#64576,#34115,#34116);
#28571=AXIS2_PLACEMENT_3D('',#64578,#34117,#34118);
#28572=AXIS2_PLACEMENT_3D('',#64579,#34119,#34120);
#28573=AXIS2_PLACEMENT_3D('',#64580,#34121,#34122);
#28574=AXIS2_PLACEMENT_3D('',#64583,#34123,#34124);
#28575=AXIS2_PLACEMENT_3D('',#64599,#34133,#34134);
#28576=AXIS2_PLACEMENT_3D('',#64601,#34135,#34136);
#28577=AXIS2_PLACEMENT_3D('',#64603,#34137,#34138);
#28578=AXIS2_PLACEMENT_3D('',#64604,#34139,#34140);
#28579=AXIS2_PLACEMENT_3D('',#64606,#34141,#34142);
#28580=AXIS2_PLACEMENT_3D('',#64608,#34144,#34145);
#28581=AXIS2_PLACEMENT_3D('',#64610,#34146,#34147);
#28582=AXIS2_PLACEMENT_3D('',#64612,#34148,#34149);
#28583=AXIS2_PLACEMENT_3D('',#64613,#34150,#34151);
#28584=AXIS2_PLACEMENT_3D('',#64614,#34152,#34153);
#28585=AXIS2_PLACEMENT_3D('',#64616,#34154,#34155);
#28586=AXIS2_PLACEMENT_3D('',#64618,#34157,#34158);
#28587=AXIS2_PLACEMENT_3D('',#64620,#34159,#34160);
#28588=AXIS2_PLACEMENT_3D('',#64622,#34161,#34162);
#28589=AXIS2_PLACEMENT_3D('',#64623,#34163,#34164);
#28590=AXIS2_PLACEMENT_3D('',#64624,#34165,#34166);
#28591=AXIS2_PLACEMENT_3D('',#64626,#34167,#34168);
#28592=AXIS2_PLACEMENT_3D('',#64628,#34170,#34171);
#28593=AXIS2_PLACEMENT_3D('',#64640,#34172,#34173);
#28594=AXIS2_PLACEMENT_3D('',#64642,#34174,#34175);
#28595=AXIS2_PLACEMENT_3D('',#64643,#34176,#34177);
#28596=AXIS2_PLACEMENT_3D('',#64644,#34178,#34179);
#28597=AXIS2_PLACEMENT_3D('',#64667,#34181,#34182);
#28598=AXIS2_PLACEMENT_3D('',#64671,#34184,#34185);
#28599=AXIS2_PLACEMENT_3D('',#64692,#34187,#34188);
#28600=AXIS2_PLACEMENT_3D('',#64694,#34189,#34190);
#28601=AXIS2_PLACEMENT_3D('',#64696,#34192,#34193);
#28602=AXIS2_PLACEMENT_3D('',#64728,#34194,#34195);
#28603=AXIS2_PLACEMENT_3D('',#64731,#34197,#34198);
#28604=AXIS2_PLACEMENT_3D('',#64732,#34199,#34200);
#28605=AXIS2_PLACEMENT_3D('',#64748,#34209,#34210);
#28606=AXIS2_PLACEMENT_3D('',#64750,#34211,#34212);
#28607=AXIS2_PLACEMENT_3D('',#64752,#34213,#34214);
#28608=AXIS2_PLACEMENT_3D('',#64754,#34215,#34216);
#28609=AXIS2_PLACEMENT_3D('',#64755,#34217,#34218);
#28610=AXIS2_PLACEMENT_3D('',#64757,#34219,#34220);
#28611=AXIS2_PLACEMENT_3D('',#64758,#34221,#34222);
#28612=AXIS2_PLACEMENT_3D('',#64759,#34223,#34224);
#28613=AXIS2_PLACEMENT_3D('',#64763,#34226,#34227);
#28614=AXIS2_PLACEMENT_3D('',#64764,#34228,#34229);
#28615=AXIS2_PLACEMENT_3D('',#64765,#34230,#34231);
#28616=AXIS2_PLACEMENT_3D('',#64783,#34232,#34233);
#28617=AXIS2_PLACEMENT_3D('',#64799,#34234,#34235);
#28618=AXIS2_PLACEMENT_3D('',#64800,#34236,#34237);
#28619=AXIS2_PLACEMENT_3D('',#64804,#34239,#34240);
#28620=AXIS2_PLACEMENT_3D('',#64806,#34242,#34243);
#28621=AXIS2_PLACEMENT_3D('',#64812,#34247,#34248);
#28622=AXIS2_PLACEMENT_3D('',#64829,#34249,#34250);
#28623=AXIS2_PLACEMENT_3D('',#64844,#34251,#34252);
#28624=AXIS2_PLACEMENT_3D('',#64848,#34254,#34255);
#28625=AXIS2_PLACEMENT_3D('',#64850,#34257,#34258);
#28626=AXIS2_PLACEMENT_3D('',#64854,#34261,#34262);
#28627=AXIS2_PLACEMENT_3D('',#64856,#34263,#34264);
#28628=AXIS2_PLACEMENT_3D('',#64857,#34265,#34266);
#28629=AXIS2_PLACEMENT_3D('',#64858,#34267,#34268);
#28630=AXIS2_PLACEMENT_3D('',#64859,#34269,#34270);
#28631=AXIS2_PLACEMENT_3D('',#64861,#34271,#34272);
#28632=AXIS2_PLACEMENT_3D('',#64865,#34274,#34275);
#28633=AXIS2_PLACEMENT_3D('',#64869,#34277,#34278);
#28634=AXIS2_PLACEMENT_3D('',#64872,#34280,#34281);
#28635=AXIS2_PLACEMENT_3D('',#64874,#34282,#34283);
#28636=AXIS2_PLACEMENT_3D('',#64876,#34284,#34285);
#28637=AXIS2_PLACEMENT_3D('',#64878,#34286,#34287);
#28638=AXIS2_PLACEMENT_3D('',#64880,#34288,#34289);
#28639=AXIS2_PLACEMENT_3D('',#64900,#34301,#34302);
#28640=AXIS2_PLACEMENT_3D('',#64902,#34303,#34304);
#28641=AXIS2_PLACEMENT_3D('',#64903,#34305,#34306);
#28642=AXIS2_PLACEMENT_3D('',#64904,#34307,#34308);
#28643=AXIS2_PLACEMENT_3D('',#64905,#34309,#34310);
#28644=AXIS2_PLACEMENT_3D('',#64906,#34311,#34312);
#28645=AXIS2_PLACEMENT_3D('',#64907,#34313,#34314);
#28646=AXIS2_PLACEMENT_3D('',#64908,#34315,#34316);
#28647=AXIS2_PLACEMENT_3D('',#64909,#34317,#34318);
#28648=AXIS2_PLACEMENT_3D('',#64910,#34319,#34320);
#28649=AXIS2_PLACEMENT_3D('',#64911,#34321,#34322);
#28650=AXIS2_PLACEMENT_3D('',#64912,#34323,#34324);
#28651=AXIS2_PLACEMENT_3D('',#64913,#34325,#34326);
#28652=AXIS2_PLACEMENT_3D('',#64916,#34327,#34328);
#28653=AXIS2_PLACEMENT_3D('',#64920,#34330,#34331);
#28654=AXIS2_PLACEMENT_3D('',#64940,#34335,#34336);
#28655=AXIS2_PLACEMENT_3D('',#64941,#34337,#34338);
#28656=AXIS2_PLACEMENT_3D('',#64943,#34340,#34341);
#28657=AXIS2_PLACEMENT_3D('',#64949,#34345,#34346);
#28658=AXIS2_PLACEMENT_3D('',#64954,#34347,#34348);
#28659=AXIS2_PLACEMENT_3D('',#64955,#34349,#34350);
#28660=AXIS2_PLACEMENT_3D('',#64970,#34357,#34358);
#28661=AXIS2_PLACEMENT_3D('',#64972,#34360,#34361);
#28662=AXIS2_PLACEMENT_3D('',#64973,#34362,#34363);
#28663=AXIS2_PLACEMENT_3D('',#64974,#34364,#34365);
#28664=AXIS2_PLACEMENT_3D('',#64977,#34367,#34368);
#28665=AXIS2_PLACEMENT_3D('',#64978,#34369,#34370);
#28666=AXIS2_PLACEMENT_3D('',#64979,#34371,#34372);
#28667=AXIS2_PLACEMENT_3D('',#64980,#34373,#34374);
#28668=AXIS2_PLACEMENT_3D('',#64982,#34375,#34376);
#28669=AXIS2_PLACEMENT_3D('',#64984,#34378,#34379);
#28670=AXIS2_PLACEMENT_3D('',#64985,#34380,#34381);
#28671=AXIS2_PLACEMENT_3D('',#64986,#34382,#34383);
#28672=AXIS2_PLACEMENT_3D('',#64992,#34387,#34388);
#28673=AXIS2_PLACEMENT_3D('',#64994,#34390,#34391);
#28674=AXIS2_PLACEMENT_3D('',#65000,#34393,#34394);
#28675=AXIS2_PLACEMENT_3D('',#65014,#34396,#34397);
#28676=AXIS2_PLACEMENT_3D('',#65015,#34398,#34399);
#28677=AXIS2_PLACEMENT_3D('',#65017,#34400,#34401);
#28678=AXIS2_PLACEMENT_3D('',#65030,#34403,#34404);
#28679=AXIS2_PLACEMENT_3D('',#65034,#34406,#34407);
#28680=AXIS2_PLACEMENT_3D('',#65038,#34409,#34410);
#28681=AXIS2_PLACEMENT_3D('',#65042,#34412,#34413);
#28682=AXIS2_PLACEMENT_3D('',#65044,#34415,#34416);
#28683=AXIS2_PLACEMENT_3D('',#65046,#34417,#34418);
#28684=AXIS2_PLACEMENT_3D('',#65050,#34420,#34421);
#28685=AXIS2_PLACEMENT_3D('',#65101,#34427,#34428);
#28686=AXIS2_PLACEMENT_3D('',#65148,#34444,#34445);
#28687=AXIS2_PLACEMENT_3D('',#65149,#34446,#34447);
#28688=AXIS2_PLACEMENT_3D('',#65150,#34448,#34449);
#28689=AXIS2_PLACEMENT_3D('',#65151,#34450,#34451);
#28690=AXIS2_PLACEMENT_3D('',#65157,#34453,#34454);
#28691=AXIS2_PLACEMENT_3D('',#65159,#34456,#34457);
#28692=AXIS2_PLACEMENT_3D('',#65161,#34458,#34459);
#28693=AXIS2_PLACEMENT_3D('',#65164,#34461,#34462);
#28694=AXIS2_PLACEMENT_3D('',#65165,#34463,#34464);
#28695=AXIS2_PLACEMENT_3D('',#65167,#34465,#34466);
#28696=AXIS2_PLACEMENT_3D('',#65169,#34468,#34469);
#28697=AXIS2_PLACEMENT_3D('',#65173,#34471,#34472);
#28698=AXIS2_PLACEMENT_3D('',#65177,#34474,#34475);
#28699=AXIS2_PLACEMENT_3D('',#65181,#34477,#34478);
#28700=AXIS2_PLACEMENT_3D('',#65184,#34480,#34481);
#28701=AXIS2_PLACEMENT_3D('',#65186,#34482,#34483);
#28702=AXIS2_PLACEMENT_3D('',#65190,#34485,#34486);
#28703=AXIS2_PLACEMENT_3D('',#65193,#34488,#34489);
#28704=AXIS2_PLACEMENT_3D('',#65194,#34490,#34491);
#28705=AXIS2_PLACEMENT_3D('',#65207,#34493,#34494);
#28706=AXIS2_PLACEMENT_3D('',#65208,#34495,#34496);
#28707=AXIS2_PLACEMENT_3D('',#65209,#34497,#34498);
#28708=AXIS2_PLACEMENT_3D('',#65210,#34499,#34500);
#28709=AXIS2_PLACEMENT_3D('',#65213,#34502,#34503);
#28710=AXIS2_PLACEMENT_3D('',#65214,#34504,#34505);
#28711=AXIS2_PLACEMENT_3D('',#65216,#34506,#34507);
#28712=AXIS2_PLACEMENT_3D('',#65218,#34509,#34510);
#28713=AXIS2_PLACEMENT_3D('',#65222,#34512,#34513);
#28714=AXIS2_PLACEMENT_3D('',#65225,#34515,#34516);
#28715=AXIS2_PLACEMENT_3D('',#65226,#34517,#34518);
#28716=AXIS2_PLACEMENT_3D('',#65230,#34520,#34521);
#28717=AXIS2_PLACEMENT_3D('',#65233,#34523,#34524);
#28718=AXIS2_PLACEMENT_3D('',#65234,#34525,#34526);
#28719=AXIS2_PLACEMENT_3D('',#65235,#34527,#34528);
#28720=AXIS2_PLACEMENT_3D('',#65236,#34529,#34530);
#28721=AXIS2_PLACEMENT_3D('',#65237,#34531,#34532);
#28722=AXIS2_PLACEMENT_3D('',#65238,#34533,#34534);
#28723=AXIS2_PLACEMENT_3D('',#65239,#34535,#34536);
#28724=AXIS2_PLACEMENT_3D('',#65240,#34537,#34538);
#28725=AXIS2_PLACEMENT_3D('',#65242,#34539,#34540);
#28726=AXIS2_PLACEMENT_3D('',#65243,#34541,#34542);
#28727=AXIS2_PLACEMENT_3D('',#65244,#34543,#34544);
#28728=AXIS2_PLACEMENT_3D('',#65248,#34547,#34548);
#28729=AXIS2_PLACEMENT_3D('',#65251,#34551,#34552);
#28730=AXIS2_PLACEMENT_3D('',#65253,#34553,#34554);
#28731=AXIS2_PLACEMENT_3D('',#65257,#34555,#34556);
#28732=AXIS2_PLACEMENT_3D('',#65258,#34557,#34558);
#28733=AXIS2_PLACEMENT_3D('',#65260,#34559,#34560);
#28734=AXIS2_PLACEMENT_3D('',#65263,#34562,#34563);
#28735=AXIS2_PLACEMENT_3D('',#65264,#34564,#34565);
#28736=AXIS2_PLACEMENT_3D('',#65265,#34566,#34567);
#28737=AXIS2_PLACEMENT_3D('',#65266,#34568,#34569);
#28738=AXIS2_PLACEMENT_3D('',#65270,#34570,#34571);
#28739=AXIS2_PLACEMENT_3D('',#65274,#34574,#34575);
#28740=AXIS2_PLACEMENT_3D('',#65280,#34579,#34580);
#28741=AXIS2_PLACEMENT_3D('',#65301,#34581,#34582);
#28742=AXIS2_PLACEMENT_3D('',#65320,#34583,#34584);
#28743=AXIS2_PLACEMENT_3D('',#65321,#34585,#34586);
#28744=AXIS2_PLACEMENT_3D('',#65322,#34587,#34588);
#28745=AXIS2_PLACEMENT_3D('',#65328,#34593,#34594);
#28746=AXIS2_PLACEMENT_3D('',#65331,#34597,#34598);
#28747=AXIS2_PLACEMENT_3D('',#65333,#34599,#34600);
#28748=AXIS2_PLACEMENT_3D('',#65336,#34602,#34603);
#28749=AXIS2_PLACEMENT_3D('',#65337,#34604,#34605);
#28750=AXIS2_PLACEMENT_3D('',#65343,#34609,#34610);
#28751=AXIS2_PLACEMENT_3D('',#65349,#34614,#34615);
#28752=AXIS2_PLACEMENT_3D('',#65355,#34619,#34620);
#28753=AXIS2_PLACEMENT_3D('',#65363,#34625,#34626);
#28754=AXIS2_PLACEMENT_3D('',#65372,#34631,#34632);
#28755=AXIS2_PLACEMENT_3D('',#65373,#34633,#34634);
#28756=AXIS2_PLACEMENT_3D('',#65374,#34635,#34636);
#28757=AXIS2_PLACEMENT_3D('',#65375,#34637,#34638);
#28758=AXIS2_PLACEMENT_3D('',#65376,#34639,#34640);
#28759=AXIS2_PLACEMENT_3D('',#65377,#34641,#34642);
#28760=AXIS2_PLACEMENT_3D('',#65388,#34643,#34644);
#28761=AXIS2_PLACEMENT_3D('',#65390,#34646,#34647);
#28762=AXIS2_PLACEMENT_3D('',#65392,#34649,#34650);
#28763=AXIS2_PLACEMENT_3D('',#65393,#34651,#34652);
#28764=AXIS2_PLACEMENT_3D('',#65395,#34654,#34655);
#28765=AXIS2_PLACEMENT_3D('',#65397,#34657,#34658);
#28766=AXIS2_PLACEMENT_3D('',#65401,#34661,#34662);
#28767=AXIS2_PLACEMENT_3D('',#65407,#34666,#34667);
#28768=AXIS2_PLACEMENT_3D('',#65409,#34668,#34669);
#28769=AXIS2_PLACEMENT_3D('',#65426,#34670,#34671);
#28770=AXIS2_PLACEMENT_3D('',#65429,#34672,#34673);
#28771=AXIS2_PLACEMENT_3D('',#65430,#34674,#34675);
#28772=AXIS2_PLACEMENT_3D('',#65447,#34676,#34677);
#28773=AXIS2_PLACEMENT_3D('',#65449,#34679,#34680);
#28774=AXIS2_PLACEMENT_3D('',#65451,#34682,#34683);
#28775=AXIS2_PLACEMENT_3D('',#65459,#34684,#34685);
#28776=AXIS2_PLACEMENT_3D('',#65461,#34687,#34688);
#28777=AXIS2_PLACEMENT_3D('',#65464,#34691,#34692);
#28778=AXIS2_PLACEMENT_3D('',#65470,#34696,#34697);
#28779=AXIS2_PLACEMENT_3D('',#65474,#34700,#34701);
#28780=AXIS2_PLACEMENT_3D('',#65500,#34706,#34707);
#28781=AXIS2_PLACEMENT_3D('',#65526,#34712,#34713);
#28782=AXIS2_PLACEMENT_3D('',#65528,#34715,#34716);
#28783=AXIS2_PLACEMENT_3D('',#65529,#34717,#34718);
#28784=AXIS2_PLACEMENT_3D('',#65535,#34722,#34723);
#28785=AXIS2_PLACEMENT_3D('',#65539,#34726,#34727);
#28786=AXIS2_PLACEMENT_3D('',#65543,#34730,#34731);
#28787=AXIS2_PLACEMENT_3D('',#65547,#34734,#34735);
#28788=AXIS2_PLACEMENT_3D('',#65551,#34738,#34739);
#28789=AXIS2_PLACEMENT_3D('',#65555,#34742,#34743);
#28790=AXIS2_PLACEMENT_3D('',#65559,#34746,#34747);
#28791=AXIS2_PLACEMENT_3D('',#65563,#34750,#34751);
#28792=AXIS2_PLACEMENT_3D('',#65567,#34754,#34755);
#28793=AXIS2_PLACEMENT_3D('',#65569,#34757,#34758);
#28794=AXIS2_PLACEMENT_3D('',#65800,#34777,#34778);
#28795=AXIS2_PLACEMENT_3D('',#65801,#34779,#34780);
#28796=AXIS2_PLACEMENT_3D('',#65807,#34784,#34785);
#28797=AXIS2_PLACEMENT_3D('',#65811,#34788,#34789);
#28798=AXIS2_PLACEMENT_3D('',#65815,#34792,#34793);
#28799=AXIS2_PLACEMENT_3D('',#65817,#34795,#34796);
#28800=AXIS2_PLACEMENT_3D('',#65818,#34797,#34798);
#28801=AXIS2_PLACEMENT_3D('',#65820,#34799,#34800);
#28802=AXIS2_PLACEMENT_3D('',#65821,#34801,#34802);
#28803=AXIS2_PLACEMENT_3D('',#65823,#34804,#34805);
#28804=AXIS2_PLACEMENT_3D('',#65825,#34806,#34807);
#28805=AXIS2_PLACEMENT_3D('',#65826,#34808,#34809);
#28806=AXIS2_PLACEMENT_3D('',#65828,#34811,#34812);
#28807=AXIS2_PLACEMENT_3D('',#65830,#34814,#34815);
#28808=AXIS2_PLACEMENT_3D('',#65832,#34817,#34818);
#28809=AXIS2_PLACEMENT_3D('',#65834,#34820,#34821);
#28810=AXIS2_PLACEMENT_3D('',#65836,#34823,#34824);
#28811=AXIS2_PLACEMENT_3D('',#65837,#34825,#34826);
#28812=AXIS2_PLACEMENT_3D('',#65838,#34827,#34828);
#28813=AXIS2_PLACEMENT_3D('',#65842,#34831,#34832);
#28814=AXIS2_PLACEMENT_3D('',#65844,#34834,#34835);
#28815=AXIS2_PLACEMENT_3D('',#65846,#34837,#34838);
#28816=AXIS2_PLACEMENT_3D('',#65848,#34840,#34841);
#28817=AXIS2_PLACEMENT_3D('',#65852,#34844,#34845);
#28818=AXIS2_PLACEMENT_3D('',#65855,#34848,#34849);
#28819=AXIS2_PLACEMENT_3D('',#65856,#34850,#34851);
#28820=AXIS2_PLACEMENT_3D('',#65857,#34852,#34853);
#28821=AXIS2_PLACEMENT_3D('',#65859,#34854,#34855);
#28822=AXIS2_PLACEMENT_3D('',#65861,#34857,#34858);
#28823=AXIS2_PLACEMENT_3D('',#65863,#34859,#34860);
#28824=AXIS2_PLACEMENT_3D('',#65864,#34861,#34862);
#28825=AXIS2_PLACEMENT_3D('',#65866,#34863,#34864);
#28826=AXIS2_PLACEMENT_3D('',#65868,#34866,#34867);
#28827=AXIS2_PLACEMENT_3D('',#65870,#34868,#34869);
#28828=AXIS2_PLACEMENT_3D('',#65871,#34870,#34871);
#28829=AXIS2_PLACEMENT_3D('',#65874,#34873,#34874);
#28830=AXIS2_PLACEMENT_3D('',#65875,#34875,#34876);
#28831=AXIS2_PLACEMENT_3D('',#65878,#34878,#34879);
#28832=AXIS2_PLACEMENT_3D('',#65879,#34880,#34881);
#28833=AXIS2_PLACEMENT_3D('',#65880,#34882,#34883);
#28834=AXIS2_PLACEMENT_3D('',#65882,#34885,#34886);
#28835=AXIS2_PLACEMENT_3D('',#65885,#34888,#34889);
#28836=AXIS2_PLACEMENT_3D('',#65886,#34890,#34891);
#28837=AXIS2_PLACEMENT_3D('',#65888,#34892,#34893);
#28838=AXIS2_PLACEMENT_3D('',#65890,#34895,#34896);
#28839=AXIS2_PLACEMENT_3D('',#65892,#34898,#34899);
#28840=AXIS2_PLACEMENT_3D('',#65894,#34900,#34901);
#28841=AXIS2_PLACEMENT_3D('',#65896,#34903,#34904);
#28842=AXIS2_PLACEMENT_3D('',#65898,#34906,#34907);
#28843=AXIS2_PLACEMENT_3D('',#65900,#34909,#34910);
#28844=AXIS2_PLACEMENT_3D('',#65902,#34912,#34913);
#28845=AXIS2_PLACEMENT_3D('',#65903,#34914,#34915);
#28846=AXIS2_PLACEMENT_3D('',#65904,#34916,#34917);
#28847=AXIS2_PLACEMENT_3D('',#65906,#34919,#34920);
#28848=AXIS2_PLACEMENT_3D('',#65908,#34922,#34923);
#28849=AXIS2_PLACEMENT_3D('',#65909,#34924,#34925);
#28850=AXIS2_PLACEMENT_3D('',#65911,#34927,#34928);
#28851=AXIS2_PLACEMENT_3D('',#65919,#34929,#34930);
#28852=AXIS2_PLACEMENT_3D('',#65920,#34931,#34932);
#28853=AXIS2_PLACEMENT_3D('',#65921,#34933,#34934);
#28854=AXIS2_PLACEMENT_3D('',#65922,#34935,#34936);
#28855=AXIS2_PLACEMENT_3D('',#65923,#34937,#34938);
#28856=AXIS2_PLACEMENT_3D('',#65925,#34940,#34941);
#28857=AXIS2_PLACEMENT_3D('',#65927,#34943,#34944);
#28858=AXIS2_PLACEMENT_3D('',#65928,#34945,#34946);
#28859=AXIS2_PLACEMENT_3D('',#65929,#34947,#34948);
#28860=AXIS2_PLACEMENT_3D('',#65931,#34950,#34951);
#28861=AXIS2_PLACEMENT_3D('',#65933,#34953,#34954);
#28862=AXIS2_PLACEMENT_3D('',#65934,#34955,#34956);
#28863=AXIS2_PLACEMENT_3D('',#65940,#34960,#34961);
#28864=AXIS2_PLACEMENT_3D('',#65943,#34963,#34964);
#28865=AXIS2_PLACEMENT_3D('',#65944,#34965,#34966);
#28866=AXIS2_PLACEMENT_3D('',#65948,#34969,#34970);
#28867=AXIS2_PLACEMENT_3D('',#65949,#34971,#34972);
#28868=AXIS2_PLACEMENT_3D('',#65950,#34973,#34974);
#28869=AXIS2_PLACEMENT_3D('',#65953,#34976,#34977);
#28870=AXIS2_PLACEMENT_3D('',#65954,#34978,#34979);
#28871=AXIS2_PLACEMENT_3D('',#65958,#34982,#34983);
#28872=AXIS2_PLACEMENT_3D('',#65959,#34984,#34985);
#28873=AXIS2_PLACEMENT_3D('',#65960,#34986,#34987);
#28874=AXIS2_PLACEMENT_3D('',#65963,#34989,#34990);
#28875=AXIS2_PLACEMENT_3D('',#65964,#34991,#34992);
#28876=AXIS2_PLACEMENT_3D('',#65968,#34995,#34996);
#28877=AXIS2_PLACEMENT_3D('',#65971,#34998,#34999);
#28878=AXIS2_PLACEMENT_3D('',#65972,#35000,#35001);
#28879=AXIS2_PLACEMENT_3D('',#65976,#35004,#35005);
#28880=AXIS2_PLACEMENT_3D('',#65977,#35006,#35007);
#28881=AXIS2_PLACEMENT_3D('',#65979,#35009,#35010);
#28882=AXIS2_PLACEMENT_3D('',#65982,#35012,#35013);
#28883=AXIS2_PLACEMENT_3D('',#65983,#35014,#35015);
#28884=AXIS2_PLACEMENT_3D('',#65987,#35018,#35019);
#28885=AXIS2_PLACEMENT_3D('',#65989,#35021,#35022);
#28886=AXIS2_PLACEMENT_3D('',#65990,#35023,#35024);
#28887=AXIS2_PLACEMENT_3D('',#65992,#35026,#35027);
#28888=AXIS2_PLACEMENT_3D('',#65994,#35029,#35030);
#28889=AXIS2_PLACEMENT_3D('',#65995,#35031,#35032);
#28890=AXIS2_PLACEMENT_3D('',#65997,#35034,#35035);
#28891=AXIS2_PLACEMENT_3D('',#65999,#35037,#35038);
#33654=DIRECTION('axis',(0.,0.,1.));
#33655=DIRECTION('refdir',(1.,0.,0.));
#33656=DIRECTION('center_axis',(0.,-1.,0.));
#33657=DIRECTION('ref_axis',(0.,0.,-1.));
#33658=DIRECTION('center_axis',(0.,1.,0.));
#33659=DIRECTION('ref_axis',(-1.,0.,0.));
#33660=DIRECTION('center_axis',(0.,1.,0.));
#33661=DIRECTION('ref_axis',(-1.,0.,0.));
#33662=DIRECTION('center_axis',(0.,-1.,0.));
#33663=DIRECTION('ref_axis',(-1.,0.,0.));
#33664=DIRECTION('center_axis',(0.,1.,0.));
#33665=DIRECTION('ref_axis',(-0.396879513944558,0.,-0.917870716065793));
#33666=DIRECTION('',(0.,1.,0.));
#33667=DIRECTION('center_axis',(0.,-1.,0.));
#33668=DIRECTION('ref_axis',(-0.396879513944558,0.,-0.917870716065793));
#33669=DIRECTION('',(0.,-1.,0.));
#33670=DIRECTION('center_axis',(0.,1.,0.));
#33671=DIRECTION('ref_axis',(-0.396879513944558,0.,-0.917870716065793));
#33672=DIRECTION('center_axis',(0.,-1.,0.));
#33673=DIRECTION('ref_axis',(-0.396879513944558,0.,0.917870716065793));
#33674=DIRECTION('',(0.,1.,0.));
#33675=DIRECTION('center_axis',(0.,-1.,0.));
#33676=DIRECTION('ref_axis',(-0.396879513944558,0.,0.917870716065793));
#33677=DIRECTION('',(0.,-1.,0.));
#33678=DIRECTION('center_axis',(0.,1.,0.));
#33679=DIRECTION('ref_axis',(-0.396879513944558,0.,0.917870716065793));
#33680=DIRECTION('center_axis',(0.,1.,0.));
#33681=DIRECTION('ref_axis',(0.,0.,1.));
#33682=DIRECTION('center_axis',(0.,-1.,0.));
#33683=DIRECTION('ref_axis',(-1.,0.,0.));
#33684=DIRECTION('center_axis',(0.,-1.,0.));
#33685=DIRECTION('ref_axis',(-1.,0.,0.));
#33686=DIRECTION('center_axis',(0.,1.,0.));
#33687=DIRECTION('ref_axis',(-1.,0.,0.));
#33688=DIRECTION('center_axis',(1.,0.,0.));
#33689=DIRECTION('ref_axis',(0.,1.,0.));
#33690=DIRECTION('',(0.,0.,1.));
#33691=DIRECTION('',(0.,1.,0.));
#33692=DIRECTION('',(0.,0.,1.));
#33693=DIRECTION('center_axis',(0.,1.,0.));
#33694=DIRECTION('ref_axis',(-1.,0.,0.));
#33695=DIRECTION('',(0.,0.,1.));
#33696=DIRECTION('',(1.,0.,0.));
#33697=DIRECTION('',(0.,0.,1.));
#33698=DIRECTION('center_axis',(0.,1.,0.));
#33699=DIRECTION('ref_axis',(0.66778348591556,0.,-0.744355570905776));
#33700=DIRECTION('',(-1.,0.,0.));
#33701=DIRECTION('center_axis',(0.,1.,0.));
#33702=DIRECTION('ref_axis',(1.,0.,0.));
#33703=DIRECTION('center_axis',(0.,1.,0.));
#33704=DIRECTION('ref_axis',(1.,0.,0.));
#33705=DIRECTION('',(0.,1.,0.));
#33706=DIRECTION('',(0.,1.,0.));
#33707=DIRECTION('center_axis',(0.,-1.,0.));
#33708=DIRECTION('ref_axis',(1.,0.,0.));
#33709=DIRECTION('center_axis',(0.,0.,-1.));
#33710=DIRECTION('ref_axis',(-0.70710678118655,0.707106781186545,0.));
#33711=DIRECTION('center_axis',(0.707106781186546,0.,0.707106781186549));
#33712=DIRECTION('ref_axis',(-0.707106781186549,1.96261557335472E-16,0.707106781186546));
#33713=DIRECTION('',(0.,0.,1.));
#33714=DIRECTION('center_axis',(0.70710678118655,0.,-0.707106781186545));
#33715=DIRECTION('ref_axis',(-0.707106781186545,-6.54205191118238E-17,-0.70710678118655));
#33716=DIRECTION('',(0.,0.,-1.));
#33717=DIRECTION('center_axis',(-0.707106781186551,0.,0.707106781186544));
#33718=DIRECTION('ref_axis',(-0.707106781186544,-6.54205191118236E-17,-0.707106781186551));
#33719=DIRECTION('center_axis',(0.,-1.,0.));
#33720=DIRECTION('ref_axis',(-1.,0.,0.));
#33721=DIRECTION('',(-1.,0.,0.));
#33722=DIRECTION('',(0.,0.,-1.));
#33723=DIRECTION('',(1.,0.,0.));
#33724=DIRECTION('',(0.,0.,1.));
#33725=DIRECTION('',(1.,0.,0.));
#33726=DIRECTION('center_axis',(-0.70710678118655,0.,0.707106781186545));
#33727=DIRECTION('ref_axis',(0.707106781186545,0.,0.70710678118655));
#33728=DIRECTION('',(0.,-1.,0.));
#33729=DIRECTION('',(-0.707106781186548,0.,-0.707106781186548));
#33730=DIRECTION('',(0.,1.,0.));
#33731=DIRECTION('center_axis',(-1.,0.,0.));
#33732=DIRECTION('ref_axis',(0.,-1.,0.));
#33733=DIRECTION('',(0.,1.,0.));
#33734=DIRECTION('',(0.,0.,-1.));
#33735=DIRECTION('center_axis',(0.,0.,1.));
#33736=DIRECTION('ref_axis',(-0.70710678118655,-0.707106781186545,0.));
#33737=DIRECTION('center_axis',(0.70710678118655,0.,-0.707106781186545));
#33738=DIRECTION('ref_axis',(-0.707106781186545,6.54205191118238E-17,-0.70710678118655));
#33739=DIRECTION('',(0.,0.,-1.));
#33740=DIRECTION('center_axis',(0.707106781186546,0.,0.707106781186549));
#33741=DIRECTION('ref_axis',(-0.707106781186549,-1.96261557335472E-16,0.707106781186546));
#33742=DIRECTION('center_axis',(-0.707106781186547,0.,0.707106781186548));
#33743=DIRECTION('ref_axis',(-0.707106781186548,6.5420519111824E-17,-0.707106781186547));
#33744=DIRECTION('',(0.,0.,1.));
#33745=DIRECTION('center_axis',(-0.70710678118655,0.,0.707106781186545));
#33746=DIRECTION('ref_axis',(0.707106781186545,0.,0.70710678118655));
#33747=DIRECTION('',(0.,1.,0.));
#33748=DIRECTION('',(-0.707106781186545,0.,-0.70710678118655));
#33749=DIRECTION('',(0.,-1.,0.));
#33750=DIRECTION('center_axis',(0.,1.,0.));
#33751=DIRECTION('ref_axis',(1.,0.,0.));
#33752=DIRECTION('',(-1.,0.,0.));
#33753=DIRECTION('',(0.,0.,-1.));
#33754=DIRECTION('',(-1.,0.,0.));
#33755=DIRECTION('',(0.,0.,-1.));
#33756=DIRECTION('',(1.,0.,0.));
#33757=DIRECTION('center_axis',(-1.,0.,0.));
#33758=DIRECTION('ref_axis',(0.,-0.707106781186545,-0.70710678118655));
#33759=DIRECTION('center_axis',(0.707106781186546,0.,0.707106781186549));
#33760=DIRECTION('ref_axis',(0.70710678118655,6.54205191118238E-17,-0.707106781186546));
#33761=DIRECTION('',(1.,0.,0.));
#33762=DIRECTION('center_axis',(1.,-5.9211894646675E-15,0.));
#33763=DIRECTION('ref_axis',(0.,0.,-1.));
#33764=DIRECTION('center_axis',(-0.40824829046386,-0.40824829046386,-0.816496580927729));
#33765=DIRECTION('ref_axis',(0.577350269189629,0.577350269189626,-0.577350269189622));
#33766=DIRECTION('center_axis',(1.,0.,1.1842378929335E-14));
#33767=DIRECTION('ref_axis',(0.,1.,0.));
#33768=DIRECTION('center_axis',(0.,2.96059473233374E-15,-1.));
#33769=DIRECTION('ref_axis',(1.,0.,0.));
#33770=DIRECTION('center_axis',(0.,1.,0.));
#33771=DIRECTION('ref_axis',(0.,0.,-1.));
#33772=DIRECTION('center_axis',(0.,0.,-1.));
#33773=DIRECTION('ref_axis',(0.707106781186545,0.70710678118655,0.));
#33774=DIRECTION('',(0.,0.,-1.));
#33775=DIRECTION('center_axis',(-0.707106781186548,-2.09345661157836E-15,
-0.707106781186548));
#33776=DIRECTION('ref_axis',(-0.707106781186548,-2.09345661157836E-15,0.707106781186548));
#33777=DIRECTION('center_axis',(-0.408248290463859,-0.816496580927727,0.408248290463866));
#33778=DIRECTION('ref_axis',(0.577350269189622,-0.577350269189625,-0.577350269189631));
#33779=DIRECTION('center_axis',(-2.96059473233375E-15,0.,-1.));
#33780=DIRECTION('ref_axis',(0.,-1.,0.));
#33781=DIRECTION('center_axis',(0.,-1.,2.96059473233375E-15));
#33782=DIRECTION('ref_axis',(1.,0.,0.));
#33783=DIRECTION('center_axis',(-1.,0.,0.));
#33784=DIRECTION('ref_axis',(0.,-0.707106781186548,-0.707106781186547));
#33785=DIRECTION('',(-1.,0.,0.));
#33786=DIRECTION('center_axis',(0.707106781186552,0.707106781186543,-4.18691322315676E-15));
#33787=DIRECTION('ref_axis',(0.707106781186543,-0.707106781186552,4.18691322315681E-15));
#33788=DIRECTION('',(1.,0.,0.));
#33789=DIRECTION('center_axis',(-0.707106781186552,0.707106781186543,0.));
#33790=DIRECTION('ref_axis',(0.707106781186543,0.707106781186552,0.));
#33791=DIRECTION('center_axis',(0.,-1.,0.));
#33792=DIRECTION('ref_axis',(0.707106781186546,0.,-0.707106781186549));
#33793=DIRECTION('',(0.,-1.,0.));
#33794=DIRECTION('',(0.,1.,0.));
#33795=DIRECTION('center_axis',(0.,0.,1.));
#33796=DIRECTION('ref_axis',(0.707106781186545,-0.70710678118655,0.));
#33797=DIRECTION('',(0.,0.,1.));
#33798=DIRECTION('center_axis',(-0.707106781186548,2.09345661157836E-15,
-0.707106781186548));
#33799=DIRECTION('ref_axis',(0.707106781186548,-2.09345661157836E-15,-0.707106781186548));
#33800=DIRECTION('center_axis',(0.,1.,0.));
#33801=DIRECTION('ref_axis',(-0.707106781186544,0.,-0.707106781186551));
#33802=DIRECTION('',(0.,1.,0.));
#33803=DIRECTION('',(0.,-1.,0.));
#33804=DIRECTION('center_axis',(0.707106781186552,0.707106781186543,0.));
#33805=DIRECTION('ref_axis',(0.707106781186543,-0.707106781186552,0.));
#33806=DIRECTION('center_axis',(1.,0.,0.));
#33807=DIRECTION('ref_axis',(0.,-0.707106781186547,-0.707106781186547));
#33808=DIRECTION('',(1.,0.,0.));
#33809=DIRECTION('center_axis',(-1.,0.,0.));
#33810=DIRECTION('ref_axis',(0.,0.,-1.));
#33811=DIRECTION('center_axis',(0.,0.,-1.));
#33812=DIRECTION('ref_axis',(1.,-1.22464679914735E-16,0.));
#33813=DIRECTION('center_axis',(1.,0.,0.));
#33814=DIRECTION('ref_axis',(0.,0.,-1.));
#33815=DIRECTION('center_axis',(0.,0.,1.));
#33816=DIRECTION('ref_axis',(1.,-6.12323399573677E-17,0.));
#33817=DIRECTION('center_axis',(0.,0.,-1.));
#33818=DIRECTION('ref_axis',(1.,-6.12323399573677E-17,0.));
#33819=DIRECTION('center_axis',(-1.,0.,0.));
#33820=DIRECTION('ref_axis',(0.,0.707106781186547,-0.707106781186547));
#33821=DIRECTION('',(-1.,0.,0.));
#33822=DIRECTION('center_axis',(1.,0.,0.));
#33823=DIRECTION('ref_axis',(0.,0.707106781186548,-0.707106781186547));
#33824=DIRECTION('',(1.,0.,0.));
#33825=DIRECTION('',(-1.,0.,0.));
#33826=DIRECTION('center_axis',(0.70710678118655,-0.707106781186545,0.));
#33827=DIRECTION('ref_axis',(-0.707106781186545,-0.70710678118655,0.));
#33828=DIRECTION('center_axis',(0.,-1.,0.));
#33829=DIRECTION('ref_axis',(0.707106781186546,0.,-0.707106781186549));
#33830=DIRECTION('',(0.,1.,0.));
#33831=DIRECTION('',(0.,-1.,0.));
#33832=DIRECTION('center_axis',(1.,0.,0.));
#33833=DIRECTION('ref_axis',(0.,0.707106781186545,-0.70710678118655));
#33834=DIRECTION('',(-1.,0.,0.));
#33835=DIRECTION('center_axis',(0.707106781186546,0.,0.707106781186549));
#33836=DIRECTION('ref_axis',(0.70710678118655,-6.54205191118238E-17,-0.707106781186546));
#33837=DIRECTION('center_axis',(-0.707106781186546,0.,-0.707106781186549));
#33838=DIRECTION('ref_axis',(-0.707106781186549,0.,0.707106781186546));
#33839=DIRECTION('',(0.,-1.,0.));
#33840=DIRECTION('',(-0.707106781186549,0.,0.707106781186546));
#33841=DIRECTION('center_axis',(0.,0.,1.));
#33842=DIRECTION('ref_axis',(1.,0.,0.));
#33843=DIRECTION('',(0.,-1.,0.));
#33844=DIRECTION('center_axis',(0.,0.,1.));
#33845=DIRECTION('ref_axis',(-0.707106781186548,0.707106781186548,0.));
#33846=DIRECTION('',(-1.,0.,0.));
#33847=DIRECTION('center_axis',(0.,0.,1.));
#33848=DIRECTION('ref_axis',(0.707106781186548,0.707106781186548,0.));
#33849=DIRECTION('',(0.,1.,0.));
#33850=DIRECTION('center_axis',(0.,0.,1.));
#33851=DIRECTION('ref_axis',(0.707106781186548,-0.707106781186548,0.));
#33852=DIRECTION('',(1.,0.,0.));
#33853=DIRECTION('center_axis',(0.,0.,1.));
#33854=DIRECTION('ref_axis',(-0.707106781186548,-0.707106781186548,0.));
#33855=DIRECTION('center_axis',(0.,0.,-1.));
#33856=DIRECTION('ref_axis',(1.,0.,0.));
#33857=DIRECTION('center_axis',(0.,0.,-1.));
#33858=DIRECTION('ref_axis',(1.,0.,0.));
#33859=DIRECTION('center_axis',(0.,0.,-1.));
#33860=DIRECTION('ref_axis',(1.,0.,0.));
#33861=DIRECTION('center_axis',(0.,0.,-1.));
#33862=DIRECTION('ref_axis',(1.,0.,0.));
#33863=DIRECTION('center_axis',(0.,0.,1.));
#33864=DIRECTION('ref_axis',(1.,0.,0.));
#33865=DIRECTION('',(0.,-1.,0.));
#33866=DIRECTION('',(-1.,0.,0.));
#33867=DIRECTION('',(0.,1.,0.));
#33868=DIRECTION('',(1.,0.,0.));
#33869=DIRECTION('',(0.,-1.,0.));
#33870=DIRECTION('center_axis',(0.,0.,-1.));
#33871=DIRECTION('ref_axis',(-1.,1.22464679914735E-16,0.));
#33872=DIRECTION('center_axis',(-1.,0.,0.));
#33873=DIRECTION('ref_axis',(0.,-1.,0.));
#33874=DIRECTION('',(0.,0.,1.));
#33875=DIRECTION('center_axis',(0.,1.,0.));
#33876=DIRECTION('ref_axis',(-1.,0.,0.));
#33877=DIRECTION('',(0.,0.,1.));
#33878=DIRECTION('center_axis',(0.,0.,1.));
#33879=DIRECTION('ref_axis',(1.,0.,0.));
#33880=DIRECTION('center_axis',(0.,0.,-1.));
#33881=DIRECTION('ref_axis',(-1.,0.,0.));
#33882=DIRECTION('center_axis',(0.,-1.,0.));
#33883=DIRECTION('ref_axis',(-1.,0.,0.));
#33884=DIRECTION('center_axis',(0.,0.,1.));
#33885=DIRECTION('ref_axis',(-1.,0.,0.));
#33886=DIRECTION('center_axis',(0.,0.,1.));
#33887=DIRECTION('ref_axis',(1.,0.,0.));
#33888=DIRECTION('center_axis',(0.,0.,1.));
#33889=DIRECTION('ref_axis',(1.,0.,0.));
#33890=DIRECTION('',(0.,0.,1.));
#33891=DIRECTION('center_axis',(0.,0.,-1.));
#33892=DIRECTION('ref_axis',(-1.,0.,0.));
#33893=DIRECTION('center_axis',(0.,0.,1.));
#33894=DIRECTION('ref_axis',(1.,0.,0.));
#33895=DIRECTION('center_axis',(0.,0.,1.));
#33896=DIRECTION('ref_axis',(1.,0.,0.));
#33897=DIRECTION('center_axis',(0.,-1.,0.));
#33898=DIRECTION('ref_axis',(-1.,0.,0.));
#33899=DIRECTION('center_axis',(0.,0.,1.));
#33900=DIRECTION('ref_axis',(1.,0.,0.));
#33901=DIRECTION('center_axis',(0.,0.,-1.));
#33902=DIRECTION('ref_axis',(-1.,0.,0.));
#33903=DIRECTION('center_axis',(0.,-1.,0.));
#33904=DIRECTION('ref_axis',(-1.,0.,0.));
#33905=DIRECTION('center_axis',(0.,0.,1.));
#33906=DIRECTION('ref_axis',(-1.,0.,0.));
#33907=DIRECTION('center_axis',(0.,0.,1.));
#33908=DIRECTION('ref_axis',(1.,0.,0.));
#33909=DIRECTION('center_axis',(0.,0.,1.));
#33910=DIRECTION('ref_axis',(1.,0.,0.));
#33911=DIRECTION('',(0.,0.,1.));
#33912=DIRECTION('center_axis',(0.,0.,-1.));
#33913=DIRECTION('ref_axis',(-1.,0.,0.));
#33914=DIRECTION('center_axis',(0.,0.,1.));
#33915=DIRECTION('ref_axis',(1.,0.,0.));
#33916=DIRECTION('center_axis',(0.,0.,1.));
#33917=DIRECTION('ref_axis',(1.,0.,0.));
#33918=DIRECTION('center_axis',(0.,-1.,0.));
#33919=DIRECTION('ref_axis',(-1.,0.,0.));
#33920=DIRECTION('center_axis',(0.,0.,1.));
#33921=DIRECTION('ref_axis',(1.,0.,0.));
#33922=DIRECTION('center_axis',(0.,-1.,0.));
#33923=DIRECTION('ref_axis',(-1.,0.,0.));
#33924=DIRECTION('center_axis',(0.,0.,1.));
#33925=DIRECTION('ref_axis',(1.,0.,0.));
#33926=DIRECTION('center_axis',(0.,0.,1.));
#33927=DIRECTION('ref_axis',(1.,0.,0.));
#33928=DIRECTION('',(0.,0.,1.));
#33929=DIRECTION('center_axis',(0.,0.,1.));
#33930=DIRECTION('ref_axis',(1.,0.,0.));
#33931=DIRECTION('center_axis',(0.,0.,1.));
#33932=DIRECTION('ref_axis',(1.,0.,0.));
#33933=DIRECTION('center_axis',(0.,-1.,0.));
#33934=DIRECTION('ref_axis',(-1.,0.,0.));
#33935=DIRECTION('center_axis',(0.,0.,1.));
#33936=DIRECTION('ref_axis',(1.,0.,0.));
#33937=DIRECTION('center_axis',(0.,0.,1.));
#33938=DIRECTION('ref_axis',(1.,0.,0.));
#33939=DIRECTION('',(0.,0.,1.));
#33940=DIRECTION('center_axis',(0.,0.,1.));
#33941=DIRECTION('ref_axis',(1.,0.,0.));
#33942=DIRECTION('center_axis',(0.,0.,1.));
#33943=DIRECTION('ref_axis',(1.,0.,0.));
#33944=DIRECTION('center_axis',(0.,-2.368475785867E-14,1.));
#33945=DIRECTION('ref_axis',(-1.,0.,0.));
#33946=DIRECTION('center_axis',(0.,1.,0.));
#33947=DIRECTION('ref_axis',(-0.721328943656992,0.,0.692592632824439));
#33948=DIRECTION('center_axis',(-0.69259263282442,0.,-0.72132894365701));
#33949=DIRECTION('ref_axis',(0.,1.,0.));
#33950=DIRECTION('center_axis',(0.,0.,1.));
#33951=DIRECTION('ref_axis',(1.,0.,0.));
#33952=DIRECTION('center_axis',(-0.692592632824435,-2.10153204267973E-14,
-0.721328943656996));
#33953=DIRECTION('ref_axis',(-0.721328943656996,0.,0.692592632824435));
#33954=DIRECTION('center_axis',(0.,-1.,0.));
#33955=DIRECTION('ref_axis',(-1.,0.,0.));
#33956=DIRECTION('center_axis',(-2.368475785867E-14,0.,1.));
#33957=DIRECTION('ref_axis',(0.,-1.,0.));
#33958=DIRECTION('center_axis',(0.,1.,0.));
#33959=DIRECTION('ref_axis',(-0.927720039574705,0.,0.373276744750471));
#33960=DIRECTION('',(0.,-1.,0.));
#33961=DIRECTION('',(0.,1.,0.));
#33962=DIRECTION('center_axis',(0.,0.,-1.));
#33963=DIRECTION('ref_axis',(-0.707106781186552,-0.707106781186543,0.));
#33964=DIRECTION('',(0.,0.,1.));
#33965=DIRECTION('',(0.,0.,-1.));
#33966=DIRECTION('center_axis',(0.,1.,0.));
#33967=DIRECTION('ref_axis',(0.,0.,1.));
#33968=DIRECTION('center_axis',(0.,1.,0.));
#33969=DIRECTION('ref_axis',(0.853668140319692,0.,-0.52081734437624));
#33970=DIRECTION('center_axis',(0.,-1.,0.));
#33971=DIRECTION('ref_axis',(0.853668140319692,0.,-0.52081734437624));
#33972=DIRECTION('center_axis',(0.,-1.,0.));
#33973=DIRECTION('ref_axis',(0.,0.,-1.));
#33974=DIRECTION('center_axis',(0.,1.,0.));
#33975=DIRECTION('ref_axis',(0.853668140319692,0.,-0.52081734437624));
#33976=DIRECTION('center_axis',(0.,-1.,0.));
#33977=DIRECTION('ref_axis',(0.853668140319692,0.,-0.52081734437624));
#33978=DIRECTION('center_axis',(0.,0.,1.));
#33979=DIRECTION('ref_axis',(-0.707106781186552,0.707106781186543,0.));
#33980=DIRECTION('',(0.,0.,1.));
#33981=DIRECTION('',(0.,0.,-1.));
#33982=DIRECTION('center_axis',(0.,1.,0.));
#33983=DIRECTION('ref_axis',(1.,0.,0.));
#33984=DIRECTION('center_axis',(0.,1.,0.));
#33985=DIRECTION('ref_axis',(1.,0.,0.));
#33986=DIRECTION('',(-1.,0.,0.));
#33987=DIRECTION('center_axis',(0.,-1.,0.));
#33988=DIRECTION('ref_axis',(0.999999998065448,0.,6.22021185913536E-5));
#33989=DIRECTION('',(0.,0.,1.));
#33990=DIRECTION('center_axis',(-1.,0.,0.));
#33991=DIRECTION('ref_axis',(0.,0.,1.));
#33992=DIRECTION('',(0.,-1.,0.));
#33993=DIRECTION('',(0.,-1.,0.));
#33994=DIRECTION('',(0.,0.,-1.));
#33995=DIRECTION('',(0.,1.,0.));
#33996=DIRECTION('',(0.,0.,1.));
#33997=DIRECTION('center_axis',(-1.,0.,0.));
#33998=DIRECTION('ref_axis',(0.,0.707106781186573,-0.707106781186522));
#33999=DIRECTION('',(-1.,0.,0.));
#34000=DIRECTION('center_axis',(1.,0.,0.));
#34001=DIRECTION('ref_axis',(0.,0.,-1.));
#34002=DIRECTION('',(1.,0.,0.));
#34003=DIRECTION('center_axis',(0.,-1.,0.));
#34004=DIRECTION('ref_axis',(-0.710342984735764,0.,-0.703855698305189));
#34005=DIRECTION('',(0.,-1.,0.));
#34006=DIRECTION('center_axis',(0.,-1.,0.));
#34007=DIRECTION('ref_axis',(-0.710342984735764,0.,-0.703855698305189));
#34008=DIRECTION('',(0.,1.,0.));
#34009=DIRECTION('center_axis',(0.,-1.,0.));
#34010=DIRECTION('ref_axis',(-0.999957915114768,0.,0.00917431192661418));
#34011=DIRECTION('',(0.,-1.,0.));
#34012=DIRECTION('center_axis',(-0.815256777504774,-0.411367939544186,0.407593921750192));
#34013=DIRECTION('ref_axis',(-0.579099634547059,0.579124006914431,-0.57381094263079));
#34014=DIRECTION('center_axis',(-0.00917431192660542,0.,-0.999957915114768));
#34015=DIRECTION('ref_axis',(-0.999957915114768,0.,0.00917431192660542));
#34016=DIRECTION('center_axis',(0.,1.,0.));
#34017=DIRECTION('ref_axis',(-1.,0.,0.));
#34018=DIRECTION('center_axis',(0.,-1.,0.));
#34019=DIRECTION('ref_axis',(-1.,0.,0.));
#34020=DIRECTION('',(0.,1.,0.));
#34021=DIRECTION('center_axis',(0.,1.,0.));
#34022=DIRECTION('ref_axis',(-1.,0.,0.));
#34023=DIRECTION('',(0.,-1.,0.));
#34024=DIRECTION('center_axis',(0.,1.,0.));
#34025=DIRECTION('ref_axis',(-1.,0.,0.));
#34026=DIRECTION('',(0.,1.,0.));
#34027=DIRECTION('center_axis',(0.,1.,0.));
#34028=DIRECTION('ref_axis',(-1.,0.,0.));
#34029=DIRECTION('',(0.,1.,0.));
#34030=DIRECTION('center_axis',(0.,1.,0.));
#34031=DIRECTION('ref_axis',(1.,0.,0.));
#34032=DIRECTION('center_axis',(0.,-1.,0.));
#34033=DIRECTION('ref_axis',(-1.07657990266682E-16,0.,1.));
#34034=DIRECTION('',(0.,0.,1.));
#34035=DIRECTION('',(-1.,0.,0.));
#34036=DIRECTION('',(0.,0.,1.));
#34037=DIRECTION('center_axis',(0.,1.,0.));
#34038=DIRECTION('ref_axis',(0.,0.,1.));
#34039=DIRECTION('center_axis',(0.,1.,0.));
#34040=DIRECTION('ref_axis',(-1.07657990266682E-16,0.,1.));
#34041=DIRECTION('center_axis',(0.,0.,1.));
#34042=DIRECTION('ref_axis',(1.,0.,0.));
#34043=DIRECTION('center_axis',(0.,1.,0.));
#34044=DIRECTION('ref_axis',(-1.,0.,0.));
#34045=DIRECTION('center_axis',(0.,1.,0.));
#34046=DIRECTION('ref_axis',(-1.,0.,0.));
#34047=DIRECTION('',(0.,1.,0.));
#34048=DIRECTION('center_axis',(0.,-1.,0.));
#34049=DIRECTION('ref_axis',(-1.,0.,0.));
#34050=DIRECTION('',(0.,1.,0.));
#34051=DIRECTION('center_axis',(0.,-1.,0.));
#34052=DIRECTION('ref_axis',(-1.07657990266682E-16,0.,1.));
#34053=DIRECTION('',(0.,-1.,0.));
#34054=DIRECTION('center_axis',(0.,1.,0.));
#34055=DIRECTION('ref_axis',(-1.,0.,0.));
#34056=DIRECTION('',(0.,-1.,0.));
#34057=DIRECTION('center_axis',(0.,1.,0.));
#34058=DIRECTION('ref_axis',(-1.,0.,0.));
#34059=DIRECTION('',(0.,1.,0.));
#34060=DIRECTION('center_axis',(0.,-1.,0.));
#34061=DIRECTION('ref_axis',(-0.710342984735764,0.,-0.703855698305189));
#34062=DIRECTION('',(0.,-1.,0.));
#34063=DIRECTION('center_axis',(0.,1.,0.));
#34064=DIRECTION('ref_axis',(0.,0.,-1.));
#34065=DIRECTION('center_axis',(0.,1.,0.));
#34066=DIRECTION('ref_axis',(-0.710342984735764,0.,-0.703855698305189));
#34067=DIRECTION('',(0.,-1.,0.));
#34068=DIRECTION('center_axis',(1.,0.,0.));
#34069=DIRECTION('ref_axis',(0.,-0.707106781186573,-0.707106781186522));
#34070=DIRECTION('',(-1.,0.,0.));
#34071=DIRECTION('center_axis',(1.,0.,0.));
#34072=DIRECTION('ref_axis',(0.,-1.,0.));
#34073=DIRECTION('',(1.,0.,0.));
#34074=DIRECTION('center_axis',(-0.815256777504774,0.411367939544186,0.407593921750192));
#34075=DIRECTION('ref_axis',(-0.579099634547059,-0.579124006914431,-0.57381094263079));
#34076=DIRECTION('center_axis',(-0.00917431192660542,0.,-0.999957915114768));
#34077=DIRECTION('ref_axis',(-0.999957915114768,0.,0.00917431192660542));
#34078=DIRECTION('center_axis',(0.,-1.,0.));
#34079=DIRECTION('ref_axis',(0.00458720422654698,0.,0.999989478723343));
#34080=DIRECTION('center_axis',(0.,1.,0.));
#34081=DIRECTION('ref_axis',(-1.07657990266682E-16,0.,1.));
#34082=DIRECTION('center_axis',(0.,0.,-1.));
#34083=DIRECTION('ref_axis',(1.,0.,0.));
#34084=DIRECTION('center_axis',(0.,1.,0.));
#34085=DIRECTION('ref_axis',(1.,0.,0.));
#34086=DIRECTION('center_axis',(0.,1.,0.));
#34087=DIRECTION('ref_axis',(-1.,0.,0.));
#34088=DIRECTION('',(0.,0.,-1.));
#34089=DIRECTION('',(1.,0.,0.));
#34090=DIRECTION('',(0.,0.,-1.));
#34091=DIRECTION('center_axis',(0.,1.,0.));
#34092=DIRECTION('ref_axis',(-1.,0.,0.));
#34093=DIRECTION('',(0.,1.,0.));
#34094=DIRECTION('center_axis',(0.,-1.,0.));
#34095=DIRECTION('ref_axis',(-1.,0.,0.));
#34096=DIRECTION('',(0.,1.,0.));
#34097=DIRECTION('center_axis',(0.,-1.,0.));
#34098=DIRECTION('ref_axis',(-1.,0.,0.));
#34099=DIRECTION('',(0.,-1.,0.));
#34100=DIRECTION('center_axis',(0.,-1.,0.));
#34101=DIRECTION('ref_axis',(-1.,0.,0.));
#34102=DIRECTION('',(0.,1.,0.));
#34103=DIRECTION('center_axis',(0.,-1.,0.));
#34104=DIRECTION('ref_axis',(-0.882032681580533,0.,0.471188230565932));
#34105=DIRECTION('',(0.,-1.,0.));
#34106=DIRECTION('center_axis',(1.,0.,0.));
#34107=DIRECTION('ref_axis',(0.,1.,0.));
#34108=DIRECTION('',(0.,0.,1.));
#34109=DIRECTION('',(0.,1.,0.));
#34110=DIRECTION('',(0.,0.,1.));
#34111=DIRECTION('center_axis',(1.,0.,0.));
#34112=DIRECTION('ref_axis',(0.,0.,-1.));
#34113=DIRECTION('center_axis',(-1.,0.,0.));
#34114=DIRECTION('ref_axis',(0.,0.,1.));
#34115=DIRECTION('center_axis',(0.,-1.,-1.22464679914736E-16));
#34116=DIRECTION('ref_axis',(0.,-1.22464679914736E-16,1.));
#34117=DIRECTION('center_axis',(1.,0.,0.));
#34118=DIRECTION('ref_axis',(0.,0.,1.));
#34119=DIRECTION('center_axis',(1.,0.,0.));
#34120=DIRECTION('ref_axis',(0.,0.,1.));
#34121=DIRECTION('center_axis',(-1.,0.,0.));
#34122=DIRECTION('ref_axis',(0.,0.,1.));
#34123=DIRECTION('center_axis',(-1.,0.,0.));
#34124=DIRECTION('ref_axis',(0.,0.,1.));
#34125=DIRECTION('',(0.,1.,0.));
#34126=DIRECTION('',(0.,0.,-1.));
#34127=DIRECTION('',(0.,1.,0.));
#34128=DIRECTION('',(0.,0.,-1.));
#34129=DIRECTION('',(0.,0.,1.));
#34130=DIRECTION('',(0.,1.,0.));
#34131=DIRECTION('',(0.,0.,1.));
#34132=DIRECTION('',(0.,1.,0.));
#34133=DIRECTION('center_axis',(-1.,0.,0.));
#34134=DIRECTION('ref_axis',(0.,0.,1.));
#34135=DIRECTION('center_axis',(-1.,0.,0.));
#34136=DIRECTION('ref_axis',(0.,0.,1.));
#34137=DIRECTION('center_axis',(-1.,0.,0.));
#34138=DIRECTION('ref_axis',(0.,0.,1.));
#34139=DIRECTION('center_axis',(-1.,0.,0.));
#34140=DIRECTION('ref_axis',(0.,0.,1.));
#34141=DIRECTION('center_axis',(-1.,0.,0.));
#34142=DIRECTION('ref_axis',(0.,0.,1.));
#34143=DIRECTION('',(-1.,0.,0.));
#34144=DIRECTION('center_axis',(1.,0.,0.));
#34145=DIRECTION('ref_axis',(0.,0.,-1.));
#34146=DIRECTION('center_axis',(0.,-1.,-1.22464679914736E-16));
#34147=DIRECTION('ref_axis',(0.,-1.22464679914736E-16,1.));
#34148=DIRECTION('center_axis',(1.,0.,0.));
#34149=DIRECTION('ref_axis',(0.,0.,1.));
#34150=DIRECTION('center_axis',(1.,0.,0.));
#34151=DIRECTION('ref_axis',(0.,0.,1.));
#34152=DIRECTION('center_axis',(-1.,0.,0.));
#34153=DIRECTION('ref_axis',(0.,0.,1.));
#34154=DIRECTION('center_axis',(-1.,0.,0.));
#34155=DIRECTION('ref_axis',(0.,0.,1.));
#34156=DIRECTION('',(-1.,0.,0.));
#34157=DIRECTION('center_axis',(1.,0.,0.));
#34158=DIRECTION('ref_axis',(0.,0.,-1.));
#34159=DIRECTION('center_axis',(0.,-1.,-1.22464679914736E-16));
#34160=DIRECTION('ref_axis',(0.,-1.22464679914736E-16,1.));
#34161=DIRECTION('center_axis',(1.,0.,0.));
#34162=DIRECTION('ref_axis',(0.,0.,1.));
#34163=DIRECTION('center_axis',(1.,0.,0.));
#34164=DIRECTION('ref_axis',(0.,0.,1.));
#34165=DIRECTION('center_axis',(-1.,0.,0.));
#34166=DIRECTION('ref_axis',(0.,0.,1.));
#34167=DIRECTION('center_axis',(-1.,0.,0.));
#34168=DIRECTION('ref_axis',(0.,0.,1.));
#34169=DIRECTION('',(-1.,0.,0.));
#34170=DIRECTION('center_axis',(1.,0.,0.));
#34171=DIRECTION('ref_axis',(0.,0.,-1.));
#34172=DIRECTION('center_axis',(0.,-1.,-1.22464679914736E-16));
#34173=DIRECTION('ref_axis',(0.,-1.22464679914736E-16,1.));
#34174=DIRECTION('center_axis',(1.,0.,0.));
#34175=DIRECTION('ref_axis',(0.,0.,1.));
#34176=DIRECTION('center_axis',(1.,0.,0.));
#34177=DIRECTION('ref_axis',(0.,0.,1.));
#34178=DIRECTION('center_axis',(0.,1.,0.));
#34179=DIRECTION('ref_axis',(-2.31525300922612E-5,0.,-0.99999999973198));
#34180=DIRECTION('',(0.,1.,0.));
#34181=DIRECTION('center_axis',(0.,-0.707106781186552,-0.707106781186543));
#34182=DIRECTION('ref_axis',(4.79143098953268E-21,0.707106781186543,-0.707106781186552));
#34183=DIRECTION('',(0.,1.,0.));
#34184=DIRECTION('center_axis',(0.,0.707106781186552,-0.707106781186543));
#34185=DIRECTION('ref_axis',(4.79143098953268E-21,-0.707106781186543,-0.707106781186552));
#34186=DIRECTION('',(0.,1.,0.));
#34187=DIRECTION('center_axis',(-1.,0.,0.));
#34188=DIRECTION('ref_axis',(0.,0.,1.));
#34189=DIRECTION('center_axis',(-1.,0.,0.));
#34190=DIRECTION('ref_axis',(0.,0.,1.));
#34191=DIRECTION('',(-1.,0.,0.));
#34192=DIRECTION('center_axis',(0.,1.,0.));
#34193=DIRECTION('ref_axis',(0.224630175168819,0.,0.974444089932114));
#34194=DIRECTION('center_axis',(0.,-1.,0.));
#34195=DIRECTION('ref_axis',(0.224630175168819,0.,0.974444089932114));
#34196=DIRECTION('',(0.,1.,0.));
#34197=DIRECTION('center_axis',(0.,1.,0.));
#34198=DIRECTION('ref_axis',(0.224630175168819,0.,0.974444089932114));
#34199=DIRECTION('center_axis',(-1.,0.,0.));
#34200=DIRECTION('ref_axis',(0.,-1.,0.));
#34201=DIRECTION('',(0.,0.,1.));
#34202=DIRECTION('',(0.,-1.,0.));
#34203=DIRECTION('',(0.,0.707106781186568,-0.707106781186527));
#34204=DIRECTION('',(0.,0.,1.));
#34205=DIRECTION('',(0.,-1.,0.));
#34206=DIRECTION('',(0.,0.707106781186568,0.707106781186527));
#34207=DIRECTION('',(0.,-1.,0.));
#34208=DIRECTION('',(0.,0.,1.));
#34209=DIRECTION('center_axis',(1.,0.,0.));
#34210=DIRECTION('ref_axis',(0.,0.,1.));
#34211=DIRECTION('center_axis',(1.,0.,0.));
#34212=DIRECTION('ref_axis',(0.,0.,1.));
#34213=DIRECTION('center_axis',(1.,0.,0.));
#34214=DIRECTION('ref_axis',(0.,0.,1.));
#34215=DIRECTION('center_axis',(1.,0.,0.));
#34216=DIRECTION('ref_axis',(0.,0.,1.));
#34217=DIRECTION('center_axis',(0.,0.,1.));
#34218=DIRECTION('ref_axis',(1.,0.,0.));
#34219=DIRECTION('center_axis',(1.22464679914735E-16,-1.,0.));
#34220=DIRECTION('ref_axis',(-1.,-1.22464679914735E-16,0.));
#34221=DIRECTION('center_axis',(0.,0.,1.));
#34222=DIRECTION('ref_axis',(-1.,1.22464679914735E-16,0.));
#34223=DIRECTION('center_axis',(0.,0.,1.));
#34224=DIRECTION('ref_axis',(1.,0.,0.));
#34225=DIRECTION('',(0.,0.,1.));
#34226=DIRECTION('center_axis',(0.,0.,-1.));
#34227=DIRECTION('ref_axis',(1.,0.,0.));
#34228=DIRECTION('center_axis',(0.,0.,-1.));
#34229=DIRECTION('ref_axis',(1.,0.,0.));
#34230=DIRECTION('center_axis',(0.,-1.,0.));
#34231=DIRECTION('ref_axis',(0.,0.,-1.));
#34232=DIRECTION('center_axis',(0.,1.,0.));
#34233=DIRECTION('ref_axis',(0.769575246904488,0.,0.638556136413938));
#34234=DIRECTION('center_axis',(0.,-1.,0.));
#34235=DIRECTION('ref_axis',(0.769575246904488,0.,0.638556136413938));
#34236=DIRECTION('center_axis',(0.,1.,0.));
#34237=DIRECTION('ref_axis',(0.490062423506214,0.,0.8716873413485));
#34238=DIRECTION('',(0.,1.,0.));
#34239=DIRECTION('center_axis',(0.,1.,0.));
#34240=DIRECTION('ref_axis',(0.769575246904488,0.,0.638556136413938));
#34241=DIRECTION('',(0.,-1.,0.));
#34242=DIRECTION('center_axis',(1.,0.,0.));
#34243=DIRECTION('ref_axis',(0.,0.,-1.));
#34244=DIRECTION('',(0.,0.,-1.));
#34245=DIRECTION('',(0.,1.,0.));
#34246=DIRECTION('',(0.,0.,1.));
#34247=DIRECTION('center_axis',(0.,1.,0.));
#34248=DIRECTION('ref_axis',(0.,0.,1.));
#34249=DIRECTION('center_axis',(0.,-1.,0.));
#34250=DIRECTION('ref_axis',(0.769575246904488,0.,0.638556136413938));
#34251=DIRECTION('center_axis',(0.,1.,0.));
#34252=DIRECTION('ref_axis',(1.,0.,0.));
#34253=DIRECTION('',(0.,0.,1.));
#34254=DIRECTION('center_axis',(0.,-1.,0.));
#34255=DIRECTION('ref_axis',(-6.22021185922419E-5,0.,0.999999998065448));
#34256=DIRECTION('',(-1.,0.,0.));
#34257=DIRECTION('center_axis',(1.,0.,0.));
#34258=DIRECTION('ref_axis',(0.,0.,-1.));
#34259=DIRECTION('',(0.,0.,-1.));
#34260=DIRECTION('',(0.,1.,0.));
#34261=DIRECTION('center_axis',(0.,0.,-1.));
#34262=DIRECTION('ref_axis',(-1.,0.,0.));
#34263=DIRECTION('center_axis',(0.,0.,1.));
#34264=DIRECTION('ref_axis',(1.,0.,0.));
#34265=DIRECTION('center_axis',(-1.22464679914735E-16,-1.,0.));
#34266=DIRECTION('ref_axis',(1.,-1.22464679914735E-16,0.));
#34267=DIRECTION('center_axis',(0.,0.,1.));
#34268=DIRECTION('ref_axis',(1.,0.,0.));
#34269=DIRECTION('center_axis',(0.,0.,-1.));
#34270=DIRECTION('ref_axis',(0.,-1.,0.));
#34271=DIRECTION('center_axis',(0.,0.,-1.));
#34272=DIRECTION('ref_axis',(-0.707106781186547,-0.707106781186547,0.));
#34273=DIRECTION('',(-1.,0.,0.));
#34274=DIRECTION('center_axis',(0.,0.,-1.));
#34275=DIRECTION('ref_axis',(0.707106781186547,-0.707106781186547,0.));
#34276=DIRECTION('',(0.,-1.,0.));
#34277=DIRECTION('center_axis',(0.,0.,-1.));
#34278=DIRECTION('ref_axis',(0.707106781186547,0.707106781186547,0.));
#34279=DIRECTION('',(1.,0.,0.));
#34280=DIRECTION('center_axis',(0.,0.,-1.));
#34281=DIRECTION('ref_axis',(-0.707106781186547,0.707106781186547,0.));
#34282=DIRECTION('center_axis',(0.,0.,-1.));
#34283=DIRECTION('ref_axis',(1.,0.,0.));
#34284=DIRECTION('center_axis',(0.,0.,-1.));
#34285=DIRECTION('ref_axis',(1.,0.,0.));
#34286=DIRECTION('center_axis',(0.,0.,-1.));
#34287=DIRECTION('ref_axis',(1.,0.,0.));
#34288=DIRECTION('center_axis',(0.,0.,-1.));
#34289=DIRECTION('ref_axis',(1.,0.,0.));
#34290=DIRECTION('',(0.,-1.,0.));
#34291=DIRECTION('',(-1.,0.,0.));
#34292=DIRECTION('',(0.,-1.,0.));
#34293=DIRECTION('',(-1.,0.,0.));
#34294=DIRECTION('',(0.,1.,0.));
#34295=DIRECTION('',(1.,0.,0.));
#34296=DIRECTION('',(0.,-1.,0.));
#34297=DIRECTION('',(1.,0.,0.));
#34298=DIRECTION('',(0.,-1.,0.));
#34299=DIRECTION('',(1.,0.,0.));
#34300=DIRECTION('',(-1.,0.,0.));
#34301=DIRECTION('center_axis',(0.,1.,0.));
#34302=DIRECTION('ref_axis',(0.66778348591556,0.,-0.744355570905776));
#34303=DIRECTION('center_axis',(0.,-1.,0.));
#34304=DIRECTION('ref_axis',(0.66778348591556,0.,-0.744355570905776));
#34305=DIRECTION('center_axis',(0.,-0.707106781186552,0.707106781186543));
#34306=DIRECTION('ref_axis',(1.96261557335473E-16,-0.707106781186543,-0.707106781186552));
#34307=DIRECTION('center_axis',(0.,0.707106781186552,0.707106781186543));
#34308=DIRECTION('ref_axis',(1.96261557335473E-16,0.707106781186543,-0.707106781186552));
#34309=DIRECTION('center_axis',(-1.,0.,0.));
#34310=DIRECTION('ref_axis',(0.,0.,1.));
#34311=DIRECTION('center_axis',(0.,-1.,1.22464679914736E-16));
#34312=DIRECTION('ref_axis',(0.,-1.22464679914736E-16,-1.));
#34313=DIRECTION('center_axis',(-1.,0.,0.));
#34314=DIRECTION('ref_axis',(0.,0.,1.));
#34315=DIRECTION('center_axis',(0.,-1.,1.22464679914736E-16));
#34316=DIRECTION('ref_axis',(0.,-1.22464679914736E-16,-1.));
#34317=DIRECTION('center_axis',(-1.,0.,0.));
#34318=DIRECTION('ref_axis',(0.,0.,1.));
#34319=DIRECTION('center_axis',(0.,-1.,1.22464679914736E-16));
#34320=DIRECTION('ref_axis',(0.,-1.22464679914736E-16,-1.));
#34321=DIRECTION('center_axis',(-1.,0.,0.));
#34322=DIRECTION('ref_axis',(0.,0.,1.));
#34323=DIRECTION('center_axis',(0.,-1.,1.22464679914736E-16));
#34324=DIRECTION('ref_axis',(0.,-1.22464679914736E-16,-1.));
#34325=DIRECTION('center_axis',(0.,1.,0.));
#34326=DIRECTION('ref_axis',(0.734977615278278,0.,-0.678091369241532));
#34327=DIRECTION('center_axis',(0.,-0.707106781186552,-0.707106781186543));
#34328=DIRECTION('ref_axis',(0.,0.707106781186543,-0.707106781186552));
#34329=DIRECTION('',(0.,-1.,0.));
#34330=DIRECTION('center_axis',(0.,0.707106781186552,-0.707106781186543));
#34331=DIRECTION('ref_axis',(0.,-0.707106781186543,-0.707106781186552));
#34332=DIRECTION('',(0.,1.,0.));
#34333=DIRECTION('',(0.,1.,0.));
#34334=DIRECTION('',(0.,1.,0.));
#34335=DIRECTION('center_axis',(0.,0.,-1.));
#34336=DIRECTION('ref_axis',(0.707106781186543,0.707106781186552,0.));
#34337=DIRECTION('center_axis',(0.,0.,1.));
#34338=DIRECTION('ref_axis',(0.707106781186543,0.707106781186552,0.));
#34339=DIRECTION('',(0.,0.,-1.));
#34340=DIRECTION('center_axis',(0.,0.,-1.));
#34341=DIRECTION('ref_axis',(-1.,0.,0.));
#34342=DIRECTION('',(-0.707106781186543,0.707106781186552,0.));
#34343=DIRECTION('',(1.,0.,0.));
#34344=DIRECTION('',(0.,1.,0.));
#34345=DIRECTION('center_axis',(0.,1.,0.));
#34346=DIRECTION('ref_axis',(0.,0.,-1.));
#34347=DIRECTION('center_axis',(0.,1.,0.));
#34348=DIRECTION('ref_axis',(0.,0.,-1.));
#34349=DIRECTION('center_axis',(-0.0803841899203101,0.,0.996763955011845));
#34350=DIRECTION('ref_axis',(0.996763955011845,0.,0.0803841899203101));
#34351=DIRECTION('',(0.996763955011845,0.,0.0803841899203101));
#34352=DIRECTION('',(0.996211888614194,0.0332777802630094,0.0803396684366286));
#34353=DIRECTION('',(-0.996763955011845,0.,-0.0803841899203101));
#34354=DIRECTION('',(0.996763955011845,0.,0.0803841899203101));
#34355=DIRECTION('',(-0.996211888614194,0.0332777802630094,-0.0803396684366286));
#34356=DIRECTION('',(-0.996763955011845,0.,-0.0803841899203101));
#34357=DIRECTION('center_axis',(1.,0.,0.));
#34358=DIRECTION('ref_axis',(0.,0.,-1.));
#34359=DIRECTION('',(0.,0.,1.));
#34360=DIRECTION('center_axis',(0.,-1.,0.));
#34361=DIRECTION('ref_axis',(0.,0.,-1.));
#34362=DIRECTION('center_axis',(0.,-1.,0.));
#34363=DIRECTION('ref_axis',(-0.742667400108486,0.,0.669660460842733));
#34364=DIRECTION('center_axis',(0.,-1.,0.));
#34365=DIRECTION('ref_axis',(1.,0.,0.));
#34366=DIRECTION('',(1.,0.,0.));
#34367=DIRECTION('center_axis',(0.,1.,0.));
#34368=DIRECTION('ref_axis',(-0.99999999973198,0.,2.31525300940375E-5));
#34369=DIRECTION('center_axis',(0.,1.,0.));
#34370=DIRECTION('ref_axis',(0.,0.,1.));
#34371=DIRECTION('center_axis',(0.,1.,0.));
#34372=DIRECTION('ref_axis',(-0.742667400108486,0.,0.669660460842733));
#34373=DIRECTION('center_axis',(0.,1.,0.));
#34374=DIRECTION('ref_axis',(-1.,0.,0.));
#34375=DIRECTION('center_axis',(0.,-1.,0.));
#34376=DIRECTION('ref_axis',(-0.99999999973198,0.,2.31525300940375E-5));
#34377=DIRECTION('',(-1.,0.,0.));
#34378=DIRECTION('center_axis',(0.,0.,1.));
#34379=DIRECTION('ref_axis',(0.707106781186543,-0.707106781186552,0.));
#34380=DIRECTION('center_axis',(0.,0.,1.));
#34381=DIRECTION('ref_axis',(0.707106781186543,-0.707106781186552,0.));
#34382=DIRECTION('center_axis',(0.,0.,-1.));
#34383=DIRECTION('ref_axis',(-1.,0.,0.));
#34384=DIRECTION('',(0.,1.,0.));
#34385=DIRECTION('',(-1.,0.,0.));
#34386=DIRECTION('',(-0.707106781186552,-0.707106781186543,0.));
#34387=DIRECTION('center_axis',(-1.,0.,0.));
#34388=DIRECTION('ref_axis',(0.,0.,1.));
#34389=DIRECTION('',(0.,0.,1.));
#34390=DIRECTION('center_axis',(0.,0.,-1.));
#34391=DIRECTION('ref_axis',(-1.,0.,0.));
#34392=DIRECTION('',(-1.,0.,0.));
#34393=DIRECTION('center_axis',(0.,1.,0.));
#34394=DIRECTION('ref_axis',(-1.,0.,3.55271367880049E-15));
#34395=DIRECTION('',(0.707106781186541,-0.707106781186554,0.));
#34396=DIRECTION('center_axis',(0.,1.,0.));
#34397=DIRECTION('ref_axis',(-1.,0.,3.55271367880049E-15));
#34398=DIRECTION('center_axis',(0.,1.,0.));
#34399=DIRECTION('ref_axis',(-1.,0.,3.55271367880049E-15));
#34400=DIRECTION('center_axis',(0.,1.,0.));
#34401=DIRECTION('ref_axis',(-1.,0.,3.55271367880049E-15));
#34402=DIRECTION('',(0.,-0.707106781186552,-0.707106781186543));
#34403=DIRECTION('center_axis',(0.,1.,0.));
#34404=DIRECTION('ref_axis',(1.,0.,0.));
#34405=DIRECTION('',(0.,0.,1.));
#34406=DIRECTION('center_axis',(0.,1.,0.));
#34407=DIRECTION('ref_axis',(-2.66453525910037E-15,0.,-1.));
#34408=DIRECTION('',(-1.,0.,0.));
#34409=DIRECTION('center_axis',(0.,-1.,0.));
#34410=DIRECTION('ref_axis',(-8.88178419700126E-16,0.,1.));
#34411=DIRECTION('',(0.,0.,1.));
#34412=DIRECTION('center_axis',(0.,-1.,0.));
#34413=DIRECTION('ref_axis',(1.,0.,0.));
#34414=DIRECTION('',(-1.,0.,0.));
#34415=DIRECTION('center_axis',(0.,-1.,0.));
#34416=DIRECTION('ref_axis',(0.,0.,-1.));
#34417=DIRECTION('center_axis',(0.,1.,0.));
#34418=DIRECTION('ref_axis',(-1.,0.,0.));
#34419=DIRECTION('',(0.,0.,1.));
#34420=DIRECTION('center_axis',(0.,-1.,0.));
#34421=DIRECTION('ref_axis',(1.,0.,0.));
#34422=DIRECTION('',(1.,0.,0.));
#34423=DIRECTION('',(1.,0.,0.));
#34424=DIRECTION('',(0.,0.,-1.));
#34425=DIRECTION('',(-1.,0.,0.));
#34426=DIRECTION('',(0.,0.,1.));
#34427=DIRECTION('center_axis',(0.,-1.,0.));
#34428=DIRECTION('ref_axis',(1.,0.,0.));
#34429=DIRECTION('',(1.,0.,0.));
#34430=DIRECTION('',(0.562642780375869,0.,-0.826700128033685));
#34431=DIRECTION('',(0.,0.,1.));
#34432=DIRECTION('',(1.,0.,0.));
#34433=DIRECTION('',(0.,0.,-1.));
#34434=DIRECTION('',(-1.,0.,0.));
#34435=DIRECTION('',(-0.563462177299479,0.,0.826141861155171));
#34436=DIRECTION('',(0.,0.,-1.));
#34437=DIRECTION('',(-1.,0.,0.));
#34438=DIRECTION('',(0.,0.,1.));
#34439=DIRECTION('',(0.,0.,-1.));
#34440=DIRECTION('',(-1.,0.,0.));
#34441=DIRECTION('',(0.,0.,1.));
#34442=DIRECTION('',(0.,0.,1.));
#34443=DIRECTION('',(1.,0.,0.));
#34444=DIRECTION('center_axis',(0.,1.,0.));
#34445=DIRECTION('ref_axis',(-0.99999999973198,0.,2.31525300940375E-5));
#34446=DIRECTION('center_axis',(0.,-1.,0.));
#34447=DIRECTION('ref_axis',(-0.99999999973198,0.,2.31525300940375E-5));
#34448=DIRECTION('center_axis',(0.,1.,0.));
#34449=DIRECTION('ref_axis',(1.,0.,0.));
#34450=DIRECTION('center_axis',(0.,0.,-1.));
#34451=DIRECTION('ref_axis',(-1.,0.,0.));
#34452=DIRECTION('',(1.,0.,0.));
#34453=DIRECTION('center_axis',(-1.,0.,0.));
#34454=DIRECTION('ref_axis',(0.,0.,1.));
#34455=DIRECTION('',(0.,0.,-1.));
#34456=DIRECTION('center_axis',(0.,1.,0.));
#34457=DIRECTION('ref_axis',(-1.,0.,0.));
#34458=DIRECTION('center_axis',(0.,1.,0.));
#34459=DIRECTION('ref_axis',(-1.,0.,0.));
#34460=DIRECTION('',(0.,1.,0.));
#34461=DIRECTION('center_axis',(0.,-1.,0.));
#34462=DIRECTION('ref_axis',(-1.,0.,0.));
#34463=DIRECTION('center_axis',(0.,-1.,0.));
#34464=DIRECTION('ref_axis',(-1.,0.,0.));
#34465=DIRECTION('center_axis',(0.,-1.,0.));
#34466=DIRECTION('ref_axis',(-1.,0.,0.));
#34467=DIRECTION('',(0.707106781186543,0.707106781186552,0.));
#34468=DIRECTION('center_axis',(0.,1.,0.));
#34469=DIRECTION('ref_axis',(1.,0.,0.));
#34470=DIRECTION('',(1.,0.,0.));
#34471=DIRECTION('center_axis',(0.,1.,0.));
#34472=DIRECTION('ref_axis',(1.,0.,0.));
#34473=DIRECTION('',(0.,0.,-1.));
#34474=DIRECTION('center_axis',(0.,1.,0.));
#34475=DIRECTION('ref_axis',(-8.88178419700126E-16,0.,1.));
#34476=DIRECTION('',(1.,0.,0.));
#34477=DIRECTION('center_axis',(0.,-1.,0.));
#34478=DIRECTION('ref_axis',(-2.66453525910037E-15,0.,-1.));
#34479=DIRECTION('',(0.,0.,-1.));
#34480=DIRECTION('center_axis',(0.,-1.,0.));
#34481=DIRECTION('ref_axis',(-1.,0.,3.55271367880049E-15));
#34482=DIRECTION('center_axis',(0.,-1.,0.));
#34483=DIRECTION('ref_axis',(-1.,0.,3.55271367880049E-15));
#34484=DIRECTION('',(-1.,0.,0.));
#34485=DIRECTION('center_axis',(0.,1.,0.));
#34486=DIRECTION('ref_axis',(1.,0.,0.));
#34487=DIRECTION('',(0.,0.,-1.));
#34488=DIRECTION('center_axis',(0.,1.,0.));
#34489=DIRECTION('ref_axis',(1.,0.,0.));
#34490=DIRECTION('center_axis',(0.,-1.,0.));
#34491=DIRECTION('ref_axis',(-1.,0.,3.55271367880049E-15));
#34492=DIRECTION('',(0.707106781186545,0.70710678118655,0.));
#34493=DIRECTION('center_axis',(0.,1.,0.));
#34494=DIRECTION('ref_axis',(-0.99999999973198,0.,2.31525300940375E-5));
#34495=DIRECTION('center_axis',(0.,-1.,0.));
#34496=DIRECTION('ref_axis',(-0.99999999973198,0.,2.31525300940375E-5));
#34497=DIRECTION('center_axis',(0.,1.,0.));
#34498=DIRECTION('ref_axis',(1.,0.,0.));
#34499=DIRECTION('center_axis',(0.,1.,0.));
#34500=DIRECTION('ref_axis',(-0.99999999973198,0.,2.31525300940375E-5));
#34501=DIRECTION('',(0.,1.,0.));
#34502=DIRECTION('center_axis',(0.,0.707106781186527,0.707106781186568));
#34503=DIRECTION('ref_axis',(3.63166511851617E-17,-0.707106781186568,0.707106781186527));
#34504=DIRECTION('center_axis',(0.,1.,0.));
#34505=DIRECTION('ref_axis',(-0.99999999973198,0.,2.31525300940375E-5));
#34506=DIRECTION('center_axis',(0.,-0.707106781186527,0.707106781186568));
#34507=DIRECTION('ref_axis',(3.63166511851617E-17,0.707106781186568,0.707106781186527));
#34508=DIRECTION('',(0.,1.,0.));
#34509=DIRECTION('center_axis',(0.,1.,0.));
#34510=DIRECTION('ref_axis',(1.,0.,0.));
#34511=DIRECTION('',(-1.,0.,0.));
#34512=DIRECTION('center_axis',(0.,1.,0.));
#34513=DIRECTION('ref_axis',(0.,0.,-1.));
#34514=DIRECTION('',(-1.,0.,0.));
#34515=DIRECTION('center_axis',(0.,1.,0.));
#34516=DIRECTION('ref_axis',(0.,0.,-1.));
#34517=DIRECTION('center_axis',(0.,1.,0.));
#34518=DIRECTION('ref_axis',(1.,0.,0.));
#34519=DIRECTION('',(1.,0.,0.));
#34520=DIRECTION('center_axis',(0.,-1.,0.));
#34521=DIRECTION('ref_axis',(0.,0.,-1.));
#34522=DIRECTION('',(1.,0.,0.));
#34523=DIRECTION('center_axis',(0.,-1.,0.));
#34524=DIRECTION('ref_axis',(0.,0.,-1.));
#34525=DIRECTION('center_axis',(0.,1.,0.));
#34526=DIRECTION('ref_axis',(1.,0.,0.));
#34527=DIRECTION('center_axis',(0.,-1.,0.));
#34528=DIRECTION('ref_axis',(1.,0.,0.));
#34529=DIRECTION('center_axis',(0.,1.,0.));
#34530=DIRECTION('ref_axis',(1.,0.,0.));
#34531=DIRECTION('center_axis',(0.,1.,0.));
#34532=DIRECTION('ref_axis',(1.,0.,0.));
#34533=DIRECTION('center_axis',(0.,1.,0.));
#34534=DIRECTION('ref_axis',(1.,0.,0.));
#34535=DIRECTION('center_axis',(0.,0.707106781186543,-0.707106781186552));
#34536=DIRECTION('ref_axis',(0.,-0.707106781186552,-0.707106781186543));
#34537=DIRECTION('center_axis',(0.,1.,0.));
#34538=DIRECTION('ref_axis',(1.,0.,0.));
#34539=DIRECTION('center_axis',(0.,-1.,0.));
#34540=DIRECTION('ref_axis',(1.,0.,0.));
#34541=DIRECTION('center_axis',(0.,-0.707106781186543,-0.707106781186552));
#34542=DIRECTION('ref_axis',(0.,0.707106781186552,-0.707106781186543));
#34543=DIRECTION('center_axis',(0.,-0.707106781186552,-0.707106781186543));
#34544=DIRECTION('ref_axis',(-1.,0.,0.));
#34545=DIRECTION('',(1.,0.,0.));
#34546=DIRECTION('',(-0.57735026918962,-0.577350269189625,0.577350269189633));
#34547=DIRECTION('center_axis',(0.,-1.,0.));
#34548=DIRECTION('ref_axis',(-2.66453525910037E-15,0.,-1.));
#34549=DIRECTION('',(0.707106781186537,0.707106781186558,0.));
#34550=DIRECTION('',(0.,0.707106781186552,0.707106781186543));
#34551=DIRECTION('center_axis',(0.,-1.,0.));
#34552=DIRECTION('ref_axis',(0.,0.,-1.));
#34553=DIRECTION('center_axis',(0.,0.923879532511286,-0.382683432365092));
#34554=DIRECTION('ref_axis',(5.40315374398936E-15,-0.382683432365092,-0.923879532511286));
#34555=DIRECTION('center_axis',(0.,-1.,0.));
#34556=DIRECTION('ref_axis',(0.,0.,-1.));
#34557=DIRECTION('center_axis',(0.,0.923879532511286,0.382683432365092));
#34558=DIRECTION('ref_axis',(0.,-0.382683432365092,0.923879532511286));
#34559=DIRECTION('center_axis',(0.,-0.923879532511286,-0.382683432365092));
#34560=DIRECTION('ref_axis',(5.40315374398936E-15,-0.382683432365092,0.923879532511286));
#34561=DIRECTION('',(-1.,0.,0.));
#34562=DIRECTION('center_axis',(0.,-0.923879532511286,-0.382683432365092));
#34563=DIRECTION('ref_axis',(1.55829399144591E-15,-0.382683432365092,0.923879532511286));
#34564=DIRECTION('center_axis',(0.,1.,0.));
#34565=DIRECTION('ref_axis',(0.,0.,-1.));
#34566=DIRECTION('center_axis',(0.,-0.707106781186543,-0.707106781186552));
#34567=DIRECTION('ref_axis',(0.,0.707106781186552,-0.707106781186543));
#34568=DIRECTION('center_axis',(0.,1.,0.));
#34569=DIRECTION('ref_axis',(0.,0.,-1.));
#34570=DIRECTION('center_axis',(0.,0.,1.));
#34571=DIRECTION('ref_axis',(1.,0.,0.));
#34572=DIRECTION('',(0.,-1.,0.));
#34573=DIRECTION('',(1.,0.,0.));
#34574=DIRECTION('center_axis',(0.,0.,1.));
#34575=DIRECTION('ref_axis',(1.,0.,0.));
#34576=DIRECTION('',(-1.,0.,0.));
#34577=DIRECTION('',(0.,-1.,0.));
#34578=DIRECTION('',(1.,0.,0.));
#34579=DIRECTION('center_axis',(0.,1.,0.));
#34580=DIRECTION('ref_axis',(-6.22021185922419E-5,0.,0.999999998065448));
#34581=DIRECTION('center_axis',(0.,1.,0.));
#34582=DIRECTION('ref_axis',(-6.22021185922419E-5,0.,0.999999998065448));
#34583=DIRECTION('center_axis',(0.,1.,0.));
#34584=DIRECTION('ref_axis',(-6.22021185922419E-5,0.,0.999999998065448));
#34585=DIRECTION('center_axis',(0.,1.,0.));
#34586=DIRECTION('ref_axis',(1.,0.,0.));
#34587=DIRECTION('center_axis',(0.,0.,-1.));
#34588=DIRECTION('ref_axis',(-1.,0.,0.));
#34589=DIRECTION('',(1.,0.,0.));
#34590=DIRECTION('',(-1.,0.,0.));
#34591=DIRECTION('',(0.,-1.,0.));
#34592=DIRECTION('',(-1.,0.,0.));
#34593=DIRECTION('center_axis',(0.,-1.,0.));
#34594=DIRECTION('ref_axis',(-8.88178419700126E-16,0.,1.));
#34595=DIRECTION('',(0.707106781186552,-0.707106781186543,0.));
#34596=DIRECTION('',(0.,-0.707106781186552,0.707106781186543));
#34597=DIRECTION('center_axis',(0.,1.,0.));
#34598=DIRECTION('ref_axis',(-1.,0.,0.));
#34599=DIRECTION('center_axis',(0.,1.,0.));
#34600=DIRECTION('ref_axis',(-1.,0.,0.));
#34601=DIRECTION('',(0.,1.,0.));
#34602=DIRECTION('center_axis',(0.,-1.,0.));
#34603=DIRECTION('ref_axis',(-1.,0.,0.));
#34604=DIRECTION('center_axis',(1.,0.,0.));
#34605=DIRECTION('ref_axis',(0.,0.,-1.));
#34606=DIRECTION('',(0.,0.,-1.));
#34607=DIRECTION('',(0.,0.,1.));
#34608=DIRECTION('',(0.,-1.,0.));
#34609=DIRECTION('center_axis',(1.,0.,0.));
#34610=DIRECTION('ref_axis',(0.,0.,-1.));
#34611=DIRECTION('',(0.,0.,1.));
#34612=DIRECTION('',(0.,-1.,0.));
#34613=DIRECTION('',(0.,0.,-1.));
#34614=DIRECTION('center_axis',(0.,0.,-1.));
#34615=DIRECTION('ref_axis',(-1.,0.,0.));
#34616=DIRECTION('',(-1.,0.,0.));
#34617=DIRECTION('',(0.,1.,0.));
#34618=DIRECTION('',(1.,0.,0.));
#34619=DIRECTION('center_axis',(0.,0.,-1.));
#34620=DIRECTION('ref_axis',(-1.,0.,0.));
#34621=DIRECTION('',(-1.,0.,0.));
#34622=DIRECTION('',(0.,1.,0.));
#34623=DIRECTION('',(1.,0.,0.));
#34624=DIRECTION('',(0.,1.,0.));
#34625=DIRECTION('center_axis',(0.,0.,-1.));
#34626=DIRECTION('ref_axis',(-1.,0.,0.));
#34627=DIRECTION('',(1.,0.,0.));
#34628=DIRECTION('',(0.,1.,0.));
#34629=DIRECTION('',(-1.,0.,0.));
#34630=DIRECTION('',(0.,1.,0.));
#34631=DIRECTION('center_axis',(0.,1.,0.));
#34632=DIRECTION('ref_axis',(-0.99999999973198,0.,2.31525300940375E-5));
#34633=DIRECTION('center_axis',(0.,1.,0.));
#34634=DIRECTION('ref_axis',(-0.99999999973198,0.,2.31525300940375E-5));
#34635=DIRECTION('center_axis',(0.,1.,0.));
#34636=DIRECTION('ref_axis',(1.,0.,0.));
#34637=DIRECTION('center_axis',(0.,-1.,0.));
#34638=DIRECTION('ref_axis',(0.99999999973198,0.,-2.31525300911954E-5));
#34639=DIRECTION('center_axis',(0.,1.,0.));
#34640=DIRECTION('ref_axis',(-0.99999999973198,0.,2.31525300940375E-5));
#34641=DIRECTION('center_axis',(0.,-1.,0.));
#34642=DIRECTION('ref_axis',(-0.99999999973198,0.,2.31525300940375E-5));
#34643=DIRECTION('center_axis',(0.,1.,0.));
#34644=DIRECTION('ref_axis',(0.99999999973198,0.,-2.31525300911954E-5));
#34645=DIRECTION('',(0.,1.,0.));
#34646=DIRECTION('center_axis',(0.,1.,0.));
#34647=DIRECTION('ref_axis',(0.99999999973198,0.,-2.31525300911954E-5));
#34648=DIRECTION('',(0.,-1.,0.));
#34649=DIRECTION('center_axis',(0.,1.,0.));
#34650=DIRECTION('ref_axis',(1.,0.,0.));
#34651=DIRECTION('center_axis',(0.,-1.,0.));
#34652=DIRECTION('ref_axis',(-1.,0.,3.55271367880049E-15));
#34653=DIRECTION('',(2.09345661157837E-15,0.707106781186552,-0.707106781186543));
#34654=DIRECTION('center_axis',(0.,-0.707106781186527,0.707106781186568));
#34655=DIRECTION('ref_axis',(1.,0.,0.));
#34656=DIRECTION('',(0.577350269189634,0.577350269189639,0.577350269189605));
#34657=DIRECTION('center_axis',(1.,0.,0.));
#34658=DIRECTION('ref_axis',(0.,0.,-1.));
#34659=DIRECTION('',(0.,1.,0.));
#34660=DIRECTION('',(0.,0.,-1.));
#34661=DIRECTION('center_axis',(1.,0.,0.));
#34662=DIRECTION('ref_axis',(0.,0.,-1.));
#34663=DIRECTION('',(0.,0.,1.));
#34664=DIRECTION('',(0.,1.,0.));
#34665=DIRECTION('',(0.,0.,-1.));
#34666=DIRECTION('center_axis',(0.,1.,0.));
#34667=DIRECTION('ref_axis',(0.999999998065448,0.,6.22021185913536E-5));
#34668=DIRECTION('center_axis',(0.,0.707106781186543,-0.707106781186552));
#34669=DIRECTION('ref_axis',(-6.91941690502001E-18,0.707106781186552,0.707106781186543));
#34670=DIRECTION('center_axis',(0.,1.,0.));
#34671=DIRECTION('ref_axis',(0.999999998065448,0.,6.22021185913536E-5));
#34672=DIRECTION('center_axis',(0.,-0.707106781186543,-0.707106781186552));
#34673=DIRECTION('ref_axis',(-6.91941690502001E-18,-0.707106781186552,0.707106781186543));
#34674=DIRECTION('center_axis',(0.,1.,0.));
#34675=DIRECTION('ref_axis',(0.999999998065448,0.,6.22021185913536E-5));
#34676=DIRECTION('center_axis',(0.,1.,0.));
#34677=DIRECTION('ref_axis',(0.490062423506214,0.,0.8716873413485));
#34678=DIRECTION('',(0.,-1.,0.));
#34679=DIRECTION('center_axis',(0.,1.,0.));
#34680=DIRECTION('ref_axis',(1.,0.,0.));
#34681=DIRECTION('',(1.,0.,0.));
#34682=DIRECTION('center_axis',(0.,0.707106781186543,0.707106781186552));
#34683=DIRECTION('ref_axis',(1.,0.,0.));
#34684=DIRECTION('center_axis',(0.,1.,0.));
#34685=DIRECTION('ref_axis',(1.,0.,0.));
#34686=DIRECTION('',(0.707106781186543,0.707106781186552,0.));
#34687=DIRECTION('center_axis',(-1.,0.,0.));
#34688=DIRECTION('ref_axis',(0.,0.,1.));
#34689=DIRECTION('',(0.,0.,1.));
#34690=DIRECTION('',(0.,0.,-1.));
#34691=DIRECTION('center_axis',(1.,0.,0.));
#34692=DIRECTION('ref_axis',(0.,1.22464679914735E-16,1.));
#34693=DIRECTION('',(0.,-1.,0.));
#34694=DIRECTION('',(0.,1.22464679914735E-16,1.));
#34695=DIRECTION('',(0.,-1.,0.));
#34696=DIRECTION('center_axis',(0.,0.,-1.));
#34697=DIRECTION('ref_axis',(1.,5.65920170377317E-32,0.));
#34698=DIRECTION('',(1.,5.65920170377317E-32,0.));
#34699=DIRECTION('',(0.,-1.,0.));
#34700=DIRECTION('center_axis',(-1.,0.,0.));
#34701=DIRECTION('ref_axis',(0.,-1.22464679914735E-16,-1.));
#34702=DIRECTION('',(0.,-1.22464679914735E-16,-1.));
#34703=DIRECTION('',(0.,-1.,0.));
#34704=DIRECTION('',(0.,-1.,0.));
#34705=DIRECTION('',(0.,-1.,0.));
#34706=DIRECTION('center_axis',(-1.,0.,0.));
#34707=DIRECTION('ref_axis',(0.,-1.22464679914737E-16,-1.));
#34708=DIRECTION('',(0.,-1.22464679914737E-16,-1.));
#34709=DIRECTION('',(0.,-1.,0.));
#34710=DIRECTION('',(0.,-1.,0.));
#34711=DIRECTION('',(0.,-1.,0.));
#34712=DIRECTION('center_axis',(0.,0.,1.));
#34713=DIRECTION('ref_axis',(-1.,0.,0.));
#34714=DIRECTION('',(-1.,0.,0.));
#34715=DIRECTION('center_axis',(-5.65920170377317E-32,1.,-1.22464679914735E-16));
#34716=DIRECTION('ref_axis',(1.,5.65920170377317E-32,0.));
#34717=DIRECTION('center_axis',(0.,0.,1.));
#34718=DIRECTION('ref_axis',(-1.,0.,0.));
#34719=DIRECTION('',(0.,-1.,0.));
#34720=DIRECTION('',(-1.,0.,0.));
#34721=DIRECTION('',(0.,-1.,0.));
#34722=DIRECTION('center_axis',(0.826700128033685,0.,0.562642780375869));
#34723=DIRECTION('ref_axis',(-0.562642780375869,1.01241566565116E-16,0.826700128033685));
#34724=DIRECTION('',(-0.562642780375869,1.01241566565116E-16,0.826700128033685));
#34725=DIRECTION('',(0.,-1.,0.));
#34726=DIRECTION('center_axis',(-1.,0.,0.));
#34727=DIRECTION('ref_axis',(0.,-1.22464679914735E-16,-1.));
#34728=DIRECTION('',(0.,-1.22464679914735E-16,-1.));
#34729=DIRECTION('',(0.,-1.,0.));
#34730=DIRECTION('center_axis',(0.,0.,1.));
#34731=DIRECTION('ref_axis',(-1.,-2.73020257228944E-32,0.));
#34732=DIRECTION('',(-1.,-2.73020257228944E-32,0.));
#34733=DIRECTION('',(0.,-1.,0.));
#34734=DIRECTION('center_axis',(1.,0.,0.));
#34735=DIRECTION('ref_axis',(0.,1.22464679914735E-16,1.));
#34736=DIRECTION('',(0.,1.22464679914735E-16,1.));
#34737=DIRECTION('',(0.,-1.,0.));
#34738=DIRECTION('center_axis',(0.,0.,-1.));
#34739=DIRECTION('ref_axis',(1.,0.,0.));
#34740=DIRECTION('',(1.,0.,0.));
#34741=DIRECTION('',(0.,-1.,0.));
#34742=DIRECTION('center_axis',(-0.826141861155171,0.,-0.563462177299479));
#34743=DIRECTION('ref_axis',(0.563462177299479,-1.01173198590532E-16,-0.826141861155171));
#34744=DIRECTION('',(0.563462177299479,-1.01173198590532E-16,-0.826141861155171));
#34745=DIRECTION('',(0.,-1.,0.));
#34746=DIRECTION('center_axis',(1.,0.,0.));
#34747=DIRECTION('ref_axis',(0.,1.22464679914735E-16,1.));
#34748=DIRECTION('',(0.,1.22464679914735E-16,1.));
#34749=DIRECTION('',(0.,-1.,0.));
#34750=DIRECTION('center_axis',(0.,0.,-1.));
#34751=DIRECTION('ref_axis',(1.,0.,0.));
#34752=DIRECTION('',(1.,0.,0.));
#34753=DIRECTION('',(0.,-1.,0.));
#34754=DIRECTION('center_axis',(-1.,0.,0.));
#34755=DIRECTION('ref_axis',(0.,-1.22464679914735E-16,-1.));
#34756=DIRECTION('',(0.,-1.22464679914735E-16,-1.));
#34757=DIRECTION('center_axis',(0.,-1.,0.));
#34758=DIRECTION('ref_axis',(0.,0.,-1.));
#34759=DIRECTION('',(0.,-1.,0.));
#34760=DIRECTION('',(0.,-1.,0.));
#34761=DIRECTION('',(0.,-1.,0.));
#34762=DIRECTION('',(0.,-1.,0.));
#34763=DIRECTION('',(0.,-1.,0.));
#34764=DIRECTION('',(0.,-1.,0.));
#34765=DIRECTION('',(0.,-1.,0.));
#34766=DIRECTION('',(0.,-1.,0.));
#34767=DIRECTION('',(0.,-1.,0.));
#34768=DIRECTION('',(0.,-1.,0.));
#34769=DIRECTION('',(0.,-1.,0.));
#34770=DIRECTION('',(0.,-1.,0.));
#34771=DIRECTION('',(0.,-1.,0.));
#34772=DIRECTION('',(0.,-1.,0.));
#34773=DIRECTION('',(0.,-1.,0.));
#34774=DIRECTION('',(0.,-1.,0.));
#34775=DIRECTION('',(0.,-1.,0.));
#34776=DIRECTION('',(0.,-1.,0.));
#34777=DIRECTION('center_axis',(5.78607751208046E-16,1.,-3.04931545996342E-16));
#34778=DIRECTION('ref_axis',(1.,-5.78607751208046E-16,0.));
#34779=DIRECTION('center_axis',(0.,0.,1.));
#34780=DIRECTION('ref_axis',(-1.,0.,0.));
#34781=DIRECTION('',(0.,-1.,0.));
#34782=DIRECTION('',(-1.,0.,0.));
#34783=DIRECTION('',(0.,-1.,0.));
#34784=DIRECTION('center_axis',(1.,0.,0.));
#34785=DIRECTION('ref_axis',(0.,1.22464679914735E-16,1.));
#34786=DIRECTION('',(0.,1.22464679914735E-16,1.));
#34787=DIRECTION('',(0.,-1.,0.));
#34788=DIRECTION('center_axis',(0.,0.,-1.));
#34789=DIRECTION('ref_axis',(1.,0.,0.));
#34790=DIRECTION('',(1.,0.,0.));
#34791=DIRECTION('',(0.,-1.,0.));
#34792=DIRECTION('center_axis',(-1.,0.,0.));
#34793=DIRECTION('ref_axis',(0.,-1.22464679914735E-16,-1.));
#34794=DIRECTION('',(0.,-1.22464679914735E-16,-1.));
#34795=DIRECTION('center_axis',(0.,-1.,0.));
#34796=DIRECTION('ref_axis',(0.,0.,-1.));
#34797=DIRECTION('center_axis',(0.,0.,-1.));
#34798=DIRECTION('ref_axis',(-1.,0.,0.));
#34799=DIRECTION('center_axis',(0.,0.,1.));
#34800=DIRECTION('ref_axis',(1.,0.,0.));
#34801=DIRECTION('center_axis',(0.,0.,1.));
#34802=DIRECTION('ref_axis',(1.,0.,0.));
#34803=DIRECTION('',(0.,0.,1.));
#34804=DIRECTION('center_axis',(0.,0.,-1.));
#34805=DIRECTION('ref_axis',(-1.,0.,0.));
#34806=DIRECTION('center_axis',(0.,0.,1.));
#34807=DIRECTION('ref_axis',(1.,0.,0.));
#34808=DIRECTION('center_axis',(0.,0.,1.));
#34809=DIRECTION('ref_axis',(1.,0.,0.));
#34810=DIRECTION('',(0.,0.,1.));
#34811=DIRECTION('center_axis',(0.,0.,1.));
#34812=DIRECTION('ref_axis',(1.,0.,0.));
#34813=DIRECTION('',(0.,0.,1.));
#34814=DIRECTION('center_axis',(0.,0.,1.));
#34815=DIRECTION('ref_axis',(1.,0.,0.));
#34816=DIRECTION('',(0.,0.,1.));
#34817=DIRECTION('center_axis',(-1.,0.,0.));
#34818=DIRECTION('ref_axis',(0.,-1.,0.));
#34819=DIRECTION('',(0.,0.,1.));
#34820=DIRECTION('center_axis',(1.,0.,0.));
#34821=DIRECTION('ref_axis',(0.,1.,0.));
#34822=DIRECTION('',(0.,0.,1.));
#34823=DIRECTION('center_axis',(0.,-1.,0.));
#34824=DIRECTION('ref_axis',(1.,0.,0.));
#34825=DIRECTION('center_axis',(0.,0.,-1.));
#34826=DIRECTION('ref_axis',(0.,-1.,0.));
#34827=DIRECTION('center_axis',(-0.707106781186546,0.,-0.707106781186549));
#34828=DIRECTION('ref_axis',(-0.707106781186549,0.,0.707106781186546));
#34829=DIRECTION('',(0.,1.,0.));
#34830=DIRECTION('',(-0.707106781186546,0.,0.707106781186549));
#34831=DIRECTION('center_axis',(-1.,0.,0.));
#34832=DIRECTION('ref_axis',(0.,-1.,0.));
#34833=DIRECTION('',(0.,0.,1.));
#34834=DIRECTION('center_axis',(-0.707106781186555,0.,-0.70710678118654));
#34835=DIRECTION('ref_axis',(-0.70710678118654,0.,0.707106781186555));
#34836=DIRECTION('',(-0.57735026918962,0.577350269189625,0.577350269189633));
#34837=DIRECTION('center_axis',(0.,0.707106781186552,-0.707106781186543));
#34838=DIRECTION('ref_axis',(-1.,0.,0.));
#34839=DIRECTION('',(-1.,0.,0.));
#34840=DIRECTION('center_axis',(0.,-1.,0.));
#34841=DIRECTION('ref_axis',(1.,0.,0.));
#34842=DIRECTION('',(-1.,0.,0.));
#34843=DIRECTION('',(0.,0.,1.));
#34844=DIRECTION('center_axis',(-0.70710678118653,0.,0.707106781186565));
#34845=DIRECTION('ref_axis',(0.707106781186565,0.,0.70710678118653));
#34846=DIRECTION('',(0.,-1.,0.));
#34847=DIRECTION('',(0.577350269189635,-0.577350269189638,0.577350269189604));
#34848=DIRECTION('center_axis',(0.,0.707106781186527,0.707106781186568));
#34849=DIRECTION('ref_axis',(1.,0.,0.));
#34850=DIRECTION('center_axis',(1.,0.,0.));
#34851=DIRECTION('ref_axis',(0.,1.,0.));
#34852=DIRECTION('center_axis',(0.,1.,0.));
#34853=DIRECTION('ref_axis',(1.,0.,0.));
#34854=DIRECTION('center_axis',(0.,1.,0.));
#34855=DIRECTION('ref_axis',(1.,0.,0.));
#34856=DIRECTION('',(0.707106781186548,-0.707106781186548,-8.65956056235493E-17));
#34857=DIRECTION('center_axis',(0.,1.,0.));
#34858=DIRECTION('ref_axis',(1.,0.,0.));
#34859=DIRECTION('center_axis',(0.,-1.,0.));
#34860=DIRECTION('ref_axis',(1.,0.,0.));
#34861=DIRECTION('center_axis',(0.,-1.,0.));
#34862=DIRECTION('ref_axis',(1.,0.,0.));
#34863=DIRECTION('center_axis',(0.,-1.,0.));
#34864=DIRECTION('ref_axis',(1.,0.,0.));
#34865=DIRECTION('',(0.707106781186548,0.707106781186548,8.65956056235493E-17));
#34866=DIRECTION('center_axis',(0.,1.,0.));
#34867=DIRECTION('ref_axis',(1.,0.,0.));
#34868=DIRECTION('center_axis',(0.,1.,0.));
#34869=DIRECTION('ref_axis',(1.,0.,0.));
#34870=DIRECTION('center_axis',(0.,1.,0.));
#34871=DIRECTION('ref_axis',(1.,0.,0.));
#34872=DIRECTION('',(0.707106781186548,-0.707106781186548,-8.65956056235493E-17));
#34873=DIRECTION('center_axis',(0.,1.,0.));
#34874=DIRECTION('ref_axis',(1.,0.,0.));
#34875=DIRECTION('center_axis',(0.,1.,0.));
#34876=DIRECTION('ref_axis',(1.,0.,0.));
#34877=DIRECTION('',(0.,-1.,0.));
#34878=DIRECTION('center_axis',(0.,-1.,0.));
#34879=DIRECTION('ref_axis',(1.,0.,0.));
#34880=DIRECTION('center_axis',(0.,1.,0.));
#34881=DIRECTION('ref_axis',(1.,0.,0.));
#34882=DIRECTION('center_axis',(0.,1.,0.));
#34883=DIRECTION('ref_axis',(1.,0.,0.));
#34884=DIRECTION('',(-0.707106781186548,0.707106781186548,-8.65956056235493E-17));
#34885=DIRECTION('center_axis',(0.,-1.,0.));
#34886=DIRECTION('ref_axis',(1.,0.,0.));
#34887=DIRECTION('',(0.707106781186548,0.707106781186548,8.65956056235493E-17));
#34888=DIRECTION('center_axis',(0.,-1.,0.));
#34889=DIRECTION('ref_axis',(1.,0.,0.));
#34890=DIRECTION('center_axis',(0.,1.,0.));
#34891=DIRECTION('ref_axis',(1.,0.,0.));
#34892=DIRECTION('center_axis',(0.,1.,0.));
#34893=DIRECTION('ref_axis',(1.,0.,0.));
#34894=DIRECTION('',(0.,-1.,0.));
#34895=DIRECTION('center_axis',(0.,-1.,0.));
#34896=DIRECTION('ref_axis',(1.,0.,0.));
#34897=DIRECTION('',(-0.707106781186548,-0.707106781186548,8.65956056235493E-17));
#34898=DIRECTION('center_axis',(0.,-0.923879532511286,0.382683432365092));
#34899=DIRECTION('ref_axis',(0.,-0.382683432365092,-0.923879532511286));
#34900=DIRECTION('center_axis',(0.,0.923879532511286,-0.382683432365092));
#34901=DIRECTION('ref_axis',(1.24663519315673E-14,0.382683432365092,0.923879532511286));
#34902=DIRECTION('',(1.,0.,0.));
#34903=DIRECTION('center_axis',(0.,1.,0.));
#34904=DIRECTION('ref_axis',(-1.,0.,0.));
#34905=DIRECTION('',(0.707106781186543,-0.707106781186552,0.));
#34906=DIRECTION('center_axis',(-0.707106781186552,-0.707106781186543,0.));
#34907=DIRECTION('ref_axis',(0.,0.,1.));
#34908=DIRECTION('',(0.707106781186543,-0.707106781186552,0.));
#34909=DIRECTION('center_axis',(0.,-1.,0.));
#34910=DIRECTION('ref_axis',(1.,0.,0.));
#34911=DIRECTION('',(0.,-0.707106781186552,-0.707106781186543));
#34912=DIRECTION('center_axis',(0.,1.,0.));
#34913=DIRECTION('ref_axis',(1.,0.,0.));
#34914=DIRECTION('center_axis',(0.,-0.707106781186543,0.707106781186552));
#34915=DIRECTION('ref_axis',(1.,0.,0.));
#34916=DIRECTION('center_axis',(-0.70710678118655,-0.707106781186545,0.));
#34917=DIRECTION('ref_axis',(0.,0.,1.));
#34918=DIRECTION('',(0.707106781186545,-0.70710678118655,0.));
#34919=DIRECTION('center_axis',(0.,1.,0.));
#34920=DIRECTION('ref_axis',(-2.66453525910037E-15,0.,-1.));
#34921=DIRECTION('',(2.09345661157837E-15,-0.707106781186552,0.707106781186543));
#34922=DIRECTION('center_axis',(0.,-0.707106781186543,-0.707106781186552));
#34923=DIRECTION('ref_axis',(-1.,0.,0.));
#34924=DIRECTION('center_axis',(-0.707106781186552,-0.707106781186543,0.));
#34925=DIRECTION('ref_axis',(0.,0.,1.));
#34926=DIRECTION('',(0.707106781186543,-0.707106781186552,0.));
#34927=DIRECTION('center_axis',(0.,-1.,0.));
#34928=DIRECTION('ref_axis',(1.,0.,0.));
#34929=DIRECTION('center_axis',(0.,1.,0.));
#34930=DIRECTION('ref_axis',(1.,0.,0.));
#34931=DIRECTION('center_axis',(0.,-1.,0.));
#34932=DIRECTION('ref_axis',(1.,0.,0.));
#34933=DIRECTION('center_axis',(0.,1.,0.));
#34934=DIRECTION('ref_axis',(0.,0.,-1.));
#34935=DIRECTION('center_axis',(0.,0.707106781186543,-0.707106781186552));
#34936=DIRECTION('ref_axis',(0.,-0.707106781186552,-0.707106781186543));
#34937=DIRECTION('center_axis',(-0.707106781186552,0.707106781186543,0.));
#34938=DIRECTION('ref_axis',(0.,0.,1.));
#34939=DIRECTION('',(0.707106781186543,0.707106781186552,0.));
#34940=DIRECTION('center_axis',(0.,1.,0.));
#34941=DIRECTION('ref_axis',(-8.88178419700126E-16,0.,1.));
#34942=DIRECTION('',(0.,0.707106781186552,0.707106781186543));
#34943=DIRECTION('center_axis',(0.,0.707106781186543,-0.707106781186552));
#34944=DIRECTION('ref_axis',(-1.,0.,0.));
#34945=DIRECTION('center_axis',(-0.70710678118655,0.707106781186545,0.));
#34946=DIRECTION('ref_axis',(0.,0.,1.));
#34947=DIRECTION('center_axis',(0.,0.707106781186543,0.707106781186552));
#34948=DIRECTION('ref_axis',(1.,0.,0.));
#34949=DIRECTION('',(0.,0.707106781186552,-0.707106781186543));
#34950=DIRECTION('center_axis',(0.,1.,0.));
#34951=DIRECTION('ref_axis',(1.,0.,0.));
#34952=DIRECTION('',(0.707106781186543,0.707106781186552,0.));
#34953=DIRECTION('center_axis',(-0.707106781186552,0.707106781186543,0.));
#34954=DIRECTION('ref_axis',(0.,0.,1.));
#34955=DIRECTION('center_axis',(0.707106781186543,0.,-0.707106781186553));
#34956=DIRECTION('ref_axis',(-0.707106781186553,0.,-0.707106781186543));
#34957=DIRECTION('',(0.707106781186553,0.,0.707106781186543));
#34958=DIRECTION('',(0.,-1.,0.));
#34959=DIRECTION('',(-0.707106781186553,0.,-0.707106781186543));
#34960=DIRECTION('center_axis',(0.,0.,1.));
#34961=DIRECTION('ref_axis',(0.707106781186548,0.707106781186548,0.));
#34962=DIRECTION('',(0.,0.707106781186553,0.707106781186543));
#34963=DIRECTION('center_axis',(0.,0.,-1.));
#34964=DIRECTION('ref_axis',(0.707106781186547,0.707106781186547,0.));
#34965=DIRECTION('center_axis',(0.,0.707106781186549,-0.707106781186546));
#34966=DIRECTION('ref_axis',(-1.,0.,0.));
#34967=DIRECTION('',(0.,0.707106781186546,0.707106781186549));
#34968=DIRECTION('',(1.,0.,0.));
#34969=DIRECTION('center_axis',(0.,0.,1.));
#34970=DIRECTION('ref_axis',(-0.707106781186548,0.707106781186548,0.));
#34971=DIRECTION('center_axis',(0.,0.,-1.));
#34972=DIRECTION('ref_axis',(-0.707106781186547,0.707106781186547,0.));
#34973=DIRECTION('center_axis',(0.,0.,1.));
#34974=DIRECTION('ref_axis',(-0.707106781186548,-0.707106781186548,0.));
#34975=DIRECTION('',(0.,-0.707106781186553,0.707106781186543));
#34976=DIRECTION('center_axis',(0.,0.,-1.));
#34977=DIRECTION('ref_axis',(-0.707106781186547,-0.707106781186547,0.));
#34978=DIRECTION('center_axis',(0.,-0.707106781186549,-0.707106781186546));
#34979=DIRECTION('ref_axis',(-1.,0.,0.));
#34980=DIRECTION('',(0.,-0.707106781186546,0.707106781186549));
#34981=DIRECTION('',(-1.,0.,0.));
#34982=DIRECTION('center_axis',(0.,0.,1.));
#34983=DIRECTION('ref_axis',(0.707106781186548,-0.707106781186548,0.));
#34984=DIRECTION('center_axis',(0.,0.,-1.));
#34985=DIRECTION('ref_axis',(0.707106781186547,-0.707106781186547,0.));
#34986=DIRECTION('center_axis',(0.,0.,1.));
#34987=DIRECTION('ref_axis',(-0.707106781186547,-0.707106781186547,0.));
#34988=DIRECTION('',(0.,0.,1.));
#34989=DIRECTION('center_axis',(0.,0.,1.));
#34990=DIRECTION('ref_axis',(-0.707106781186547,-0.707106781186547,0.));
#34991=DIRECTION('center_axis',(0.,-1.,0.));
#34992=DIRECTION('ref_axis',(1.,0.,0.));
#34993=DIRECTION('',(0.,0.,-1.));
#34994=DIRECTION('',(1.,0.,0.));
#34995=DIRECTION('center_axis',(0.,0.,1.));
#34996=DIRECTION('ref_axis',(0.707106781186547,-0.707106781186547,0.));
#34997=DIRECTION('',(0.,0.,1.));
#34998=DIRECTION('center_axis',(0.,0.,1.));
#34999=DIRECTION('ref_axis',(0.707106781186547,-0.707106781186547,0.));
#35000=DIRECTION('center_axis',(1.,0.,0.));
#35001=DIRECTION('ref_axis',(0.,1.,0.));
#35002=DIRECTION('',(0.,0.,-1.));
#35003=DIRECTION('',(0.,1.,0.));
#35004=DIRECTION('center_axis',(0.,-0.707106781186543,0.707106781186552));
#35005=DIRECTION('ref_axis',(1.,0.,0.));
#35006=DIRECTION('center_axis',(0.,0.,-1.));
#35007=DIRECTION('ref_axis',(-0.707106781186547,-0.707106781186547,0.));
#35008=DIRECTION('',(0.,0.707106781186543,0.707106781186552));
#35009=DIRECTION('center_axis',(0.,0.,-1.));
#35010=DIRECTION('ref_axis',(-0.707106781186547,0.707106781186547,0.));
#35011=DIRECTION('',(0.,0.707106781186543,-0.707106781186552));
#35012=DIRECTION('center_axis',(0.,0.,1.));
#35013=DIRECTION('ref_axis',(-0.707106781186547,0.707106781186547,0.));
#35014=DIRECTION('center_axis',(0.,0.707106781186548,0.707106781186548));
#35015=DIRECTION('ref_axis',(1.,0.,0.));
#35016=DIRECTION('',(0.,0.707106781186548,-0.707106781186548));
#35017=DIRECTION('',(-1.,0.,0.));
#35018=DIRECTION('center_axis',(0.,0.,-1.));
#35019=DIRECTION('ref_axis',(0.707106781186548,0.707106781186548,0.));
#35020=DIRECTION('',(0.70710678118656,0.,-0.707106781186535));
#35021=DIRECTION('center_axis',(0.,0.,1.));
#35022=DIRECTION('ref_axis',(0.707106781186547,0.707106781186547,0.));
#35023=DIRECTION('center_axis',(0.707106781186552,0.,0.707106781186543));
#35024=DIRECTION('ref_axis',(0.707106781186543,0.,-0.707106781186552));
#35025=DIRECTION('',(0.707106781186543,0.,-0.707106781186552));
#35026=DIRECTION('center_axis',(0.,0.,-1.));
#35027=DIRECTION('ref_axis',(0.707106781186548,-0.707106781186548,0.));
#35028=DIRECTION('',(0.,-0.707106781186552,-0.707106781186543));
#35029=DIRECTION('center_axis',(0.,-0.707106781186548,0.707106781186548));
#35030=DIRECTION('ref_axis',(1.,0.,0.));
#35031=DIRECTION('center_axis',(0.,0.,1.));
#35032=DIRECTION('ref_axis',(0.707106781186547,0.707106781186547,0.));
#35033=DIRECTION('',(0.,0.,1.));
#35034=DIRECTION('center_axis',(0.,0.,1.));
#35035=DIRECTION('ref_axis',(-0.707106781186547,0.707106781186547,0.));
#35036=DIRECTION('',(0.,0.,-1.));
#35037=DIRECTION('center_axis',(0.,1.,0.));
#35038=DIRECTION('ref_axis',(-1.,0.,0.));
#63930=CARTESIAN_POINT('',(0.,0.,0.));
#63931=CARTESIAN_POINT('Origin',(9.31,4.82,78.));
#63932=CARTESIAN_POINT('',(5.02549199084668,4.82,73.4428061134618));
#63933=CARTESIAN_POINT('',(3.055,4.82,78.));
#63934=CARTESIAN_POINT('Origin',(9.31,4.82,78.));
#63935=CARTESIAN_POINT('',(5.02549199084668,4.82,82.5571938865382));
#63936=CARTESIAN_POINT('Origin',(9.31,4.82,78.));
#63937=CARTESIAN_POINT('',(4.60618911786999,4.52,82.565324543245));
#63938=CARTESIAN_POINT('Ctrl Pts',(5.02549199084668,4.82,82.5571938865382));
#63939=CARTESIAN_POINT('Ctrl Pts',(5.02530843195014,4.81974208420639,82.5570213111372));
#63940=CARTESIAN_POINT('Ctrl Pts',(5.02512465556946,4.81948416828985,82.556848966888));
#63941=CARTESIAN_POINT('Ctrl Pts',(4.98582218891929,4.76439138566817,82.5200843217974));
#63942=CARTESIAN_POINT('Ctrl Pts',(4.93753334401095,4.71048862403654,82.4945375858532));
#63943=CARTESIAN_POINT('Ctrl Pts',(4.84464785310685,4.6276739222328,82.4739443292949));
#63944=CARTESIAN_POINT('Ctrl Pts',(4.80287073114975,4.59679810761626,82.4733979122501));
#63945=CARTESIAN_POINT('Ctrl Pts',(4.73196607374269,4.55526307036662,82.4873225644575));
#63946=CARTESIAN_POINT('Ctrl Pts',(4.70113087228767,4.54073321204008,82.4982082535911));
#63947=CARTESIAN_POINT('Ctrl Pts',(4.64789443637829,4.52392737915209,82.5285504834486));
#63948=CARTESIAN_POINT('Ctrl Pts',(4.62586036645017,4.52,82.5453381759243));
#63949=CARTESIAN_POINT('Ctrl Pts',(4.60618911787,4.52,82.565324543245));
#63950=CARTESIAN_POINT('',(4.60618911786999,4.52,73.434675456755));
#63951=CARTESIAN_POINT('Origin',(9.31,4.52,78.));
#63952=CARTESIAN_POINT('Ctrl Pts',(4.60618911787001,4.52,73.434675456755));
#63953=CARTESIAN_POINT('Ctrl Pts',(4.62582177000828,4.52,73.4546226093476));
#63954=CARTESIAN_POINT('Ctrl Pts',(4.64779152745104,4.52391160862118,73.4713675032503));
#63955=CARTESIAN_POINT('Ctrl Pts',(4.69786840426422,4.53968449182505,73.4999585882815));
#63956=CARTESIAN_POINT('Ctrl Pts',(4.72544220605375,4.55223271719695,73.5103111906513));
#63957=CARTESIAN_POINT('Ctrl Pts',(4.78901185813479,4.58789763273166,73.5249530214543));
#63958=CARTESIAN_POINT('Ctrl Pts',(4.82447324095024,4.61297821285604,73.5260203885605));
#63959=CARTESIAN_POINT('Ctrl Pts',(4.88969454090697,4.66653559525648,73.5178493906711));
#63960=CARTESIAN_POINT('Ctrl Pts',(4.92001482640919,4.69535645684422,73.5086915524274));
#63961=CARTESIAN_POINT('Ctrl Pts',(4.97624170572235,4.75557099156908,73.4823061485807));
#63962=CARTESIAN_POINT('Ctrl Pts',(5.002315693931,4.78751138710799,73.4644871845292));
#63963=CARTESIAN_POINT('Ctrl Pts',(5.0251246555687,4.8194841682894,73.4431510331127));
#63964=CARTESIAN_POINT('Ctrl Pts',(5.02530843195051,4.81974208420691,73.4429786888625));
#63965=CARTESIAN_POINT('Ctrl Pts',(5.02549199084668,4.82,73.4428061134618));
#63966=CARTESIAN_POINT('Origin',(4.82,0.,82.7757643367319));
#63967=CARTESIAN_POINT('',(4.52,-4.52,82.7757643367319));
#63968=CARTESIAN_POINT('',(4.52,4.52,82.7757643367319));
#63969=CARTESIAN_POINT('',(4.52,0.,82.7757643367319));
#63970=CARTESIAN_POINT('Origin',(4.82,4.52,82.7757643367319));
#63971=CARTESIAN_POINT('',(5.02549199084668,-4.82,82.5571938865382));
#63972=CARTESIAN_POINT('',(5.02549199084668,0.,82.5571938865382));
#63973=CARTESIAN_POINT('',(4.60618911786999,-4.52,82.565324543245));
#63974=CARTESIAN_POINT('Ctrl Pts',(5.02549199084668,-4.82,82.5571938865382));
#63975=CARTESIAN_POINT('Ctrl Pts',(5.02530843195014,-4.81974208420639,82.5570213111372));
#63976=CARTESIAN_POINT('Ctrl Pts',(5.02512465556946,-4.81948416828985,82.556848966888));
#63977=CARTESIAN_POINT('Ctrl Pts',(4.98582218891934,-4.76439138566824,82.5200843217975));
#63978=CARTESIAN_POINT('Ctrl Pts',(4.93753334401101,-4.7104886240366,82.4945375858533));
#63979=CARTESIAN_POINT('Ctrl Pts',(4.8446478531067,-4.62767392223266,82.4739443292949));
#63980=CARTESIAN_POINT('Ctrl Pts',(4.80287073114959,-4.59679810761617,82.4733979122501));
#63981=CARTESIAN_POINT('Ctrl Pts',(4.73196607374269,-4.55526307036662,82.4873225644575));
#63982=CARTESIAN_POINT('Ctrl Pts',(4.70113087228767,-4.54073321204007,82.4982082535911));
#63983=CARTESIAN_POINT('Ctrl Pts',(4.64789443637828,-4.52392737915208,82.5285504834486));
#63984=CARTESIAN_POINT('Ctrl Pts',(4.62586036645016,-4.52,82.5453381759243));
#63985=CARTESIAN_POINT('Ctrl Pts',(4.60618911786998,-4.52,82.565324543245));
#63986=CARTESIAN_POINT('Origin',(4.82,-4.52,82.7757643367319));
#63987=CARTESIAN_POINT('Origin',(4.82,0.,73.2242356632681));
#63988=CARTESIAN_POINT('',(5.02549199084668,-4.82,73.4428061134618));
#63989=CARTESIAN_POINT('',(5.02549199084668,0.,73.4428061134618));
#63990=CARTESIAN_POINT('',(4.52,4.52,73.2242356632681));
#63991=CARTESIAN_POINT('Origin',(4.82,4.52,73.2242356632681));
#63992=CARTESIAN_POINT('',(4.52,-4.52,73.2242356632681));
#63993=CARTESIAN_POINT('',(4.52,0.,73.2242356632681));
#63994=CARTESIAN_POINT('',(4.60618911786999,-4.52,73.434675456755));
#63995=CARTESIAN_POINT('Origin',(4.82,-4.52,73.2242356632681));
#63996=CARTESIAN_POINT('Ctrl Pts',(4.60618911787,-4.52,73.434675456755));
#63997=CARTESIAN_POINT('Ctrl Pts',(4.62582177000827,-4.52,73.4546226093476));
#63998=CARTESIAN_POINT('Ctrl Pts',(4.64779152745104,-4.52391160862118,73.4713675032503));
#63999=CARTESIAN_POINT('Ctrl Pts',(4.69786840426422,-4.53968449182505,73.4999585882815));
#64000=CARTESIAN_POINT('Ctrl Pts',(4.72544220605375,-4.55223271719695,73.5103111906513));
#64001=CARTESIAN_POINT('Ctrl Pts',(4.78901185813476,-4.58789763273165,73.5249530214543));
#64002=CARTESIAN_POINT('Ctrl Pts',(4.82447324095018,-4.612978212856,73.5260203885605));
#64003=CARTESIAN_POINT('Ctrl Pts',(4.88969454090694,-4.66653559525646,73.5178493906711));
#64004=CARTESIAN_POINT('Ctrl Pts',(4.92001482640915,-4.69535645684417,73.5086915524274));
#64005=CARTESIAN_POINT('Ctrl Pts',(4.9762417057226,-4.75557099156931,73.4823061485806));
#64006=CARTESIAN_POINT('Ctrl Pts',(5.00231569392393,-4.78751138711695,73.4644871845359));
#64007=CARTESIAN_POINT('Ctrl Pts',(5.02512465556945,-4.81948416828983,73.443151033112));
#64008=CARTESIAN_POINT('Ctrl Pts',(5.02530843194999,-4.81974208420617,73.442978688863));
#64009=CARTESIAN_POINT('Ctrl Pts',(5.02549199084668,-4.82,73.4428061134618));
#64010=CARTESIAN_POINT('Origin',(9.31,-4.82,78.));
#64011=CARTESIAN_POINT('',(3.055,-4.82,78.));
#64012=CARTESIAN_POINT('Origin',(9.31,-4.82,78.));
#64013=CARTESIAN_POINT('Origin',(9.31,-4.82,78.));
#64014=CARTESIAN_POINT('Origin',(9.31,-4.52,78.));
#64015=CARTESIAN_POINT('Origin',(4.52,-4.52,62.));
#64016=CARTESIAN_POINT('',(4.52,4.52,64.2));
#64017=CARTESIAN_POINT('',(4.52,4.52,62.));
#64018=CARTESIAN_POINT('',(4.52,-4.52,64.2));
#64019=CARTESIAN_POINT('',(4.52,-2.26,64.2));
#64020=CARTESIAN_POINT('',(4.52,-4.52,62.));
#64021=CARTESIAN_POINT('Origin',(4.52,4.52,62.));
#64022=CARTESIAN_POINT('',(4.52,4.52,91.8));
#64023=CARTESIAN_POINT('',(4.52,4.52,62.));
#64024=CARTESIAN_POINT('',(-6.1,4.52,91.8));
#64025=CARTESIAN_POINT('',(-0.74,4.52,91.8));
#64026=CARTESIAN_POINT('',(-6.1,4.52,64.3216946934853));
#64027=CARTESIAN_POINT('',(-6.1,4.52,62.));
#64028=CARTESIAN_POINT('',(-6.1257913174651,4.52,64.2));
#64029=CARTESIAN_POINT('Origin',(-6.4,4.52,64.3216946934853));
#64030=CARTESIAN_POINT('',(14.26,4.52,64.2));
#64031=CARTESIAN_POINT('Origin',(9.31,0.,78.));
#64032=CARTESIAN_POINT('',(3.055,-13.8,78.));
#64033=CARTESIAN_POINT('Origin',(9.31,-13.8,78.));
#64034=CARTESIAN_POINT('',(3.055,0.,78.));
#64035=CARTESIAN_POINT('',(3.055,13.8,78.));
#64036=CARTESIAN_POINT('',(3.055,0.,78.));
#64037=CARTESIAN_POINT('Origin',(9.31,13.8,78.));
#64038=CARTESIAN_POINT('Origin',(-11.7,-4.3,5.5));
#64039=CARTESIAN_POINT('',(-11.9,-4.07639320225002,0.100000000000002));
#64040=CARTESIAN_POINT('',(-12.,-4.3,0.2));
#64041=CARTESIAN_POINT('Origin',(-11.7,-4.3,-0.0999999999999988));
#64042=CARTESIAN_POINT('',(-12.,-4.3,10.7));
#64043=CARTESIAN_POINT('',(-12.,-4.3,5.5));
#64044=CARTESIAN_POINT('',(-11.7,-4.,11.));
#64045=CARTESIAN_POINT('Origin',(-11.7,-4.3,11.));
#64046=CARTESIAN_POINT('',(-11.7,-4.,0.300000000000001));
#64047=CARTESIAN_POINT('',(-11.7,-4.,5.5));
#64048=CARTESIAN_POINT('Origin',(-11.7,-4.3,0.300000000000001));
#64049=CARTESIAN_POINT('Origin',(0.,-4.,11.));
#64050=CARTESIAN_POINT('',(0.,-4.,11.));
#64051=CARTESIAN_POINT('',(11.75,-4.,11.));
#64052=CARTESIAN_POINT('',(0.,-4.,5.3));
#64053=CARTESIAN_POINT('',(0.,-4.,11.));
#64054=CARTESIAN_POINT('',(-6.3,-4.,5.3));
#64055=CARTESIAN_POINT('',(10.5,-4.,5.3));
#64056=CARTESIAN_POINT('',(-6.3,-4.,0.300000000000001));
#64057=CARTESIAN_POINT('',(-6.3,-4.,5.5));
#64058=CARTESIAN_POINT('',(11.75,-4.,0.300000000000001));
#64059=CARTESIAN_POINT('Origin',(-11.85,9.5,10.85));
#64060=CARTESIAN_POINT('',(-12.,-17.5,10.7));
#64061=CARTESIAN_POINT('',(-12.,9.5,10.7));
#64062=CARTESIAN_POINT('',(-11.7,-17.5,11.));
#64063=CARTESIAN_POINT('',(-11.7,-17.5,11.));
#64064=CARTESIAN_POINT('',(-11.7,9.5,11.));
#64065=CARTESIAN_POINT('Origin',(-12.,19.,0.));
#64066=CARTESIAN_POINT('',(-12.,-17.5,0.2));
#64067=CARTESIAN_POINT('',(-12.,9.5,0.2));
#64068=CARTESIAN_POINT('',(-12.,-17.5,0.));
#64069=CARTESIAN_POINT('Origin',(-11.7,4.3,5.5));
#64070=CARTESIAN_POINT('',(-11.7,4.,11.));
#64071=CARTESIAN_POINT('',(-12.,4.3,10.7));
#64072=CARTESIAN_POINT('Origin',(-11.7,4.3,11.));
#64073=CARTESIAN_POINT('',(-12.,4.3,0.2));
#64074=CARTESIAN_POINT('',(-12.,4.3,5.5));
#64075=CARTESIAN_POINT('',(-11.9,4.07639320225002,0.1));
#64076=CARTESIAN_POINT('Origin',(-11.7,4.3,-0.0999999999999988));
#64077=CARTESIAN_POINT('',(-11.7,4.,0.300000000000001));
#64078=CARTESIAN_POINT('Origin',(-11.7,4.3,0.300000000000001));
#64079=CARTESIAN_POINT('',(-11.7,4.,5.5));
#64080=CARTESIAN_POINT('Origin',(-11.85,9.5,10.85));
#64081=CARTESIAN_POINT('',(-11.7,17.5,11.));
#64082=CARTESIAN_POINT('',(-11.7,9.5,11.));
#64083=CARTESIAN_POINT('',(-12.,17.5,10.7));
#64084=CARTESIAN_POINT('',(-11.7,17.5,11.));
#64085=CARTESIAN_POINT('',(-12.,9.5,10.7));
#64086=CARTESIAN_POINT('Origin',(-12.5,4.,11.));
#64087=CARTESIAN_POINT('',(-6.3,4.,0.300000000000001));
#64088=CARTESIAN_POINT('',(5.5,4.,0.300000000000001));
#64089=CARTESIAN_POINT('',(-6.3,4.,5.3));
#64090=CARTESIAN_POINT('',(-6.3,4.,5.5));
#64091=CARTESIAN_POINT('',(0.,4.,5.3));
#64092=CARTESIAN_POINT('',(4.25,4.,5.3));
#64093=CARTESIAN_POINT('',(0.,4.,11.));
#64094=CARTESIAN_POINT('',(0.,4.,11.));
#64095=CARTESIAN_POINT('',(5.5,4.,11.));
#64096=CARTESIAN_POINT('Origin',(5.5,4.3,0.300000000000001));
#64097=CARTESIAN_POINT('',(-11.8,4.3,0.));
#64098=CARTESIAN_POINT('Origin',(-12.1,4.3,0.300000000000001));
#64099=CARTESIAN_POINT('',(-6.3,4.3,0.));
#64100=CARTESIAN_POINT('',(5.5,4.3,0.));
#64101=CARTESIAN_POINT('Origin',(-6.3,4.3,0.300000000000001));
#64102=CARTESIAN_POINT('Origin',(-6.3,-4.3,0.3));
#64103=CARTESIAN_POINT('',(-6.3,-4.3,0.));
#64104=CARTESIAN_POINT('Origin',(-6.3,-4.3,0.300000000000001));
#64105=CARTESIAN_POINT('',(-6.,-4.3,0.3));
#64106=CARTESIAN_POINT('Origin',(-6.3,-4.3,0.3));
#64107=CARTESIAN_POINT('Origin',(-6.3,-4.3,0.3));
#64108=CARTESIAN_POINT('Origin',(-6.3,-4.3,5.5));
#64109=CARTESIAN_POINT('',(-6.,-4.3,5.));
#64110=CARTESIAN_POINT('',(-6.,-4.3,5.5));
#64111=CARTESIAN_POINT('Origin',(-6.3,-4.3,5.3));
#64112=CARTESIAN_POINT('Origin',(-6.3,4.3,0.300000000000001));
#64113=CARTESIAN_POINT('',(-6.,4.3,0.3));
#64114=CARTESIAN_POINT('Origin',(-6.3,4.3,0.300000000000001));
#64115=CARTESIAN_POINT('Origin',(-6.3,4.3,0.3));
#64116=CARTESIAN_POINT('Origin',(35.75,11.3,0.3));
#64117=CARTESIAN_POINT('',(48.,11.,0.3));
#64118=CARTESIAN_POINT('',(-6.,11.,0.3));
#64119=CARTESIAN_POINT('',(35.75,11.,0.3));
#64120=CARTESIAN_POINT('',(-6.3,11.3,0.));
#64121=CARTESIAN_POINT('Origin',(-6.3,11.3,0.3));
#64122=CARTESIAN_POINT('',(48.3,11.3,0.));
#64123=CARTESIAN_POINT('',(35.75,11.3,0.));
#64124=CARTESIAN_POINT('Origin',(48.3,11.3,0.3));
#64125=CARTESIAN_POINT('Origin',(-6.3,5.5,0.3));
#64126=CARTESIAN_POINT('',(-6.,5.5,0.3));
#64127=CARTESIAN_POINT('',(-6.3,5.5,0.));
#64128=CARTESIAN_POINT('Origin',(-6.3,4.3,5.5));
#64129=CARTESIAN_POINT('',(-6.,4.3,5.));
#64130=CARTESIAN_POINT('',(-6.,4.3,5.5));
#64131=CARTESIAN_POINT('Origin',(-6.3,4.3,5.3));
#64132=CARTESIAN_POINT('Origin',(48.3,-5.5,0.3));
#64133=CARTESIAN_POINT('',(48.,-11.,0.3));
#64134=CARTESIAN_POINT('',(48.,-5.5,0.3));
#64135=CARTESIAN_POINT('',(48.3,-11.3,0.));
#64136=CARTESIAN_POINT('',(48.3,-5.5,0.));
#64137=CARTESIAN_POINT('Origin',(48.3,-11.3,0.3));
#64138=CARTESIAN_POINT('Origin',(4.25,4.3,5.3));
#64139=CARTESIAN_POINT('',(0.,4.3,5.));
#64140=CARTESIAN_POINT('',(4.25,4.3,5.));
#64141=CARTESIAN_POINT('Origin',(0.,4.3,5.3));
#64142=CARTESIAN_POINT('Origin',(0.,0.,5.3));
#64143=CARTESIAN_POINT('',(0.,-4.3,5.));
#64144=CARTESIAN_POINT('Origin',(0.,-4.3,5.3));
#64145=CARTESIAN_POINT('Origin',(0.,0.,5.3));
#64146=CARTESIAN_POINT('Origin',(0.,0.,5.));
#64147=CARTESIAN_POINT('Origin',(10.5,-4.3,5.3));
#64148=CARTESIAN_POINT('',(10.5,-4.3,5.));
#64149=CARTESIAN_POINT('Origin',(8.75,-11.3,0.3));
#64150=CARTESIAN_POINT('',(-6.,-11.,0.3));
#64151=CARTESIAN_POINT('',(8.75,-11.,0.3));
#64152=CARTESIAN_POINT('',(-6.3,-11.3,0.));
#64153=CARTESIAN_POINT('',(8.75,-11.3,0.));
#64154=CARTESIAN_POINT('Origin',(-6.3,-11.3,0.3));
#64155=CARTESIAN_POINT('Origin',(-6.3,5.5,0.3));
#64156=CARTESIAN_POINT('',(-6.3,5.5,0.));
#64157=CARTESIAN_POINT('',(-6.,5.5,0.3));
#64158=CARTESIAN_POINT('Origin',(11.75,-4.3,0.300000000000001));
#64159=CARTESIAN_POINT('',(-11.8,-4.3,0.));
#64160=CARTESIAN_POINT('',(11.75,-4.3,0.));
#64161=CARTESIAN_POINT('Origin',(-12.1,-4.3,0.300000000000001));
#64162=CARTESIAN_POINT('Origin',(-11.9,9.5,0.1));
#64163=CARTESIAN_POINT('',(-11.8,-17.5,0.));
#64164=CARTESIAN_POINT('',(-11.8,9.5,0.));
#64165=CARTESIAN_POINT('',(-11.8,-17.5,0.));
#64166=CARTESIAN_POINT('Origin',(23.5,0.,0.));
#64167=CARTESIAN_POINT('',(-11.8,17.5,0.));
#64168=CARTESIAN_POINT('',(-11.8,9.5,0.));
#64169=CARTESIAN_POINT('',(-10.5,18.8,0.));
#64170=CARTESIAN_POINT('Origin',(-10.5,17.5,0.));
#64171=CARTESIAN_POINT('',(57.5,18.8,0.));
#64172=CARTESIAN_POINT('',(41.25,18.8,0.));
#64173=CARTESIAN_POINT('',(58.8,17.5,0.));
#64174=CARTESIAN_POINT('Origin',(57.5,17.5,0.));
#64175=CARTESIAN_POINT('',(58.8,-17.5,0.));
#64176=CARTESIAN_POINT('',(58.8,-9.5,0.));
#64177=CARTESIAN_POINT('',(57.5,-18.8,0.));
#64178=CARTESIAN_POINT('Origin',(57.5,-17.5,0.));
#64179=CARTESIAN_POINT('',(-10.5,-18.8,0.));
#64180=CARTESIAN_POINT('',(5.75,-18.8,0.));
#64181=CARTESIAN_POINT('Origin',(-10.5,-17.5,0.));
#64182=CARTESIAN_POINT('',(-9.4,-15.,0.));
#64183=CARTESIAN_POINT('Origin',(-8.,-15.,0.));
#64184=CARTESIAN_POINT('',(52.6,-15.,0.));
#64185=CARTESIAN_POINT('Origin',(54.,-15.,0.));
#64186=CARTESIAN_POINT('',(52.6,15.,0.));
#64187=CARTESIAN_POINT('Origin',(54.,15.,0.));
#64188=CARTESIAN_POINT('',(-9.4,15.,0.));
#64189=CARTESIAN_POINT('Origin',(-8.,15.,0.));
#64190=CARTESIAN_POINT('Origin',(21.,0.,5.));
#64191=CARTESIAN_POINT('',(-6.,11.,5.));
#64192=CARTESIAN_POINT('',(-6.,11.,5.));
#64193=CARTESIAN_POINT('',(48.,11.,5.));
#64194=CARTESIAN_POINT('',(48.,11.,5.));
#64195=CARTESIAN_POINT('',(48.,-11.,5.));
#64196=CARTESIAN_POINT('',(48.,-11.,5.));
#64197=CARTESIAN_POINT('',(-6.,-11.,5.));
#64198=CARTESIAN_POINT('',(-6.,-11.,5.));
#64199=CARTESIAN_POINT('',(-6.,11.,5.));
#64200=CARTESIAN_POINT('',(5.2,-2.81668763803891E-16,5.));
#64201=CARTESIAN_POINT('Origin',(7.5,0.,5.));
#64202=CARTESIAN_POINT('Origin',(-6.,11.,0.));
#64203=CARTESIAN_POINT('',(-6.,11.,0.));
#64204=CARTESIAN_POINT('Origin',(48.,11.,0.));
#64205=CARTESIAN_POINT('',(48.,11.,0.));
#64206=CARTESIAN_POINT('Origin',(-8.,-15.,10.2));
#64207=CARTESIAN_POINT('',(-9.1,-15.,10.2));
#64208=CARTESIAN_POINT('Origin',(-8.,-15.,10.2));
#64209=CARTESIAN_POINT('',(-9.4,-15.,10.5));
#64210=CARTESIAN_POINT('Origin',(-9.4,-15.,10.2));
#64211=CARTESIAN_POINT('Origin',(-8.,-15.,10.5));
#64212=CARTESIAN_POINT('Origin',(-8.,-15.,5.235));
#64213=CARTESIAN_POINT('',(-9.1,-15.,0.3));
#64214=CARTESIAN_POINT('Origin',(-8.,-15.,0.3));
#64215=CARTESIAN_POINT('',(-9.1,-15.,5.235));
#64216=CARTESIAN_POINT('Origin',(-5.75,-15.,10.5));
#64217=CARTESIAN_POINT('',(-10.25,-15.,10.5));
#64218=CARTESIAN_POINT('Origin',(-8.,-15.,10.5));
#64219=CARTESIAN_POINT('Origin',(-8.,-15.,0.3));
#64220=CARTESIAN_POINT('Origin',(-9.4,-15.,0.3));
#64221=CARTESIAN_POINT('Origin',(-8.,15.,10.2));
#64222=CARTESIAN_POINT('',(-9.1,15.,10.2));
#64223=CARTESIAN_POINT('Origin',(-8.,15.,10.2));
#64224=CARTESIAN_POINT('',(-9.4,15.,10.5));
#64225=CARTESIAN_POINT('Origin',(-9.4,15.,10.2));
#64226=CARTESIAN_POINT('Origin',(-8.,15.,10.5));
#64227=CARTESIAN_POINT('Origin',(-8.,15.,5.235));
#64228=CARTESIAN_POINT('',(-9.1,15.,0.3));
#64229=CARTESIAN_POINT('Origin',(-8.,15.,0.3));
#64230=CARTESIAN_POINT('',(-9.1,15.,5.235));
#64231=CARTESIAN_POINT('Origin',(-5.75,15.,10.5));
#64232=CARTESIAN_POINT('',(-10.25,15.,10.5));
#64233=CARTESIAN_POINT('Origin',(-8.,15.,10.5));
#64234=CARTESIAN_POINT('Origin',(-8.,15.,0.3));
#64235=CARTESIAN_POINT('Origin',(-9.4,15.,0.3));
#64236=CARTESIAN_POINT('Origin',(54.,-15.,0.3));
#64237=CARTESIAN_POINT('',(52.9,-15.,0.3));
#64238=CARTESIAN_POINT('Origin',(52.6,-15.,0.3));
#64239=CARTESIAN_POINT('Origin',(54.,-15.,0.3));
#64240=CARTESIAN_POINT('Origin',(54.,-15.,5.235));
#64241=CARTESIAN_POINT('',(52.9,-15.,10.5));
#64242=CARTESIAN_POINT('',(52.9,-15.,5.235));
#64243=CARTESIAN_POINT('Origin',(54.,-15.,10.5));
#64244=CARTESIAN_POINT('Origin',(54.,15.,0.3));
#64245=CARTESIAN_POINT('',(52.9,15.,0.3));
#64246=CARTESIAN_POINT('Origin',(52.6,15.,0.3));
#64247=CARTESIAN_POINT('Origin',(54.,15.,0.3));
#64248=CARTESIAN_POINT('Origin',(54.,15.,5.235));
#64249=CARTESIAN_POINT('',(52.9,15.,10.5));
#64250=CARTESIAN_POINT('',(52.9,15.,5.235));
#64251=CARTESIAN_POINT('Origin',(54.,15.,10.5));
#64252=CARTESIAN_POINT('Origin',(25.3,11.7,15.8789502076511));
#64253=CARTESIAN_POINT('',(25.,11.7,15.8789502076511));
#64254=CARTESIAN_POINT('',(25.3,12.,15.8789502076511));
#64255=CARTESIAN_POINT('Origin',(25.3,11.7,15.8789502076511));
#64256=CARTESIAN_POINT('',(25.0836013169029,11.7,16.0867279974984));
#64257=CARTESIAN_POINT('Origin',(25.3,11.7,15.8789502076511));
#64258=CARTESIAN_POINT('Origin',(25.3,11.7,15.8789502076511));
#64259=CARTESIAN_POINT('Origin',(25.3,-11.7,15.8789502076511));
#64260=CARTESIAN_POINT('',(25.0836013169029,-11.7,16.0867279974984));
#64261=CARTESIAN_POINT('',(25.3,-12.,15.8789502076511));
#64262=CARTESIAN_POINT('Origin',(25.3,-11.7,15.8789502076511));
#64263=CARTESIAN_POINT('',(25.,-11.7,15.8789502076511));
#64264=CARTESIAN_POINT('Origin',(25.3,-11.7,15.8789502076511));
#64265=CARTESIAN_POINT('Origin',(25.3,-11.7,15.8789502076511));
#64266=CARTESIAN_POINT('Origin',(25.3,0.,15.8789502076511));
#64267=CARTESIAN_POINT('',(25.,0.,15.8789502076511));
#64268=CARTESIAN_POINT('',(25.0836013169029,0.,16.0867279974984));
#64269=CARTESIAN_POINT('Origin',(25.3,-11.7,15.1654284885127));
#64270=CARTESIAN_POINT('',(25.,-11.7,11.0627460668062));
#64271=CARTESIAN_POINT('',(25.3,-12.,11.1063316512536));
#64272=CARTESIAN_POINT('Ctrl Pts',(25.3,-12.,11.1063316512536));
#64273=CARTESIAN_POINT('Ctrl Pts',(25.2623920424744,-12.,11.1001380359884));
#64274=CARTESIAN_POINT('Ctrl Pts',(25.2221896898711,-11.9924955895806,11.0938216843788));
#64275=CARTESIAN_POINT('Ctrl Pts',(25.1480978181083,-11.9617896898647,11.0827230314705));
#64276=CARTESIAN_POINT('Ctrl Pts',(25.114212401788,-11.9385837288878,11.0779257180335));
#64277=CARTESIAN_POINT('Ctrl Pts',(25.0610047777006,-11.8851612194794,11.0706254416663));
#64278=CARTESIAN_POINT('Ctrl Pts',(25.0380212421969,-11.8515254269881,11.0676139543331));
#64279=CARTESIAN_POINT('Ctrl Pts',(25.0075180393908,-11.7777632812766,11.0636819697985));
#64280=CARTESIAN_POINT('Ctrl Pts',(25.,-11.7376370768973,11.0627460668062));
#64281=CARTESIAN_POINT('Ctrl Pts',(25.,-11.7,11.0627460668062));
#64282=CARTESIAN_POINT('',(25.3,-12.,15.1654284885127));
#64283=CARTESIAN_POINT('',(25.,-11.7,15.1654284885127));
#64284=CARTESIAN_POINT('Origin',(2.98958333333334,-11.7,37.3005642361111));
#64285=CARTESIAN_POINT('',(32.,-12.,26.5750822305795));
#64286=CARTESIAN_POINT('',(32.,-11.7,27.4736520332184));
#64287=CARTESIAN_POINT('Ctrl Pts',(32.,-12.,26.5750822305795));
#64288=CARTESIAN_POINT('Ctrl Pts',(32.,-12.,26.6950140675156));
#64289=CARTESIAN_POINT('Ctrl Pts',(32.,-11.9912295487024,26.8263190451688));
#64290=CARTESIAN_POINT('Ctrl Pts',(32.,-11.9602181513312,27.0190335202355));
#64291=CARTESIAN_POINT('Ctrl Pts',(32.,-11.9469632164437,27.0825245437305));
#64292=CARTESIAN_POINT('Ctrl Pts',(32.,-11.9132295457478,27.2045478171391));
#64293=CARTESIAN_POINT('Ctrl Pts',(32.,-11.8929743256761,27.2631417484441));
#64294=CARTESIAN_POINT('Ctrl Pts',(32.,-11.8446924251946,27.3623327659357));
#64295=CARTESIAN_POINT('Ctrl Pts',(32.,-11.8132217751365,27.4139121820562));
#64296=CARTESIAN_POINT('Ctrl Pts',(32.,-11.7626708395818,27.4537183942209));
#64297=CARTESIAN_POINT('Ctrl Pts',(32.,-11.748290736922,27.4623826653623));
#64298=CARTESIAN_POINT('Ctrl Pts',(32.,-11.7245725726024,27.471101807326));
#64299=CARTESIAN_POINT('Ctrl Pts',(32.,-11.7112795402592,27.4736520332184));
#64300=CARTESIAN_POINT('Ctrl Pts',(32.,-11.7,27.4736520332184));
#64301=CARTESIAN_POINT('Origin',(2.98958333333334,-11.7,37.3005642361111));
#64302=CARTESIAN_POINT('Origin',(2.98958333333334,-12.,37.3005642361111));
#64303=CARTESIAN_POINT('Origin',(2.98958333333334,11.7,37.3005642361111));
#64304=CARTESIAN_POINT('',(32.,11.7,27.4736520332184));
#64305=CARTESIAN_POINT('',(32.,12.,26.5750822305795));
#64306=CARTESIAN_POINT('Ctrl Pts',(32.,11.7,27.4736520332184));
#64307=CARTESIAN_POINT('Ctrl Pts',(32.,11.7112795402592,27.4736520332184));
#64308=CARTESIAN_POINT('Ctrl Pts',(32.,11.7245725726024,27.471101807326));
#64309=CARTESIAN_POINT('Ctrl Pts',(32.,11.748290736922,27.4623826653623));
#64310=CARTESIAN_POINT('Ctrl Pts',(32.,11.7626708395818,27.4537183942209));
#64311=CARTESIAN_POINT('Ctrl Pts',(32.,11.8132217751365,27.4139121820562));
#64312=CARTESIAN_POINT('Ctrl Pts',(32.,11.8446924251946,27.3623327659357));
#64313=CARTESIAN_POINT('Ctrl Pts',(32.,11.8929743256761,27.2631417484441));
#64314=CARTESIAN_POINT('Ctrl Pts',(32.,11.9132295457478,27.2045478171391));
#64315=CARTESIAN_POINT('Ctrl Pts',(32.,11.9469632164437,27.0825245437305));
#64316=CARTESIAN_POINT('Ctrl Pts',(32.,11.9602181513312,27.0190335202355));
#64317=CARTESIAN_POINT('Ctrl Pts',(32.,11.9912295487024,26.8263190451688));
#64318=CARTESIAN_POINT('Ctrl Pts',(32.,12.,26.6950140675156));
#64319=CARTESIAN_POINT('Ctrl Pts',(32.,12.,26.5750822305795));
#64320=CARTESIAN_POINT('Origin',(2.98958333333334,12.,37.3005642361111));
#64321=CARTESIAN_POINT('Origin',(2.98958333333334,11.7,37.3005642361111));
#64322=CARTESIAN_POINT('Origin',(25.3,11.7,15.1654284885127));
#64323=CARTESIAN_POINT('',(25.3,12.,11.1063316512536));
#64324=CARTESIAN_POINT('',(25.,11.7,11.0627460668062));
#64325=CARTESIAN_POINT('Ctrl Pts',(25.,11.7,11.0627460668062));
#64326=CARTESIAN_POINT('Ctrl Pts',(25.,11.7376370768973,11.0627460668062));
#64327=CARTESIAN_POINT('Ctrl Pts',(25.0075180393908,11.7777632812766,11.0636819697985));
#64328=CARTESIAN_POINT('Ctrl Pts',(25.0380212421969,11.8515254269881,11.0676139543331));
#64329=CARTESIAN_POINT('Ctrl Pts',(25.0610047777006,11.8851612194794,11.0706254416663));
#64330=CARTESIAN_POINT('Ctrl Pts',(25.114212401788,11.9385837288878,11.0779257180335));
#64331=CARTESIAN_POINT('Ctrl Pts',(25.1480978181083,11.9617896898647,11.0827230314705));
#64332=CARTESIAN_POINT('Ctrl Pts',(25.2221896898711,11.9924955895806,11.0938216843788));
#64333=CARTESIAN_POINT('Ctrl Pts',(25.2623920424744,12.,11.1001380359884));
#64334=CARTESIAN_POINT('Ctrl Pts',(25.3,12.,11.1063316512536));
#64335=CARTESIAN_POINT('',(25.,11.7,15.1654284885127));
#64336=CARTESIAN_POINT('',(25.3,12.,15.1654284885127));
#64337=CARTESIAN_POINT('Origin',(28.5000000077377,-12.,19.2681696700813));
#64338=CARTESIAN_POINT('',(26.1702534414211,-12.,11.3));
#64339=CARTESIAN_POINT('Origin',(24.,-12.,19.));
#64340=CARTESIAN_POINT('',(26.1706823007161,-12.,11.3));
#64341=CARTESIAN_POINT('',(26.1875000038689,-12.,11.3));
#64342=CARTESIAN_POINT('',(32.,-12.,19.));
#64343=CARTESIAN_POINT('Origin',(24.0004975859988,-12.,18.9995024140012));
#64344=CARTESIAN_POINT('',(32.,-12.,19.));
#64345=CARTESIAN_POINT('Origin',(25.,0.,11.0626873069442));
#64346=CARTESIAN_POINT('',(25.,-12.025,11.0627460668062));
#64347=CARTESIAN_POINT('',(25.,0.,11.0627460668062));
#64348=CARTESIAN_POINT('',(25.,12.025,11.0627460668062));
#64349=CARTESIAN_POINT('',(25.,0.,11.0627460668062));
#64350=CARTESIAN_POINT('',(25.,12.025,11.));
#64351=CARTESIAN_POINT('',(25.,12.025,11.));
#64352=CARTESIAN_POINT('',(25.,-12.025,11.));
#64353=CARTESIAN_POINT('',(25.,0.,11.));
#64354=CARTESIAN_POINT('',(25.,-12.025,11.));
#64355=CARTESIAN_POINT('Origin',(7.25,12.3,89.3));
#64356=CARTESIAN_POINT('',(-8.49857139617605,12.6,89.3));
#64357=CARTESIAN_POINT('',(-8.5,12.3,89.));
#64358=CARTESIAN_POINT('Ctrl Pts',(-8.49857139617605,12.6,89.3));
#64359=CARTESIAN_POINT('Ctrl Pts',(-8.49893015222796,12.6,89.2623323229503));
#64360=CARTESIAN_POINT('Ctrl Pts',(-8.4992383058263,12.592472261564,89.2221531517712));
#64361=CARTESIAN_POINT('Ctrl Pts',(-8.49967287208156,12.5618564029082,89.1482390701713));
#64362=CARTESIAN_POINT('Ctrl Pts',(-8.49980314675217,12.5387682604362,89.1145041917242));
#64363=CARTESIAN_POINT('Ctrl Pts',(-8.49995174729688,12.4854962982069,89.061232229495));
#64364=CARTESIAN_POINT('Ctrl Pts',(-8.49998062468412,12.4517619778622,89.0381442166394));
#64365=CARTESIAN_POINT('Ctrl Pts',(-8.50000282006993,12.37784817429,89.0075281022651));
#64366=CARTESIAN_POINT('Ctrl Pts',(-8.5,12.3376686925819,89.));
#64367=CARTESIAN_POINT('Ctrl Pts',(-8.5,12.3,89.));
#64368=CARTESIAN_POINT('',(-9.69862382425291,12.3,89.));
#64369=CARTESIAN_POINT('',(7.25,12.3,89.));
#64370=CARTESIAN_POINT('',(-9.69862382425291,12.6,89.3));
#64371=CARTESIAN_POINT('Origin',(-9.69862382425291,12.3,89.3));
#64372=CARTESIAN_POINT('',(7.25,12.6,89.3));
#64373=CARTESIAN_POINT('Origin',(-9.69862382425291,0.,89.3));
#64374=CARTESIAN_POINT('',(-9.69862382425291,11.8685749135175,88.999999999999));
#64375=CARTESIAN_POINT('',(-9.86042062850469,11.7000210181992,89.0473702429758));
#64376=CARTESIAN_POINT('Ctrl Pts',(-9.86042062850418,11.7000210181987,89.0473702429758));
#64377=CARTESIAN_POINT('Ctrl Pts',(-9.83339601165222,11.7306347273028,89.030062318944));
#64378=CARTESIAN_POINT('Ctrl Pts',(-9.80439864031728,11.7618204016055,89.0177472843307));
#64379=CARTESIAN_POINT('Ctrl Pts',(-9.75206287401563,11.8159965452229,89.0037464949648));
#64380=CARTESIAN_POINT('Ctrl Pts',(-9.72575618919431,11.8423829851573,89.));
#64381=CARTESIAN_POINT('Ctrl Pts',(-9.69862382425277,11.8685749135171,89.));
#64382=CARTESIAN_POINT('',(-9.86042062850543,12.,89.0473702429767));
#64383=CARTESIAN_POINT('',(-9.86042062850543,0.,89.0473702429767));
#64384=CARTESIAN_POINT('',(-9.99861119878734,12.,89.302752293578));
#64385=CARTESIAN_POINT('Origin',(-9.69862382425291,12.,89.3));
#64386=CARTESIAN_POINT('',(-9.99861119878734,12.3,89.302752293578));
#64387=CARTESIAN_POINT('',(-9.99861119878734,0.,89.302752293578));
#64388=CARTESIAN_POINT('Origin',(-9.69862382425291,12.3,89.3));
#64389=CARTESIAN_POINT('',(-9.69862382425291,0.,89.));
#64390=CARTESIAN_POINT('Origin',(-9.69862382425291,12.3,89.3));
#64391=CARTESIAN_POINT('Origin',(-9.69862382425291,12.3,89.3));
#64392=CARTESIAN_POINT('Origin',(23.,12.,89.));
#64393=CARTESIAN_POINT('',(54.5,12.6,89.));
#64394=CARTESIAN_POINT('Origin',(23.,12.6,89.));
#64395=CARTESIAN_POINT('',(54.5,12.,89.));
#64396=CARTESIAN_POINT('',(54.5,12.,89.));
#64397=CARTESIAN_POINT('',(44.873285764796,12.,111.667363539935));
#64398=CARTESIAN_POINT('Origin',(23.,12.,89.));
#64399=CARTESIAN_POINT('',(44.5360362332209,11.7,111.988021736578));
#64400=CARTESIAN_POINT('Ctrl Pts',(44.5360362332209,11.7,111.988021736578));
#64401=CARTESIAN_POINT('Ctrl Pts',(44.6032500460304,11.7599031326984,111.925053329613));
#64402=CARTESIAN_POINT('Ctrl Pts',(44.6704247023372,11.8197125550768,111.861567377855));
#64403=CARTESIAN_POINT('Ctrl Pts',(44.7828052847954,11.9196471425502,111.754413327953));
#64404=CARTESIAN_POINT('Ctrl Pts',(44.8281067726021,11.9598974683211,111.710959832247));
#64405=CARTESIAN_POINT('Ctrl Pts',(44.8732857647959,12.,111.667363539935));
#64406=CARTESIAN_POINT('',(44.5360362332209,12.,111.988021736578));
#64407=CARTESIAN_POINT('',(44.5360362332209,12.,111.988021736578));
#64408=CARTESIAN_POINT('',(-8.4243682746133,12.,91.1815312377953));
#64409=CARTESIAN_POINT('Origin',(23.,12.,89.));
#64410=CARTESIAN_POINT('',(-8.42436827451122,11.7000371816704,91.1815312379487));
#64411=CARTESIAN_POINT('',(-8.42436827461331,12.,91.1815312377953));
#64412=CARTESIAN_POINT('',(-8.45008814603704,12.,90.7725562350742));
#64413=CARTESIAN_POINT('Ctrl Pts',(-8.45008814603704,12.,90.7725562350742));
#64414=CARTESIAN_POINT('Ctrl Pts',(-8.44952770606724,11.9929198577654,90.782500002218));
#64415=CARTESIAN_POINT('Ctrl Pts',(-8.44896290115791,11.9858275744744,90.792437287118));
#64416=CARTESIAN_POINT('Ctrl Pts',(-8.44108102807065,11.8874474044361,90.9299630010769));
#64417=CARTESIAN_POINT('Ctrl Pts',(-8.4330514997603,11.7942613180871,91.0564517247953));
#64418=CARTESIAN_POINT('Ctrl Pts',(-8.42436827460622,11.7000371815935,91.1815312378974));
#64419=CARTESIAN_POINT('',(-8.5,12.,89.));
#64420=CARTESIAN_POINT('Origin',(23.,12.,89.));
#64421=CARTESIAN_POINT('',(-8.5,12.,89.));
#64422=CARTESIAN_POINT('Origin',(23.,12.6,67.75));
#64423=CARTESIAN_POINT('',(55.7,12.6,89.));
#64424=CARTESIAN_POINT('Origin',(23.,12.6,89.));
#64425=CARTESIAN_POINT('',(55.7,12.6,13.5));
#64426=CARTESIAN_POINT('',(55.7,12.6,83.875));
#64427=CARTESIAN_POINT('',(54.5,12.6,13.5));
#64428=CARTESIAN_POINT('',(56.,12.6,13.5));
#64429=CARTESIAN_POINT('',(54.5,12.6,13.5));
#64430=CARTESIAN_POINT('Origin',(23.,12.3,89.));
#64431=CARTESIAN_POINT('',(56.,12.3,89.));
#64432=CARTESIAN_POINT('Origin',(23.,12.3,89.));
#64433=CARTESIAN_POINT('Origin',(55.7,12.3,89.));
#64434=CARTESIAN_POINT('Origin',(23.,0.,89.));
#64435=CARTESIAN_POINT('',(-10.,12.,89.));
#64436=CARTESIAN_POINT('Origin',(23.,12.,89.));
#64437=CARTESIAN_POINT('',(-10.,-12.,89.));
#64438=CARTESIAN_POINT('',(-10.,0.,89.));
#64439=CARTESIAN_POINT('',(-9.99861119878734,-12.,89.302752293578));
#64440=CARTESIAN_POINT('Origin',(23.,-12.,89.));
#64441=CARTESIAN_POINT('',(-9.99861119878734,-12.3,89.302752293578));
#64442=CARTESIAN_POINT('',(-9.99861119878734,0.,89.302752293578));
#64443=CARTESIAN_POINT('',(56.,-12.3,89.));
#64444=CARTESIAN_POINT('Origin',(23.,-12.3,89.));
#64445=CARTESIAN_POINT('',(56.,0.,89.));
#64446=CARTESIAN_POINT('',(-6.6697247706422,-4.82,103.446710076496));
#64447=CARTESIAN_POINT('',(4.65321100917432,-4.82,116.429825623327));
#64448=CARTESIAN_POINT('Origin',(23.,-4.82,89.));
#64449=CARTESIAN_POINT('',(-6.6697247706422,4.82,103.446710076496));
#64450=CARTESIAN_POINT('',(-6.6697247706422,0.,103.446710076496));
#64451=CARTESIAN_POINT('',(4.65321100917432,4.82,116.429825623327));
#64452=CARTESIAN_POINT('Origin',(23.,4.82,89.));
#64453=CARTESIAN_POINT('',(4.65321100917432,0.,116.429825623327));
#64454=CARTESIAN_POINT('Origin',(-9.69862382425291,0.,89.3));
#64455=CARTESIAN_POINT('',(-9.69862382425291,-11.8685749135175,88.999999999999));
#64456=CARTESIAN_POINT('',(-9.86042062850469,-11.7000210181992,89.0473702429758));
#64457=CARTESIAN_POINT('Ctrl Pts',(-9.69862382425277,-11.8685749135171,
89.));
#64458=CARTESIAN_POINT('Ctrl Pts',(-9.72575618919431,-11.8423829851573,
89.));
#64459=CARTESIAN_POINT('Ctrl Pts',(-9.75206287401563,-11.8159965452229,
89.0037464949648));
#64460=CARTESIAN_POINT('Ctrl Pts',(-9.80439864031728,-11.7618204016055,
89.0177472843307));
#64461=CARTESIAN_POINT('Ctrl Pts',(-9.83339601165223,-11.7306347273028,
89.030062318944));
#64462=CARTESIAN_POINT('Ctrl Pts',(-9.86042062850418,-11.7000210181987,
89.0473702429759));
#64463=CARTESIAN_POINT('',(-9.69862382425291,-12.3,89.));
#64464=CARTESIAN_POINT('',(-9.69862382425291,0.,89.));
#64465=CARTESIAN_POINT('Origin',(-9.69862382425291,-12.3,89.3));
#64466=CARTESIAN_POINT('',(-9.86042062850543,-12.,89.0473702429767));
#64467=CARTESIAN_POINT('Origin',(-9.69862382425291,-12.,89.3));
#64468=CARTESIAN_POINT('',(-9.86042062850543,0.,89.0473702429767));
#64469=CARTESIAN_POINT('Origin',(7.25,-12.3,89.3));
#64470=CARTESIAN_POINT('',(-8.5,-12.3,89.));
#64471=CARTESIAN_POINT('',(-8.49857139617605,-12.6,89.3));
#64472=CARTESIAN_POINT('Ctrl Pts',(-8.5,-12.3,89.));
#64473=CARTESIAN_POINT('Ctrl Pts',(-8.5,-12.3376686925819,89.));
#64474=CARTESIAN_POINT('Ctrl Pts',(-8.50000282006993,-12.37784817429,89.0075281022651));
#64475=CARTESIAN_POINT('Ctrl Pts',(-8.49998062468412,-12.4517619778622,
89.0381442166394));
#64476=CARTESIAN_POINT('Ctrl Pts',(-8.49995174729688,-12.4854962982069,
89.061232229495));
#64477=CARTESIAN_POINT('Ctrl Pts',(-8.49980314675217,-12.5387682604362,
89.1145041917242));
#64478=CARTESIAN_POINT('Ctrl Pts',(-8.49967287208156,-12.5618564029082,
89.1482390701713));
#64479=CARTESIAN_POINT('Ctrl Pts',(-8.4992383058263,-12.592472261564,89.2221531517712));
#64480=CARTESIAN_POINT('Ctrl Pts',(-8.49893015222796,-12.6,89.2623323229503));
#64481=CARTESIAN_POINT('Ctrl Pts',(-8.49857139617605,-12.6,89.3));
#64482=CARTESIAN_POINT('',(-9.69862382425291,-12.6,89.3));
#64483=CARTESIAN_POINT('',(7.25,-12.6,89.3));
#64484=CARTESIAN_POINT('Origin',(-9.69862382425291,-12.3,89.3));
#64485=CARTESIAN_POINT('',(7.25,-12.3,89.));
#64486=CARTESIAN_POINT('Origin',(-9.69862382425291,-12.3,89.3));
#64487=CARTESIAN_POINT('Origin',(-9.69862382425291,-12.3,89.3));
#64488=CARTESIAN_POINT('Origin',(23.,-12.3,89.));
#64489=CARTESIAN_POINT('',(55.7,-12.6,89.));
#64490=CARTESIAN_POINT('Origin',(23.,-12.6,89.));
#64491=CARTESIAN_POINT('Origin',(55.7,-12.3,89.));
#64492=CARTESIAN_POINT('Origin',(23.,-12.6,67.75));
#64493=CARTESIAN_POINT('',(54.5,-12.6,89.));
#64494=CARTESIAN_POINT('Origin',(23.,-12.6,89.));
#64495=CARTESIAN_POINT('',(54.5,-12.6,13.5));
#64496=CARTESIAN_POINT('',(54.5,-12.6,13.5));
#64497=CARTESIAN_POINT('',(55.7,-12.6,13.5));
#64498=CARTESIAN_POINT('',(56.,-12.6,13.5));
#64499=CARTESIAN_POINT('',(55.7,-12.6,83.875));
#64500=CARTESIAN_POINT('Origin',(23.,-12.,89.));
#64501=CARTESIAN_POINT('',(-8.5,-12.,89.));
#64502=CARTESIAN_POINT('',(-8.5,-12.,89.));
#64503=CARTESIAN_POINT('',(-8.45008814603704,-12.,90.7725562350742));
#64504=CARTESIAN_POINT('Origin',(23.,-12.,89.));
#64505=CARTESIAN_POINT('',(-8.4243682745111,-11.7000371816705,91.1815312379489));
#64506=CARTESIAN_POINT('Ctrl Pts',(-8.42436827460621,-11.7000371815934,
91.1815312378975));
#64507=CARTESIAN_POINT('Ctrl Pts',(-8.43305149973544,-11.7942613178173,
91.0564517251533));
#64508=CARTESIAN_POINT('Ctrl Pts',(-8.44108102802452,-11.8874474039008,
90.9299630018033));
#64509=CARTESIAN_POINT('Ctrl Pts',(-8.44896290111612,-11.9858275739497,
90.7924372878531));
#64510=CARTESIAN_POINT('Ctrl Pts',(-8.44952770604651,-11.9929198575035,
90.7825000025858));
#64511=CARTESIAN_POINT('Ctrl Pts',(-8.45008814603704,-12.,90.7725562350742));
#64512=CARTESIAN_POINT('',(-8.4243682746133,-12.,91.1815312377953));
#64513=CARTESIAN_POINT('',(-8.42436827461331,-12.,91.1815312377953));
#64514=CARTESIAN_POINT('',(44.5360362332209,-12.,111.988021736578));
#64515=CARTESIAN_POINT('Origin',(23.,-12.,89.));
#64516=CARTESIAN_POINT('',(44.5360362332209,-11.7,111.988021736578));
#64517=CARTESIAN_POINT('',(44.5360362332209,-12.,111.988021736578));
#64518=CARTESIAN_POINT('',(44.873285764796,-12.,111.667363539935));
#64519=CARTESIAN_POINT('Ctrl Pts',(44.873285764796,-12.,111.667363539935));
#64520=CARTESIAN_POINT('Ctrl Pts',(44.8281067726021,-11.9598974683211,111.710959832247));
#64521=CARTESIAN_POINT('Ctrl Pts',(44.7828052847954,-11.9196471425502,111.754413327953));
#64522=CARTESIAN_POINT('Ctrl Pts',(44.6704247023372,-11.8197125550768,111.861567377855));
#64523=CARTESIAN_POINT('Ctrl Pts',(44.6032500460304,-11.7599031326984,111.925053329613));
#64524=CARTESIAN_POINT('Ctrl Pts',(44.5360362332209,-11.7,111.988021736578));
#64525=CARTESIAN_POINT('',(54.5,-12.,89.));
#64526=CARTESIAN_POINT('Origin',(23.,-12.,89.));
#64527=CARTESIAN_POINT('',(54.5,-12.,89.));
#64528=CARTESIAN_POINT('Origin',(4.82,0.,116.180463572206));
#64529=CARTESIAN_POINT('',(4.52,4.57127326170559,116.180463572206));
#64530=CARTESIAN_POINT('Ctrl Pts',(4.52,4.57127326170559,116.180463572206));
#64531=CARTESIAN_POINT('Ctrl Pts',(4.52,4.59032279673937,116.214621871278));
#64532=CARTESIAN_POINT('Ctrl Pts',(4.52581302559788,4.61305103487801,116.246803205237));
#64533=CARTESIAN_POINT('Ctrl Pts',(4.54680207258012,4.66516558526338,116.309299708264));
#64534=CARTESIAN_POINT('Ctrl Pts',(4.56333143461808,4.69541449500085,116.339164914641));
#64535=CARTESIAN_POINT('Ctrl Pts',(4.60315123270544,4.75667572971404,116.390247753154));
#64536=CARTESIAN_POINT('Ctrl Pts',(4.62660338914075,4.78808658725471,116.411941289625));
#64537=CARTESIAN_POINT('Ctrl Pts',(4.65282998347464,4.81954351280017,116.429570453179));
#64538=CARTESIAN_POINT('Ctrl Pts',(4.65302042328646,4.81977175643649,116.429698147523));
#64539=CARTESIAN_POINT('Ctrl Pts',(4.65321100917433,4.82,116.429825623327));
#64540=CARTESIAN_POINT('',(4.52,-4.57127326170559,116.180463572206));
#64541=CARTESIAN_POINT('',(4.52,0.,116.180463572206));
#64542=CARTESIAN_POINT('Ctrl Pts',(4.65321100917432,-4.82,116.429825623327));
#64543=CARTESIAN_POINT('Ctrl Pts',(4.65302042470636,-4.81977175813695,116.429698148473));
#64544=CARTESIAN_POINT('Ctrl Pts',(4.65282998631353,-4.81954351619801,116.429570455082));
#64545=CARTESIAN_POINT('Ctrl Pts',(4.62660209328677,-4.78808503348141,116.411940419215));
#64546=CARTESIAN_POINT('Ctrl Pts',(4.60314888688512,-4.75667258912483,116.390245585618));
#64547=CARTESIAN_POINT('Ctrl Pts',(4.56332857524287,-4.69540962032475,116.339160391622));
#64548=CARTESIAN_POINT('Ctrl Pts',(4.54679946880003,-4.66516046552692,116.309294367754));
#64549=CARTESIAN_POINT('Ctrl Pts',(4.52581220928109,-4.61304783029562,116.246798662654));
#64550=CARTESIAN_POINT('Ctrl Pts',(4.52,-4.59032144835482,116.214619453449));
#64551=CARTESIAN_POINT('Ctrl Pts',(4.52,-4.57127326170558,116.180463572206));
#64552=CARTESIAN_POINT('Origin',(4.52,-4.52,62.));
#64553=CARTESIAN_POINT('',(4.52,4.52,115.977390533556));
#64554=CARTESIAN_POINT('Ctrl Pts',(4.52,4.57127326170559,116.180463572206));
#64555=CARTESIAN_POINT('Ctrl Pts',(4.52,4.56121444363019,116.162426800414));
#64556=CARTESIAN_POINT('Ctrl Pts',(4.52,4.5527871400801,116.143675769804));
#64557=CARTESIAN_POINT('Ctrl Pts',(4.52,4.52968731714536,116.081272993969));
#64558=CARTESIAN_POINT('Ctrl Pts',(4.52,4.52,116.024985987463));
#64559=CARTESIAN_POINT('Ctrl Pts',(4.52,4.52,115.977390533556));
#64560=CARTESIAN_POINT('',(4.52,4.52,92.));
#64561=CARTESIAN_POINT('',(4.52,4.52,62.));
#64562=CARTESIAN_POINT('',(4.52,-4.52,92.));
#64563=CARTESIAN_POINT('',(4.52,-2.26,92.));
#64564=CARTESIAN_POINT('',(4.52,-4.52,115.977390533556));
#64565=CARTESIAN_POINT('',(4.52,-4.52,62.));
#64566=CARTESIAN_POINT('Ctrl Pts',(4.52,-4.52,115.977390533556));
#64567=CARTESIAN_POINT('Ctrl Pts',(4.52,-4.52,116.024985987463));
#64568=CARTESIAN_POINT('Ctrl Pts',(4.52,-4.52968731714536,116.081272993969));
#64569=CARTESIAN_POINT('Ctrl Pts',(4.52,-4.5527871400801,116.143675769804));
#64570=CARTESIAN_POINT('Ctrl Pts',(4.52,-4.56121444363017,116.162426800414));
#64571=CARTESIAN_POINT('Ctrl Pts',(4.52,-4.57127326170558,116.180463572206));
#64572=CARTESIAN_POINT('Origin',(-9.7,0.,87.));
#64573=CARTESIAN_POINT('',(-10.,-1.35323471305783E-16,88.105));
#64574=CARTESIAN_POINT('Origin',(-10.,0.,87.));
#64575=CARTESIAN_POINT('',(-9.7,-9.85840673313618E-17,87.805));
#64576=CARTESIAN_POINT('Origin',(-9.7,-1.35323471305782E-16,88.105));
#64577=CARTESIAN_POINT('',(-9.7,9.8584067331361E-17,86.195));
#64578=CARTESIAN_POINT('Origin',(-9.7,0.,87.));
#64579=CARTESIAN_POINT('Origin',(-9.7,0.,87.));
#64580=CARTESIAN_POINT('Origin',(-10.,0.,68.));
#64581=CARTESIAN_POINT('',(-9.99999999942964,-0.470126090455401,68.0000190309882));
#64582=CARTESIAN_POINT('',(-10.,-1.35323471305783E-16,70.105));
#64583=CARTESIAN_POINT('Origin',(-10.,0.,69.));
#64584=CARTESIAN_POINT('',(-10.,-11.7,68.));
#64585=CARTESIAN_POINT('',(-10.,0.,68.));
#64586=CARTESIAN_POINT('',(-10.,-11.7,88.));
#64587=CARTESIAN_POINT('',(-10.,-11.7,64.75));
#64588=CARTESIAN_POINT('',(-10.,-12.,88.));
#64589=CARTESIAN_POINT('',(-10.,0.,88.));
#64590=CARTESIAN_POINT('',(-10.,-12.,68.));
#64591=CARTESIAN_POINT('',(-10.,12.,88.));
#64592=CARTESIAN_POINT('',(-10.,12.,68.));
#64593=CARTESIAN_POINT('',(-10.,11.7,88.));
#64594=CARTESIAN_POINT('',(-10.,0.,88.));
#64595=CARTESIAN_POINT('',(-10.,11.7,68.));
#64596=CARTESIAN_POINT('',(-10.,11.7,64.75));
#64597=CARTESIAN_POINT('',(-9.99999999942964,0.4701260904554,68.0000190309882));
#64598=CARTESIAN_POINT('',(-10.,0.,68.));
#64599=CARTESIAN_POINT('Origin',(-10.,0.,69.));
#64600=CARTESIAN_POINT('',(-10.,-1.35323471305783E-16,83.105));
#64601=CARTESIAN_POINT('Origin',(-10.,0.,82.));
#64602=CARTESIAN_POINT('',(-10.,-1.35323471305783E-16,75.105));
#64603=CARTESIAN_POINT('Origin',(-10.,0.,74.));
#64604=CARTESIAN_POINT('Origin',(-8.05,0.,87.));
#64605=CARTESIAN_POINT('',(-6.4,-9.8584067331361E-17,86.195));
#64606=CARTESIAN_POINT('Origin',(-6.4,0.,87.));
#64607=CARTESIAN_POINT('',(-8.05,-9.8584067331361E-17,86.195));
#64608=CARTESIAN_POINT('Origin',(-9.7,0.,82.));
#64609=CARTESIAN_POINT('',(-9.7,-9.85840673313618E-17,82.805));
#64610=CARTESIAN_POINT('Origin',(-9.7,-1.35323471305782E-16,83.105));
#64611=CARTESIAN_POINT('',(-9.7,9.8584067331361E-17,81.195));
#64612=CARTESIAN_POINT('Origin',(-9.7,0.,82.));
#64613=CARTESIAN_POINT('Origin',(-9.7,0.,82.));
#64614=CARTESIAN_POINT('Origin',(-8.05,0.,82.));
#64615=CARTESIAN_POINT('',(-6.4,-9.8584067331361E-17,81.195));
#64616=CARTESIAN_POINT('Origin',(-6.4,0.,82.));
#64617=CARTESIAN_POINT('',(-8.05,-9.8584067331361E-17,81.195));
#64618=CARTESIAN_POINT('Origin',(-9.7,0.,74.));
#64619=CARTESIAN_POINT('',(-9.7,-9.85840673313618E-17,74.805));
#64620=CARTESIAN_POINT('Origin',(-9.7,-1.35323471305782E-16,75.105));
#64621=CARTESIAN_POINT('',(-9.7,9.8584067331361E-17,73.195));
#64622=CARTESIAN_POINT('Origin',(-9.7,0.,74.));
#64623=CARTESIAN_POINT('Origin',(-9.7,0.,74.));
#64624=CARTESIAN_POINT('Origin',(-8.05,0.,74.));
#64625=CARTESIAN_POINT('',(-6.4,-9.8584067331361E-17,73.195));
#64626=CARTESIAN_POINT('Origin',(-6.4,0.,74.));
#64627=CARTESIAN_POINT('',(-8.05,-9.8584067331361E-17,73.195));
#64628=CARTESIAN_POINT('Origin',(-9.7,0.,69.));
#64629=CARTESIAN_POINT('Ctrl Pts',(-9.99999999942964,0.470126090455401,
68.0000190309882));
#64630=CARTESIAN_POINT('Ctrl Pts',(-9.99999998813253,0.468118427919553,
67.9992943413484));
#64631=CARTESIAN_POINT('Ctrl Pts',(-9.99999980855369,0.466342204530572,
67.9986571434586));
#64632=CARTESIAN_POINT('Ctrl Pts',(-9.99996282245433,0.273581519871146,
67.9300626849876));
#64633=CARTESIAN_POINT('Ctrl Pts',(-9.99914891965457,0.112578315718402,
67.9175814939608));
#64634=CARTESIAN_POINT('Ctrl Pts',(-9.99914891965457,-0.112578315316757,
67.9175814939608));
#64635=CARTESIAN_POINT('Ctrl Pts',(-9.99996282245425,-0.273581519475881,
67.9300626848471));
#64636=CARTESIAN_POINT('Ctrl Pts',(-9.99999980855369,-0.466342204533258,
67.9986571434596));
#64637=CARTESIAN_POINT('Ctrl Pts',(-9.99999998813253,-0.468118427917354,
67.9992943413476));
#64638=CARTESIAN_POINT('Ctrl Pts',(-9.99999999942964,-0.47012609045541,
68.0000190309882));
#64639=CARTESIAN_POINT('',(-9.7,-9.85840673313618E-17,69.805));
#64640=CARTESIAN_POINT('Origin',(-9.7,-1.35323471305782E-16,70.105));
#64641=CARTESIAN_POINT('',(-9.7,9.8584067331361E-17,68.195));
#64642=CARTESIAN_POINT('Origin',(-9.7,0.,69.));
#64643=CARTESIAN_POINT('Origin',(-9.7,0.,69.));
#64644=CARTESIAN_POINT('Origin',(-5.9999073877354,0.,68.0000926122646));
#64645=CARTESIAN_POINT('',(-6.,11.7,64.));
#64646=CARTESIAN_POINT('Ctrl Pts',(-6.,11.7,64.));
#64647=CARTESIAN_POINT('Ctrl Pts',(-6.25112253076429,11.700005814122,64.0000058141219));
#64648=CARTESIAN_POINT('Ctrl Pts',(-6.51082246976745,11.700011270506,64.0240405917389));
#64649=CARTESIAN_POINT('Ctrl Pts',(-7.02743037635765,11.7000208877413,64.1252738553641));
#64650=CARTESIAN_POINT('Ctrl Pts',(-7.28434258369625,11.7000250491913,64.2024507041098));
#64651=CARTESIAN_POINT('Ctrl Pts',(-7.7770960960606,11.7000317321778,64.4065625747948));
#64652=CARTESIAN_POINT('Ctrl Pts',(-8.01332979059301,11.7000342590358,64.5336601351113));
#64653=CARTESIAN_POINT('Ctrl Pts',(-8.45020267146997,11.7000375733931,64.8273844766965));
#64654=CARTESIAN_POINT('Ctrl Pts',(-8.65082955549268,11.7000383601839,64.9940295554927));
#64655=CARTESIAN_POINT('Ctrl Pts',(-9.00597044450735,11.7000383601839,65.3491704445074));
#64656=CARTESIAN_POINT('Ctrl Pts',(-9.17261552330358,11.7000375733931,65.5497973285301));
#64657=CARTESIAN_POINT('Ctrl Pts',(-9.46633986488873,11.7000342590358,65.986670209407));
#64658=CARTESIAN_POINT('Ctrl Pts',(-9.59343742520522,11.7000317321777,66.2229039039394));
#64659=CARTESIAN_POINT('Ctrl Pts',(-9.79754929589018,11.7000250491913,66.7156574163038));
#64660=CARTESIAN_POINT('Ctrl Pts',(-9.87472614463586,11.7000208877412,66.9725696236423));
#64661=CARTESIAN_POINT('Ctrl Pts',(-9.97595940826116,11.700011270506,67.4891775302326));
#64662=CARTESIAN_POINT('Ctrl Pts',(-9.99999418587806,11.7000058141219,67.7488774692357));
#64663=CARTESIAN_POINT('Ctrl Pts',(-10.,11.7,68.));
#64664=CARTESIAN_POINT('',(-6.,4.72,64.));
#64665=CARTESIAN_POINT('',(-6.,0.,64.));
#64666=CARTESIAN_POINT('',(-6.43243912956307,4.69654632125481,64.0234536787452));
#64667=CARTESIAN_POINT('Origin',(-5.9999073877354,0.719907387735438,68.0000926122646));
#64668=CARTESIAN_POINT('',(-6.43243912956307,-4.69654632125481,64.0234536787452));
#64669=CARTESIAN_POINT('',(-6.43243912956307,0.,64.0234536787452));
#64670=CARTESIAN_POINT('',(-6.,-4.72,64.));
#64671=CARTESIAN_POINT('Origin',(-5.9999073877354,-0.719907387735438,68.0000926122646));
#64672=CARTESIAN_POINT('',(-6.,-11.7,64.));
#64673=CARTESIAN_POINT('',(-6.,0.,64.));
#64674=CARTESIAN_POINT('Ctrl Pts',(-10.,-11.7,68.));
#64675=CARTESIAN_POINT('Ctrl Pts',(-9.9999941870305,-11.7000058129695,67.7489272452332));
#64676=CARTESIAN_POINT('Ctrl Pts',(-9.97596913895641,-11.700011268298,67.4892826274773));
#64677=CARTESIAN_POINT('Ctrl Pts',(-9.87476627167497,-11.7000208852123,
66.9727189780775));
#64678=CARTESIAN_POINT('Ctrl Pts',(-9.79759683635832,-11.7000250470742,
66.7157963928911));
#64679=CARTESIAN_POINT('Ctrl Pts',(-9.59349620678922,-11.7000317308133,
66.2230216156946));
#64680=CARTESIAN_POINT('Ctrl Pts',(-9.46640247476706,-11.7000342580129,
65.9867769970987));
#64681=CARTESIAN_POINT('Ctrl Pts',(-9.17268217075586,-11.7000375729573,
65.5498827986129));
#64682=CARTESIAN_POINT('Ctrl Pts',(-9.00603729816346,-11.7000383599935,
65.3492455223435));
#64683=CARTESIAN_POINT('Ctrl Pts',(-8.65089367384098,-11.7000383603743,
64.9940854526933));
#64684=CARTESIAN_POINT('Ctrl Pts',(-8.45026411428748,-11.7000375737319,
64.8274312897584));
#64685=CARTESIAN_POINT('Ctrl Pts',(-8.01338351700647,-11.7000342595708,
64.53369075565));
#64686=CARTESIAN_POINT('Ctrl Pts',(-7.7771447837467,-11.7000317327607,64.4065860844428));
#64687=CARTESIAN_POINT('Ctrl Pts',(-7.28437945797041,-11.7000250497688,
64.2024626371268));
#64688=CARTESIAN_POINT('Ctrl Pts',(-7.02746044639484,-11.700020888265,64.1252813050771));
#64689=CARTESIAN_POINT('Ctrl Pts',(-6.5108379773071,-11.7000112708308,64.0240420734374));
#64690=CARTESIAN_POINT('Ctrl Pts',(-6.25113027928763,-11.7000058143014,
64.0000058143013));
#64691=CARTESIAN_POINT('Ctrl Pts',(-6.,-11.7,64.));
#64692=CARTESIAN_POINT('Origin',(-8.05,0.,69.));
#64693=CARTESIAN_POINT('',(-6.4,-9.8584067331361E-17,68.195));
#64694=CARTESIAN_POINT('Origin',(-6.4,0.,69.));
#64695=CARTESIAN_POINT('',(-8.05,-9.8584067331361E-17,68.195));
#64696=CARTESIAN_POINT('Origin',(-6.4,0.,103.315376348528));
#64697=CARTESIAN_POINT('',(-6.26743038421116,4.52,103.584495833088));
#64698=CARTESIAN_POINT('Ctrl Pts',(-6.6697247706422,4.82,103.446710076496));
#64699=CARTESIAN_POINT('Ctrl Pts',(-6.6696252575399,4.81977372209222,103.446914450111));
#64700=CARTESIAN_POINT('Ctrl Pts',(-6.6695255121209,4.81954744411124,103.447118710688));
#64701=CARTESIAN_POINT('Ctrl Pts',(-6.65517755554285,4.78707393638485,103.476416233538));
#64702=CARTESIAN_POINT('Ctrl Pts',(-6.63612325427058,4.75462574198187,103.503393613814));
#64703=CARTESIAN_POINT('Ctrl Pts',(-6.58988824959697,4.6928359313211,103.5498694845));
#64704=CARTESIAN_POINT('Ctrl Pts',(-6.56262383483166,4.66300885428511,103.56987026714));
#64705=CARTESIAN_POINT('Ctrl Pts',(-6.50176857960494,4.60981011685317,103.599492331102));
#64706=CARTESIAN_POINT('Ctrl Pts',(-6.46823886939747,4.58584069575979,103.609814075921));
#64707=CARTESIAN_POINT('Ctrl Pts',(-6.40390283804146,4.55140125451023,103.61665065922));
#64708=CARTESIAN_POINT('Ctrl Pts',(-6.37449937904038,4.5391620652867,103.615845514477));
#64709=CARTESIAN_POINT('Ctrl Pts',(-6.31820829087247,4.52382192841078,103.605248291869));
#64710=CARTESIAN_POINT('Ctrl Pts',(-6.29224369239987,4.52,103.596718993883));
#64711=CARTESIAN_POINT('Ctrl Pts',(-6.26743038421117,4.52,103.584495833088));
#64712=CARTESIAN_POINT('',(-6.26743038421116,-4.52,103.584495833088));
#64713=CARTESIAN_POINT('Ctrl Pts',(-6.26743038421116,-4.52,103.584495833088));
#64714=CARTESIAN_POINT('Ctrl Pts',(-6.2922436925302,-4.52,103.596718993948));
#64715=CARTESIAN_POINT('Ctrl Pts',(-6.31820829113994,-4.52382192845083,
103.605248291956));
#64716=CARTESIAN_POINT('Ctrl Pts',(-6.37449937946708,-4.53916206544046,
103.615845514515));
#64717=CARTESIAN_POINT('Ctrl Pts',(-6.40390283848748,-4.55140125471072,
103.616650659215));
#64718=CARTESIAN_POINT('Ctrl Pts',(-6.46823886988568,-4.58584069607141,
103.609814075813));
#64719=CARTESIAN_POINT('Ctrl Pts',(-6.50176858011075,-4.60981011723393,
103.599492330925));
#64720=CARTESIAN_POINT('Ctrl Pts',(-6.5626238352147,-4.6630088546851,103.56987026688));
#64721=CARTESIAN_POINT('Ctrl Pts',(-6.58988824987319,-4.69283593165289,
103.549869484264));
#64722=CARTESIAN_POINT('Ctrl Pts',(-6.63612325437506,-4.7546257421599,103.503393613666));
#64723=CARTESIAN_POINT('Ctrl Pts',(-6.65517755560667,-4.78707393641448,
103.476416233408));
#64724=CARTESIAN_POINT('Ctrl Pts',(-6.66952551212043,-4.81954744411345,
103.447118710689));
#64725=CARTESIAN_POINT('Ctrl Pts',(-6.66962525753937,-4.819773722091,103.446914450112));
#64726=CARTESIAN_POINT('Ctrl Pts',(-6.6697247706422,-4.82,103.446710076496));
#64727=CARTESIAN_POINT('',(-6.1,-4.52,103.315376348528));
#64728=CARTESIAN_POINT('Origin',(-6.4,-4.52,103.315376348528));
#64729=CARTESIAN_POINT('',(-6.1,4.52,103.315376348528));
#64730=CARTESIAN_POINT('',(-6.1,0.,103.315376348528));
#64731=CARTESIAN_POINT('Origin',(-6.4,4.52,103.315376348528));
#64732=CARTESIAN_POINT('Origin',(-6.1,4.52,62.));
#64733=CARTESIAN_POINT('',(-6.1,-4.52,91.9987475176032));
#64734=CARTESIAN_POINT('',(-6.1,-4.52,62.));
#64735=CARTESIAN_POINT('',(-6.1,-4.71874751760316,91.9987475176032));
#64736=CARTESIAN_POINT('',(-6.1,0.,91.9987475176032));
#64737=CARTESIAN_POINT('',(-6.1,-4.52,91.8));
#64738=CARTESIAN_POINT('',(-6.1,5.14000000000013,82.1400000000004));
#64739=CARTESIAN_POINT('',(-6.1,-4.52,64.3216946934853));
#64740=CARTESIAN_POINT('',(-6.1,-4.52,62.));
#64741=CARTESIAN_POINT('',(-6.1,0.,64.3216946934853));
#64742=CARTESIAN_POINT('',(-6.1,4.71874751760317,91.9987475176032));
#64743=CARTESIAN_POINT('',(-6.1,-2.88,84.4000000000004));
#64744=CARTESIAN_POINT('',(-6.1,4.52,91.9987475176032));
#64745=CARTESIAN_POINT('',(-6.1,0.,91.9987475176032));
#64746=CARTESIAN_POINT('',(-6.1,4.52,62.));
#64747=CARTESIAN_POINT('',(-6.1,1.35323471305782E-16,67.895));
#64748=CARTESIAN_POINT('Origin',(-6.1,0.,69.));
#64749=CARTESIAN_POINT('',(-6.1,1.35323471305782E-16,80.895));
#64750=CARTESIAN_POINT('Origin',(-6.1,0.,82.));
#64751=CARTESIAN_POINT('',(-6.1,1.35323471305782E-16,85.895));
#64752=CARTESIAN_POINT('Origin',(-6.1,0.,87.));
#64753=CARTESIAN_POINT('',(-6.1,1.35323471305782E-16,72.895));
#64754=CARTESIAN_POINT('Origin',(-6.1,0.,74.));
#64755=CARTESIAN_POINT('Origin',(7.5,0.,5.3));
#64756=CARTESIAN_POINT('',(5.5,-2.44929359829471E-16,5.3));
#64757=CARTESIAN_POINT('Origin',(5.2,-2.81668763803891E-16,5.3));
#64758=CARTESIAN_POINT('Origin',(7.5,0.,5.3));
#64759=CARTESIAN_POINT('Origin',(7.5,0.,8.015));
#64760=CARTESIAN_POINT('',(5.5,2.44929359829471E-16,10.7));
#64761=CARTESIAN_POINT('',(5.5,-2.44929359829471E-16,8.015));
#64762=CARTESIAN_POINT('',(9.5,-2.44929359829471E-16,10.7));
#64763=CARTESIAN_POINT('Origin',(7.5,0.,10.7));
#64764=CARTESIAN_POINT('Origin',(7.5,0.,10.7));
#64765=CARTESIAN_POINT('Origin',(2.98958333333334,11.7,37.3005642361111));
#64766=CARTESIAN_POINT('',(18.,11.7,64.));
#64767=CARTESIAN_POINT('',(18.6030508954915,12.,64.));
#64768=CARTESIAN_POINT('Ctrl Pts',(18.,11.7,64.));
#64769=CARTESIAN_POINT('Ctrl Pts',(18.,11.713619465494,64.));
#64770=CARTESIAN_POINT('Ctrl Pts',(18.0024287979856,11.7297813438019,64.));
#64771=CARTESIAN_POINT('Ctrl Pts',(18.0106135791545,11.7575865944757,64.));
#64772=CARTESIAN_POINT('Ctrl Pts',(18.0184092824072,11.7742960137653,64.));
#64773=CARTESIAN_POINT('Ctrl Pts',(18.0495162615657,11.8244485505029,64.));
#64774=CARTESIAN_POINT('Ctrl Pts',(18.0890723943383,11.8587863834563,64.));
#64775=CARTESIAN_POINT('Ctrl Pts',(18.1815113443949,11.9183072782496,64.));
#64776=CARTESIAN_POINT('Ctrl Pts',(18.2556738060324,11.9470895942332,64.));
#64777=CARTESIAN_POINT('Ctrl Pts',(18.3630495042082,11.97583451019,64.));
#64778=CARTESIAN_POINT('Ctrl Pts',(18.411396622125,11.9852271561232,64.));
#64779=CARTESIAN_POINT('Ctrl Pts',(18.5089669840554,11.9972984211227,64.));
#64780=CARTESIAN_POINT('Ctrl Pts',(18.5581873861427,12.,64.));
#64781=CARTESIAN_POINT('Ctrl Pts',(18.6030508954915,12.,64.));
#64782=CARTESIAN_POINT('',(32.,12.,48.0260462416427));
#64783=CARTESIAN_POINT('Origin',(2.98958333333334,12.,37.3005642361111));
#64784=CARTESIAN_POINT('',(32.,11.7,47.1274764390038));
#64785=CARTESIAN_POINT('Ctrl Pts',(32.,12.,48.0260462416427));
#64786=CARTESIAN_POINT('Ctrl Pts',(32.,12.,47.9061144047066));
#64787=CARTESIAN_POINT('Ctrl Pts',(32.,11.9912295487024,47.7748094270535));
#64788=CARTESIAN_POINT('Ctrl Pts',(32.,11.9602181513312,47.5820949519867));
#64789=CARTESIAN_POINT('Ctrl Pts',(32.,11.9469632164437,47.5186039284917));
#64790=CARTESIAN_POINT('Ctrl Pts',(32.,11.9132295457478,47.3965806550831));
#64791=CARTESIAN_POINT('Ctrl Pts',(32.,11.8929743256761,47.3379867237781));
#64792=CARTESIAN_POINT('Ctrl Pts',(32.,11.8446924251946,47.2387957062865));
#64793=CARTESIAN_POINT('Ctrl Pts',(32.,11.8132217751365,47.187216290166));
#64794=CARTESIAN_POINT('Ctrl Pts',(32.,11.7626708395818,47.1474100780013));
#64795=CARTESIAN_POINT('Ctrl Pts',(32.,11.748290736922,47.1387458068599));
#64796=CARTESIAN_POINT('Ctrl Pts',(32.,11.7245725726024,47.1300266648962));
#64797=CARTESIAN_POINT('Ctrl Pts',(32.,11.7112795402592,47.1274764390039));
#64798=CARTESIAN_POINT('Ctrl Pts',(32.,11.7,47.1274764390039));
#64799=CARTESIAN_POINT('Origin',(2.98958333333334,11.7,37.3005642361111));
#64800=CARTESIAN_POINT('Origin',(2.98958333333334,0.,37.3005642361111));
#64801=CARTESIAN_POINT('',(32.,-11.7,47.1274764390038));
#64802=CARTESIAN_POINT('',(32.,0.,47.1274764390038));
#64803=CARTESIAN_POINT('',(18.,-11.7,64.));
#64804=CARTESIAN_POINT('Origin',(2.98958333333334,-11.7,37.3005642361111));
#64805=CARTESIAN_POINT('',(18.,0.,64.));
#64806=CARTESIAN_POINT('Origin',(32.,0.,56.));
#64807=CARTESIAN_POINT('',(32.,12.,56.));
#64808=CARTESIAN_POINT('',(32.,12.,19.));
#64809=CARTESIAN_POINT('',(32.,11.7,56.));
#64810=CARTESIAN_POINT('',(32.,0.,56.));
#64811=CARTESIAN_POINT('',(32.,11.7,40.25));
#64812=CARTESIAN_POINT('Origin',(2.98958333333334,-11.7,37.3005642361111));
#64813=CARTESIAN_POINT('',(32.,-12.,48.0260462416427));
#64814=CARTESIAN_POINT('Ctrl Pts',(32.,-11.7,47.1274764390039));
#64815=CARTESIAN_POINT('Ctrl Pts',(32.,-11.7112795402592,47.1274764390039));
#64816=CARTESIAN_POINT('Ctrl Pts',(32.,-11.7245725726024,47.1300266648962));
#64817=CARTESIAN_POINT('Ctrl Pts',(32.,-11.748290736922,47.1387458068599));
#64818=CARTESIAN_POINT('Ctrl Pts',(32.,-11.7626708395818,47.1474100780013));
#64819=CARTESIAN_POINT('Ctrl Pts',(32.,-11.8132217751365,47.187216290166));
#64820=CARTESIAN_POINT('Ctrl Pts',(32.,-11.8446924251946,47.2387957062865));
#64821=CARTESIAN_POINT('Ctrl Pts',(32.,-11.8929743256761,47.3379867237781));
#64822=CARTESIAN_POINT('Ctrl Pts',(32.,-11.9132295457478,47.3965806550831));
#64823=CARTESIAN_POINT('Ctrl Pts',(32.,-11.9469632164437,47.5186039284917));
#64824=CARTESIAN_POINT('Ctrl Pts',(32.,-11.9602181513312,47.5820949519868));
#64825=CARTESIAN_POINT('Ctrl Pts',(32.,-11.9912295487024,47.7748094270535));
#64826=CARTESIAN_POINT('Ctrl Pts',(32.,-12.,47.9061144047066));
#64827=CARTESIAN_POINT('Ctrl Pts',(32.,-12.,48.0260462416428));
#64828=CARTESIAN_POINT('',(18.6030508954915,-12.,64.));
#64829=CARTESIAN_POINT('Origin',(2.98958333333334,-12.,37.3005642361111));
#64830=CARTESIAN_POINT('Ctrl Pts',(18.6030508954915,-12.,64.));
#64831=CARTESIAN_POINT('Ctrl Pts',(18.5581873861427,-12.,64.));
#64832=CARTESIAN_POINT('Ctrl Pts',(18.5089669840554,-11.9972984211227,64.));
#64833=CARTESIAN_POINT('Ctrl Pts',(18.411396622125,-11.9852271561232,64.));
#64834=CARTESIAN_POINT('Ctrl Pts',(18.3630495042082,-11.97583451019,64.));
#64835=CARTESIAN_POINT('Ctrl Pts',(18.2556738060324,-11.9470895942332,64.));
#64836=CARTESIAN_POINT('Ctrl Pts',(18.1815113443949,-11.9183072782496,64.));
#64837=CARTESIAN_POINT('Ctrl Pts',(18.0890723943383,-11.8587863834563,64.));
#64838=CARTESIAN_POINT('Ctrl Pts',(18.0495162615657,-11.8244485505029,64.));
#64839=CARTESIAN_POINT('Ctrl Pts',(18.0184092824072,-11.7742960137653,64.));
#64840=CARTESIAN_POINT('Ctrl Pts',(18.0106135791545,-11.7575865944757,64.));
#64841=CARTESIAN_POINT('Ctrl Pts',(18.0024287979856,-11.7297813438019,64.));
#64842=CARTESIAN_POINT('Ctrl Pts',(18.,-11.713619465494,64.));
#64843=CARTESIAN_POINT('Ctrl Pts',(18.,-11.7,64.));
#64844=CARTESIAN_POINT('Origin',(25.0000000077377,-12.,55.5637382272397));
#64845=CARTESIAN_POINT('',(32.,-12.,56.));
#64846=CARTESIAN_POINT('',(32.,-12.,19.));
#64847=CARTESIAN_POINT('',(24.,-12.,64.));
#64848=CARTESIAN_POINT('Origin',(24.0004975859988,-12.,56.0004975859988));
#64849=CARTESIAN_POINT('',(24.,-12.,64.));
#64850=CARTESIAN_POINT('Origin',(32.,0.,56.));
#64851=CARTESIAN_POINT('',(32.,-11.7,56.));
#64852=CARTESIAN_POINT('',(32.,-11.7,40.25));
#64853=CARTESIAN_POINT('',(32.,0.,56.));
#64854=CARTESIAN_POINT('Origin',(7.5,0.,10.7));
#64855=CARTESIAN_POINT('',(9.8,-2.81668763803891E-16,11.));
#64856=CARTESIAN_POINT('Origin',(7.5,0.,11.));
#64857=CARTESIAN_POINT('Origin',(9.8,-2.81668763803891E-16,10.7));
#64858=CARTESIAN_POINT('Origin',(23.5,0.,11.));
#64859=CARTESIAN_POINT('Origin',(0.,0.,11.));
#64860=CARTESIAN_POINT('',(-10.5,-18.7,11.));
#64861=CARTESIAN_POINT('Origin',(-10.5,-17.5,11.));
#64862=CARTESIAN_POINT('',(57.5,-18.7,11.));
#64863=CARTESIAN_POINT('',(5.75,-18.7,11.));
#64864=CARTESIAN_POINT('',(58.7,-17.5,11.));
#64865=CARTESIAN_POINT('Origin',(57.5,-17.5,11.));
#64866=CARTESIAN_POINT('',(58.7,17.5,11.));
#64867=CARTESIAN_POINT('',(58.7,-9.5,11.));
#64868=CARTESIAN_POINT('',(57.5,18.7,11.));
#64869=CARTESIAN_POINT('Origin',(57.5,17.5,11.));
#64870=CARTESIAN_POINT('',(-10.5,18.7,11.));
#64871=CARTESIAN_POINT('',(41.25,18.7,11.));
#64872=CARTESIAN_POINT('Origin',(-10.5,17.5,11.));
#64873=CARTESIAN_POINT('',(-10.25,-15.,11.));
#64874=CARTESIAN_POINT('Origin',(-8.,-15.,11.));
#64875=CARTESIAN_POINT('',(51.75,-15.,11.));
#64876=CARTESIAN_POINT('Origin',(54.,-15.,11.));
#64877=CARTESIAN_POINT('',(-10.25,15.,11.));
#64878=CARTESIAN_POINT('Origin',(-8.,15.,11.));
#64879=CARTESIAN_POINT('',(51.75,15.,11.));
#64880=CARTESIAN_POINT('Origin',(54.,15.,11.));
#64881=CARTESIAN_POINT('',(24.,12.3,11.));
#64882=CARTESIAN_POINT('',(24.,12.025,11.));
#64883=CARTESIAN_POINT('',(24.,0.,11.));
#64884=CARTESIAN_POINT('',(58.5,12.3,11.));
#64885=CARTESIAN_POINT('',(23.875,12.3,11.));
#64886=CARTESIAN_POINT('',(58.5,12.025,11.));
#64887=CARTESIAN_POINT('',(58.5,0.,11.));
#64888=CARTESIAN_POINT('',(-20.,12.025,11.));
#64889=CARTESIAN_POINT('',(25.,0.,11.));
#64890=CARTESIAN_POINT('',(58.5,-12.025,11.));
#64891=CARTESIAN_POINT('',(-20.,-12.025,11.));
#64892=CARTESIAN_POINT('',(58.5,-12.3,11.));
#64893=CARTESIAN_POINT('',(58.5,0.,11.));
#64894=CARTESIAN_POINT('',(24.,-12.3,11.));
#64895=CARTESIAN_POINT('',(23.875,-12.3,11.));
#64896=CARTESIAN_POINT('',(24.,-12.025,11.));
#64897=CARTESIAN_POINT('',(24.,0.,11.));
#64898=CARTESIAN_POINT('',(-20.,-12.025,11.));
#64899=CARTESIAN_POINT('',(-20.,12.025,11.));
#64900=CARTESIAN_POINT('Origin',(-6.4,0.,64.3216946934853));
#64901=CARTESIAN_POINT('',(-6.1257913174651,-4.52,64.2));
#64902=CARTESIAN_POINT('Origin',(-6.4,-4.52,64.3216946934853));
#64903=CARTESIAN_POINT('Origin',(-6.4,-4.39830530651473,64.3216946934853));
#64904=CARTESIAN_POINT('Origin',(-6.4,4.39830530651473,64.3216946934853));
#64905=CARTESIAN_POINT('Origin',(-6.4,0.,69.));
#64906=CARTESIAN_POINT('Origin',(-6.4,-1.35323471305782E-16,67.895));
#64907=CARTESIAN_POINT('Origin',(-6.4,0.,74.));
#64908=CARTESIAN_POINT('Origin',(-6.4,-1.35323471305782E-16,72.895));
#64909=CARTESIAN_POINT('Origin',(-6.4,0.,82.));
#64910=CARTESIAN_POINT('Origin',(-6.4,-1.35323471305782E-16,80.895));
#64911=CARTESIAN_POINT('Origin',(-6.4,0.,87.));
#64912=CARTESIAN_POINT('Origin',(-6.4,-1.35323471305782E-16,85.895));
#64913=CARTESIAN_POINT('Origin',(55.7,0.,13.7767804169048));
#64914=CARTESIAN_POINT('',(55.8157264050162,12.5767804169048,13.5));
#64915=CARTESIAN_POINT('',(56.,12.3,13.7767804169048));
#64916=CARTESIAN_POINT('Origin',(55.7,12.3,13.7767804169048));
#64917=CARTESIAN_POINT('',(56.,-12.3,13.7767804169048));
#64918=CARTESIAN_POINT('',(56.,0.,13.7767804169048));
#64919=CARTESIAN_POINT('',(55.8157264050162,-12.5767804169048,13.5));
#64920=CARTESIAN_POINT('Origin',(55.7,-12.3,13.7767804169048));
#64921=CARTESIAN_POINT('',(55.8157264050162,-11.8842735949838,13.5));
#64922=CARTESIAN_POINT('',(55.8157264050162,0.,13.5));
#64923=CARTESIAN_POINT('',(55.7241152569761,-11.9759739037501,13.4777512304013));
#64924=CARTESIAN_POINT('Ctrl Pts',(55.8157264050162,-11.8842735949838,13.5));
#64925=CARTESIAN_POINT('Ctrl Pts',(55.8154916174147,-11.8845083825853,13.4999018314758));
#64926=CARTESIAN_POINT('Ctrl Pts',(55.8152567556258,-11.8847432497585,13.4998039828686));
#64927=CARTESIAN_POINT('Ctrl Pts',(55.7851007909116,-11.9149005830658,13.4872853308607));
#64928=CARTESIAN_POINT('Ctrl Pts',(55.7539530047584,-11.9461178286373,13.4801575003837));
#64929=CARTESIAN_POINT('Ctrl Pts',(55.7241152569761,-11.9759739037501,13.4777512304013));
#64930=CARTESIAN_POINT('',(55.7241152569761,11.9759739037501,13.4777512304013));
#64931=CARTESIAN_POINT('',(55.7241152569761,0.,13.4777512304013));
#64932=CARTESIAN_POINT('',(55.8157264050162,11.8842735949838,13.5));
#64933=CARTESIAN_POINT('Ctrl Pts',(55.7241152569761,11.9759739037501,13.4777512304013));
#64934=CARTESIAN_POINT('Ctrl Pts',(55.7539530047584,11.9461178286373,13.4801575003837));
#64935=CARTESIAN_POINT('Ctrl Pts',(55.7851007909116,11.9149005830658,13.4872853308607));
#64936=CARTESIAN_POINT('Ctrl Pts',(55.8152567556258,11.8847432497585,13.4998039828686));
#64937=CARTESIAN_POINT('Ctrl Pts',(55.8154916174147,11.8845083825853,13.4999018314758));
#64938=CARTESIAN_POINT('Ctrl Pts',(55.8157264050162,11.8842735949838,13.5));
#64939=CARTESIAN_POINT('',(55.8157264050162,0.,13.5));
#64940=CARTESIAN_POINT('Origin',(55.7,12.3,83.875));
#64941=CARTESIAN_POINT('Origin',(55.7,12.3,13.5));
#64942=CARTESIAN_POINT('',(56.,12.3,83.875));
#64943=CARTESIAN_POINT('Origin',(56.,12.,13.5));
#64944=CARTESIAN_POINT('',(55.7,12.,13.5));
#64945=CARTESIAN_POINT('',(56.,11.7,13.5));
#64946=CARTESIAN_POINT('',(54.5,12.,13.5));
#64947=CARTESIAN_POINT('',(40.125,12.,13.5));
#64948=CARTESIAN_POINT('',(54.5,12.,13.5));
#64949=CARTESIAN_POINT('Origin',(58.5,11.85,13.5));
#64950=CARTESIAN_POINT('',(55.7001044519953,12.,13.4758148751609));
#64951=CARTESIAN_POINT('Ctrl Pts',(55.7241152569761,11.9759739037501,13.4777512304013));
#64952=CARTESIAN_POINT('Ctrl Pts',(55.7121615840951,11.9879349189719,13.4767872245238));
#64953=CARTESIAN_POINT('Ctrl Pts',(55.7001044519953,12.,13.4758148751609));
#64954=CARTESIAN_POINT('Origin',(58.5,12.,13.5));
#64955=CARTESIAN_POINT('Origin',(25.,0.,11.));
#64956=CARTESIAN_POINT('',(55.7001044519953,-12.,13.4758148751609));
#64957=CARTESIAN_POINT('Ctrl Pts',(55.7001044519953,-12.,13.4758148751609));
#64958=CARTESIAN_POINT('Ctrl Pts',(55.7121615840951,-11.9879349189719,13.4767872245238));
#64959=CARTESIAN_POINT('Ctrl Pts',(55.7241152569761,-11.9759739037501,13.4777512304013));
#64960=CARTESIAN_POINT('',(32.44,-12.,11.6));
#64961=CARTESIAN_POINT('',(26.6505556991471,-12.,11.1331093305764));
#64962=CARTESIAN_POINT('',(31.6915937956643,-12.025,11.5396446609407));
#64963=CARTESIAN_POINT('',(24.7539493851376,-12.2567472907873,10.9801572084788));
#64964=CARTESIAN_POINT('',(56.,-12.025,13.5));
#64965=CARTESIAN_POINT('',(31.6915937956643,12.025,11.5396446609407));
#64966=CARTESIAN_POINT('',(56.,12.025,13.5));
#64967=CARTESIAN_POINT('',(32.44,12.,11.6));
#64968=CARTESIAN_POINT('',(24.7539493851376,12.2567472907873,10.9801572084788));
#64969=CARTESIAN_POINT('',(26.6505556991471,12.,11.1331093305764));
#64970=CARTESIAN_POINT('Origin',(56.,0.,100.));
#64971=CARTESIAN_POINT('',(56.,-12.3,83.875));
#64972=CARTESIAN_POINT('Origin',(23.,-4.82,89.));
#64973=CARTESIAN_POINT('Origin',(23.,-4.52,89.));
#64974=CARTESIAN_POINT('Origin',(-6.1,-4.52,62.));
#64975=CARTESIAN_POINT('',(-6.,-4.52,92.));
#64976=CARTESIAN_POINT('',(10.45,-4.52,92.));
#64977=CARTESIAN_POINT('Origin',(-5.9999073877354,-4.52,87.9999073877354));
#64978=CARTESIAN_POINT('Origin',(23.,4.82,89.));
#64979=CARTESIAN_POINT('Origin',(23.,4.52,89.));
#64980=CARTESIAN_POINT('Origin',(4.52,4.52,62.));
#64981=CARTESIAN_POINT('',(-6.,4.52,92.));
#64982=CARTESIAN_POINT('Origin',(-5.9999073877354,4.52,87.9999073877354));
#64983=CARTESIAN_POINT('',(15.76,4.52,92.));
#64984=CARTESIAN_POINT('Origin',(55.7,-12.3,83.875));
#64985=CARTESIAN_POINT('Origin',(55.7,-12.3,13.5));
#64986=CARTESIAN_POINT('Origin',(56.,-12.,13.5));
#64987=CARTESIAN_POINT('',(54.5,-12.,13.5));
#64988=CARTESIAN_POINT('',(54.5,-12.,13.5));
#64989=CARTESIAN_POINT('',(55.7,-12.,13.5));
#64990=CARTESIAN_POINT('',(40.125,-12.,13.5));
#64991=CARTESIAN_POINT('',(56.,-11.7,13.5));
#64992=CARTESIAN_POINT('Origin',(54.5,-12.,13.5));
#64993=CARTESIAN_POINT('',(54.5,-12.,37.5));
#64994=CARTESIAN_POINT('Origin',(-8.5,-12.,89.));
#64995=CARTESIAN_POINT('',(-9.56230262611138,-12.,89.));
#64996=CARTESIAN_POINT('Ctrl Pts',(-9.56230262611138,-12.,89.));
#64997=CARTESIAN_POINT('Ctrl Pts',(-9.62927380717335,-11.9355211853595,
88.9999999999994));
#64998=CARTESIAN_POINT('Ctrl Pts',(-9.69862382425291,-11.8685749135175,
88.999999999999));
#64999=CARTESIAN_POINT('',(7.875,-12.,89.));
#65000=CARTESIAN_POINT('Origin',(-5.99999999999999,-11.85,88.));
#65001=CARTESIAN_POINT('',(-9.87296247153814,-11.7000202118089,88.9999999999986));
#65002=CARTESIAN_POINT('Ctrl Pts',(-9.86042062850558,-11.7000210181973,
89.0473702429761));
#65003=CARTESIAN_POINT('Ctrl Pts',(-9.86470019847172,-11.7000207520943,
89.0315975247012));
#65004=CARTESIAN_POINT('Ctrl Pts',(-9.86888098571992,-11.700020483277,89.0158063555326));
#65005=CARTESIAN_POINT('Ctrl Pts',(-9.8729624715378,-11.7000202118089,88.9999999999985));
#65006=CARTESIAN_POINT('Ctrl Pts',(-9.87296247153813,-11.7000202118089,
88.9999999999972));
#65007=CARTESIAN_POINT('Ctrl Pts',(-9.8927585501957,-11.7000188951308,88.9233357969584));
#65008=CARTESIAN_POINT('Ctrl Pts',(-9.91021935852739,-11.7000175158046,
88.8463010263897));
#65009=CARTESIAN_POINT('Ctrl Pts',(-9.9759579265626,-11.7000112708308,88.5108379773071));
#65010=CARTESIAN_POINT('Ctrl Pts',(-9.99999418569865,-11.7000058143013,
88.2511302792877));
#65011=CARTESIAN_POINT('Ctrl Pts',(-10.,-11.7,88.));
#65012=CARTESIAN_POINT('',(-9.7,-12.,88.));
#65013=CARTESIAN_POINT('',(-10.,-11.7,88.));
#65014=CARTESIAN_POINT('Origin',(-5.99999999999999,-12.,88.));
#65015=CARTESIAN_POINT('Origin',(-5.99999999999999,-11.85,88.));
#65016=CARTESIAN_POINT('',(-6.,-12.,91.7));
#65017=CARTESIAN_POINT('Origin',(-5.99999999999999,-12.,88.));
#65018=CARTESIAN_POINT('',(-6.,-11.7,92.));
#65019=CARTESIAN_POINT('',(-6.,-11.7,92.));
#65020=CARTESIAN_POINT('Ctrl Pts',(-6.,-11.7,92.));
#65021=CARTESIAN_POINT('Ctrl Pts',(-6.25107275476676,-11.7000058129695,
91.9999941870305));
#65022=CARTESIAN_POINT('Ctrl Pts',(-6.51071737252271,-11.700011268298,91.9759691389564));
#65023=CARTESIAN_POINT('Ctrl Pts',(-7.02728102192247,-11.7000208852123,
91.874766271675));
#65024=CARTESIAN_POINT('Ctrl Pts',(-7.28420360710883,-11.7000250470743,
91.7975968363583));
#65025=CARTESIAN_POINT('Ctrl Pts',(-7.77697838430535,-11.7000317308133,
91.5934962067892));
#65026=CARTESIAN_POINT('Ctrl Pts',(-8.01322300290132,-11.7000342580129,
91.4664024747671));
#65027=CARTESIAN_POINT('Ctrl Pts',(-8.29756107931325,-11.7000364154344,
91.2752443716494));
#65028=CARTESIAN_POINT('Ctrl Pts',(-8.36185049180696,-11.7000368371963,
91.2291710362983));
#65029=CARTESIAN_POINT('Ctrl Pts',(-8.42436827442,-11.7000371816705,91.1815312379426));
#65030=CARTESIAN_POINT('Origin',(24.25,-12.,61.5));
#65031=CARTESIAN_POINT('',(-9.7,-12.,68.));
#65032=CARTESIAN_POINT('',(-9.7,-12.,64.75));
#65033=CARTESIAN_POINT('',(-6.,-12.,64.3));
#65034=CARTESIAN_POINT('Origin',(-5.99999999999999,-12.,68.));
#65035=CARTESIAN_POINT('',(24.,-12.,64.3));
#65036=CARTESIAN_POINT('',(24.125,-12.,64.3));
#65037=CARTESIAN_POINT('',(32.3,-12.,56.));
#65038=CARTESIAN_POINT('Origin',(24.,-12.,56.));
#65039=CARTESIAN_POINT('',(32.3,-12.,19.));
#65040=CARTESIAN_POINT('',(32.3,-12.,40.25));
#65041=CARTESIAN_POINT('',(27.7589892258425,-12.,11.6));
#65042=CARTESIAN_POINT('Origin',(24.,-12.,19.));
#65043=CARTESIAN_POINT('',(24.0625,-12.,11.6));
#65044=CARTESIAN_POINT('Origin',(58.5,-12.,13.5));
#65045=CARTESIAN_POINT('',(32.3,-12.,100.));
#65046=CARTESIAN_POINT('Origin',(44.,-12.,100.));
#65047=CARTESIAN_POINT('',(32.3,-12.,97.));
#65048=CARTESIAN_POINT('',(32.3,-12.,79.25));
#65049=CARTESIAN_POINT('',(27.,-12.,91.7));
#65050=CARTESIAN_POINT('Origin',(27.,-12.,97.));
#65051=CARTESIAN_POINT('',(9.125,-12.,91.7));
#65052=CARTESIAN_POINT('',(40.6103012561798,-12.,83.4957704544067));
#65053=CARTESIAN_POINT('',(41.4561398029327,-12.,85.8598899841309));
#65054=CARTESIAN_POINT('Ctrl Pts',(40.6103012561798,-12.,83.4957704544067));
#65055=CARTESIAN_POINT('Ctrl Pts',(40.6103012561798,-12.,85.0140514373779));
#65056=CARTESIAN_POINT('Ctrl Pts',(41.4561398029327,-12.,85.8598899841309));
#65057=CARTESIAN_POINT('',(43.8118011951447,-12.,86.7057290077209));
#65058=CARTESIAN_POINT('Ctrl Pts',(41.4561398029327,-12.,85.8598899841309));
#65059=CARTESIAN_POINT('Ctrl Pts',(42.3019783496857,-12.,86.7057290077209));
#65060=CARTESIAN_POINT('Ctrl Pts',(43.8118011951447,-12.,86.7057290077209));
#65061=CARTESIAN_POINT('',(46.1970684528351,-12.,85.874692440033));
#65062=CARTESIAN_POINT('Ctrl Pts',(43.8118011951447,-12.,86.7057290077209));
#65063=CARTESIAN_POINT('Ctrl Pts',(45.35968708992,-12.,86.7057290077209));
#65064=CARTESIAN_POINT('Ctrl Pts',(46.1970684528351,-12.,85.874692440033));
#65065=CARTESIAN_POINT('',(47.0344479084015,-12.,83.5465202331543));
#65066=CARTESIAN_POINT('Ctrl Pts',(46.1970684528351,-12.,85.874692440033));
#65067=CARTESIAN_POINT('Ctrl Pts',(47.0344479084015,-12.,85.0436553955078));
#65068=CARTESIAN_POINT('Ctrl Pts',(47.0344479084015,-12.,83.5465202331543));
#65069=CARTESIAN_POINT('',(46.6686222553253,-12.,81.7639150619507));
#65070=CARTESIAN_POINT('Ctrl Pts',(47.0344479084015,-12.,83.5465202331543));
#65071=CARTESIAN_POINT('Ctrl Pts',(47.0344479084015,-12.,82.4596176147461));
#65072=CARTESIAN_POINT('Ctrl Pts',(46.6686222553253,-12.,81.7639150619507));
#65073=CARTESIAN_POINT('',(45.611323595047,-12.,80.6812410354614));
#65074=CARTESIAN_POINT('Ctrl Pts',(46.6686222553253,-12.,81.7639150619507));
#65075=CARTESIAN_POINT('Ctrl Pts',(46.3027966022491,-12.,81.0682125091553));
#65076=CARTESIAN_POINT('Ctrl Pts',(45.611323595047,-12.,80.6812410354614));
#65077=CARTESIAN_POINT('',(43.8879272937775,-12.,80.2942695617676));
#65078=CARTESIAN_POINT('Ctrl Pts',(45.611323595047,-12.,80.6812410354614));
#65079=CARTESIAN_POINT('Ctrl Pts',(44.9198505878448,-12.,80.2942695617676));
#65080=CARTESIAN_POINT('Ctrl Pts',(43.8879272937775,-12.,80.2942695617676));
#65081=CARTESIAN_POINT('',(42.1518423557281,-12.,80.6283760070801));
#65082=CARTESIAN_POINT('Ctrl Pts',(43.8879272937775,-12.,80.2942695617676));
#65083=CARTESIAN_POINT('Ctrl Pts',(42.8390867710114,-12.,80.2942695617676));
#65084=CARTESIAN_POINT('Ctrl Pts',(42.1518423557281,-12.,80.6283760070801));
#65085=CARTESIAN_POINT('',(41.0374491214752,-12.,81.6856746673584));
#65086=CARTESIAN_POINT('Ctrl Pts',(42.1518423557281,-12.,80.6283760070801));
#65087=CARTESIAN_POINT('Ctrl Pts',(41.4645979404449,-12.,80.9624824523926));
#65088=CARTESIAN_POINT('Ctrl Pts',(41.0374491214752,-12.,81.6856746673584));
#65089=CARTESIAN_POINT('Ctrl Pts',(41.0374491214752,-12.,81.6856746673584));
#65090=CARTESIAN_POINT('Ctrl Pts',(40.6103012561798,-12.,82.4088668823242));
#65091=CARTESIAN_POINT('Ctrl Pts',(40.6103012561798,-12.,83.4957704544067));
#65092=CARTESIAN_POINT('',(47.7322647571564,-12.,82.1255111694336));
#65093=CARTESIAN_POINT('',(49.5719635486603,-12.,82.1255111694336));
#65094=CARTESIAN_POINT('',(36.9109817743301,-12.,82.1255111694336));
#65095=CARTESIAN_POINT('',(49.5719635486603,-12.,80.3999996185303));
#65096=CARTESIAN_POINT('',(49.5719635486603,-12.,70.9499998092651));
#65097=CARTESIAN_POINT('',(47.7322647571564,-12.,80.3999996185303));
#65098=CARTESIAN_POINT('',(35.9911323785782,-12.,80.3999996185303));
#65099=CARTESIAN_POINT('',(47.7322647571564,-12.,71.8127555847168));
#65100=CARTESIAN_POINT('',(-0.990000000000002,-12.,78.));
#65101=CARTESIAN_POINT('Origin',(9.31,-12.,78.));
#65102=CARTESIAN_POINT('',(33.6490461826324,-12.,86.5999994277954));
#65103=CARTESIAN_POINT('',(35.4379951953888,-12.,86.5999994277954));
#65104=CARTESIAN_POINT('',(29.8439975976944,-12.,86.5999994277954));
#65105=CARTESIAN_POINT('',(37.772510766983,-12.,83.1698579788208));
#65106=CARTESIAN_POINT('',(40.6718459545618,-12.,78.9098179420808));
#65107=CARTESIAN_POINT('',(37.772510766983,-12.,86.5999994277954));
#65108=CARTESIAN_POINT('',(37.772510766983,-12.,74.0499997138977));
#65109=CARTESIAN_POINT('',(39.5783770084381,-12.,86.5999994277954));
#65110=CARTESIAN_POINT('',(31.9141885042191,-12.,86.5999994277954));
#65111=CARTESIAN_POINT('',(39.5783770084381,-12.,80.3999996185303));
#65112=CARTESIAN_POINT('',(39.5783770084381,-12.,70.9499998092651));
#65113=CARTESIAN_POINT('',(37.772510766983,-12.,80.3999996185303));
#65114=CARTESIAN_POINT('',(31.0112553834915,-12.,80.3999996185303));
#65115=CARTESIAN_POINT('',(35.4506828784943,-12.,83.8042373657227));
#65116=CARTESIAN_POINT('',(38.8639403839799,-12.,78.7997578783887));
#65117=CARTESIAN_POINT('',(35.4506828784943,-12.,80.3999996185303));
#65118=CARTESIAN_POINT('',(35.4506828784943,-12.,70.9499998092651));
#65119=CARTESIAN_POINT('',(33.6490461826324,-12.,80.3999996185303));
#65120=CARTESIAN_POINT('',(28.9495230913162,-12.,80.3999996185303));
#65121=CARTESIAN_POINT('',(33.6490461826324,-12.,74.0499997138977));
#65122=CARTESIAN_POINT('',(54.3509571552277,-12.,86.7057294845581));
#65123=CARTESIAN_POINT('',(54.3509571552277,-12.,80.3999996185303));
#65124=CARTESIAN_POINT('',(54.3509571552277,-12.,70.9499998092651));
#65125=CARTESIAN_POINT('',(52.6085274219513,-12.,80.3999996185303));
#65126=CARTESIAN_POINT('',(38.4292637109756,-12.,80.3999996185303));
#65127=CARTESIAN_POINT('',(52.6085274219513,-12.,84.5319232940674));
#65128=CARTESIAN_POINT('',(52.6085274219513,-12.,73.0159616470337));
#65129=CARTESIAN_POINT('',(51.7901794910431,-12.,84.0117321014404));
#65130=CARTESIAN_POINT('Ctrl Pts',(52.6085274219513,-12.,84.5319232940674));
#65131=CARTESIAN_POINT('Ctrl Pts',(52.1856091022491,-12.,84.2105045318604));
#65132=CARTESIAN_POINT('Ctrl Pts',(51.7901794910431,-12.,84.0117321014404));
#65133=CARTESIAN_POINT('',(50.7984325885773,-12.,83.6311044692993));
#65134=CARTESIAN_POINT('Ctrl Pts',(51.7901794910431,-12.,84.0117321014404));
#65135=CARTESIAN_POINT('Ctrl Pts',(51.394749879837,-12.,83.8129596710205));
#65136=CARTESIAN_POINT('Ctrl Pts',(50.7984325885773,-12.,83.6311044692993));
#65137=CARTESIAN_POINT('',(50.7984325885773,-12.,85.0436553955078));
#65138=CARTESIAN_POINT('',(50.7984325885773,-12.,73.2718276977539));
#65139=CARTESIAN_POINT('',(52.1644623279572,-12.,85.7245559692383));
#65140=CARTESIAN_POINT('Ctrl Pts',(50.7984325885773,-12.,85.0436553955078));
#65141=CARTESIAN_POINT('Ctrl Pts',(51.6781055927277,-12.,85.3270111083984));
#65142=CARTESIAN_POINT('Ctrl Pts',(52.1644623279572,-12.,85.7245559692383));
#65143=CARTESIAN_POINT('',(52.9257175922394,-12.,86.7057294845581));
#65144=CARTESIAN_POINT('Ctrl Pts',(52.1644623279572,-12.,85.7245559692383));
#65145=CARTESIAN_POINT('Ctrl Pts',(52.6508209705353,-12.,86.122100353241));
#65146=CARTESIAN_POINT('Ctrl Pts',(52.9257175922394,-12.,86.7057294845581));
#65147=CARTESIAN_POINT('',(39.3004785776138,-12.,86.7057294845581));
#65148=CARTESIAN_POINT('Origin',(-5.9999073877354,0.,87.9999073877354));
#65149=CARTESIAN_POINT('Origin',(-5.9999073877354,-12.,87.9999073877354));
#65150=CARTESIAN_POINT('Origin',(18.5190608795662,-12.,105.));
#65151=CARTESIAN_POINT('Origin',(-8.5,12.,89.));
#65152=CARTESIAN_POINT('',(-9.56230262611138,12.,89.));
#65153=CARTESIAN_POINT('',(7.875,12.,89.));
#65154=CARTESIAN_POINT('Ctrl Pts',(-9.69862382425291,11.8685749135175,88.999999999999));
#65155=CARTESIAN_POINT('Ctrl Pts',(-9.62927380717316,11.9355211853597,88.9999999999994));
#65156=CARTESIAN_POINT('Ctrl Pts',(-9.56230262611138,12.,89.));
#65157=CARTESIAN_POINT('Origin',(54.5,12.,13.5));
#65158=CARTESIAN_POINT('',(54.5,12.,37.5));
#65159=CARTESIAN_POINT('Origin',(44.,0.,100.));
#65160=CARTESIAN_POINT('',(32.,11.7,100.));
#65161=CARTESIAN_POINT('Origin',(44.,11.7,100.));
#65162=CARTESIAN_POINT('',(32.,12.,100.));
#65163=CARTESIAN_POINT('',(32.,0.,100.));
#65164=CARTESIAN_POINT('Origin',(44.,12.,100.));
#65165=CARTESIAN_POINT('Origin',(44.,11.85,100.));
#65166=CARTESIAN_POINT('',(32.3,12.,100.));
#65167=CARTESIAN_POINT('Origin',(44.,12.,100.));
#65168=CARTESIAN_POINT('',(32.,11.7,100.));
#65169=CARTESIAN_POINT('Origin',(24.25,12.,61.5));
#65170=CARTESIAN_POINT('',(27.7589892258425,12.,11.6));
#65171=CARTESIAN_POINT('',(24.0625,12.,11.6));
#65172=CARTESIAN_POINT('',(32.3,12.,19.));
#65173=CARTESIAN_POINT('Origin',(24.,12.,19.));
#65174=CARTESIAN_POINT('',(32.3,12.,56.));
#65175=CARTESIAN_POINT('',(32.3,12.,40.25));
#65176=CARTESIAN_POINT('',(24.,12.,64.3));
#65177=CARTESIAN_POINT('Origin',(24.,12.,56.));
#65178=CARTESIAN_POINT('',(-6.,12.,64.3));
#65179=CARTESIAN_POINT('',(24.125,12.,64.3));
#65180=CARTESIAN_POINT('',(-9.70000000000001,12.,68.));
#65181=CARTESIAN_POINT('Origin',(-5.99999999999999,12.,68.));
#65182=CARTESIAN_POINT('',(-9.7,12.,88.));
#65183=CARTESIAN_POINT('',(-9.7,12.,64.75));
#65184=CARTESIAN_POINT('Origin',(-5.99999999999999,12.,88.));
#65185=CARTESIAN_POINT('',(-6.,12.,91.7));
#65186=CARTESIAN_POINT('Origin',(-5.99999999999999,12.,88.));
#65187=CARTESIAN_POINT('',(27.,12.,91.7));
#65188=CARTESIAN_POINT('',(9.125,12.,91.7));
#65189=CARTESIAN_POINT('',(32.3,12.,97.));
#65190=CARTESIAN_POINT('Origin',(27.,12.,97.));
#65191=CARTESIAN_POINT('',(32.3,12.,79.25));
#65192=CARTESIAN_POINT('',(-0.990000000000002,12.,78.));
#65193=CARTESIAN_POINT('Origin',(9.31,12.,78.));
#65194=CARTESIAN_POINT('Origin',(-5.99999999999999,11.85,88.));
#65195=CARTESIAN_POINT('',(-10.,11.7,88.));
#65196=CARTESIAN_POINT('',(-9.87296247153813,11.7000202118089,88.9999999999986));
#65197=CARTESIAN_POINT('Ctrl Pts',(-10.,11.7,88.));
#65198=CARTESIAN_POINT('Ctrl Pts',(-9.99999418587805,11.700005814122,88.2511225307642));
#65199=CARTESIAN_POINT('Ctrl Pts',(-9.97595940826116,11.700011270506,88.5108224697674));
#65200=CARTESIAN_POINT('Ctrl Pts',(-9.91022279769886,11.7000175155328,88.8462858496168));
#65201=CARTESIAN_POINT('Ctrl Pts',(-9.89276050036787,11.7000188950011,88.9233282445336));
#65202=CARTESIAN_POINT('Ctrl Pts',(-9.87296247153813,11.7000202118089,88.9999999999972));
#65203=CARTESIAN_POINT('Ctrl Pts',(-9.8729624715378,11.7000202118089,88.9999999999985));
#65204=CARTESIAN_POINT('Ctrl Pts',(-9.86888099751967,11.7000204832762,89.0158063098357));
#65205=CARTESIAN_POINT('Ctrl Pts',(-9.8647001926743,11.7000207520947,89.0315975460681));
#65206=CARTESIAN_POINT('Ctrl Pts',(-9.86042062850558,11.7000210181973,89.0473702429761));
#65207=CARTESIAN_POINT('Origin',(-5.9999073877354,0.,87.9999073877354));
#65208=CARTESIAN_POINT('Origin',(-5.9999073877354,12.,87.9999073877354));
#65209=CARTESIAN_POINT('Origin',(18.5190608795662,12.,105.));
#65210=CARTESIAN_POINT('Origin',(-5.9999073877354,0.,87.9999073877354));
#65211=CARTESIAN_POINT('',(-6.,-4.72,92.));
#65212=CARTESIAN_POINT('',(-6.,0.,92.));
#65213=CARTESIAN_POINT('Origin',(-5.9999073877354,-0.71990738773516,87.9999073877354));
#65214=CARTESIAN_POINT('Origin',(-5.9999073877354,0.,87.9999073877354));
#65215=CARTESIAN_POINT('',(-6.,4.72,92.));
#65216=CARTESIAN_POINT('Origin',(-5.9999073877354,0.71990738773516,87.9999073877354));
#65217=CARTESIAN_POINT('',(-6.,0.,92.));
#65218=CARTESIAN_POINT('Origin',(25.,-12.025,73.));
#65219=CARTESIAN_POINT('',(56.4658830061617,-12.025,11.5396446609407));
#65220=CARTESIAN_POINT('',(24.53125,-12.025,11.5396446609407));
#65221=CARTESIAN_POINT('',(56.7593104814471,-12.025,11.275));
#65222=CARTESIAN_POINT('Origin',(58.5,-12.025,13.5));
#65223=CARTESIAN_POINT('',(57.3600986884822,-12.025,11.275));
#65224=CARTESIAN_POINT('',(24.4375,-12.025,11.275));
#65225=CARTESIAN_POINT('Origin',(58.5,-12.025,13.5));
#65226=CARTESIAN_POINT('Origin',(25.,12.025,73.));
#65227=CARTESIAN_POINT('',(56.4658830061617,12.025,11.5396446609407));
#65228=CARTESIAN_POINT('',(24.53125,12.025,11.5396446609407));
#65229=CARTESIAN_POINT('',(57.3600986884822,12.025,11.275));
#65230=CARTESIAN_POINT('Origin',(58.5,12.025,13.5));
#65231=CARTESIAN_POINT('',(56.7593104814471,12.025,11.275));
#65232=CARTESIAN_POINT('',(24.4375,12.025,11.275));
#65233=CARTESIAN_POINT('Origin',(58.5,12.025,13.5));
#65234=CARTESIAN_POINT('Origin',(25.,12.025,73.));
#65235=CARTESIAN_POINT('Origin',(24.,12.025,19.));
#65236=CARTESIAN_POINT('Origin',(25.,-12.025,73.));
#65237=CARTESIAN_POINT('Origin',(24.,-12.025,19.));
#65238=CARTESIAN_POINT('Origin',(24.,0.,19.));
#65239=CARTESIAN_POINT('Origin',(24.,-4.29999999999991,19.));
#65240=CARTESIAN_POINT('Origin',(24.,0.,19.));
#65241=CARTESIAN_POINT('',(26.1702534414211,12.,11.3));
#65242=CARTESIAN_POINT('Origin',(24.,12.,19.));
#65243=CARTESIAN_POINT('Origin',(24.,4.29999999999991,19.));
#65244=CARTESIAN_POINT('Origin',(14.26,4.62,64.1));
#65245=CARTESIAN_POINT('',(4.72,4.72,64.));
#65246=CARTESIAN_POINT('',(14.26,4.72,64.));
#65247=CARTESIAN_POINT('',(4.72,4.72,64.));
#65248=CARTESIAN_POINT('Origin',(-5.99999999999999,11.85,68.));
#65249=CARTESIAN_POINT('',(-10.,11.7,68.));
#65250=CARTESIAN_POINT('',(-6.,11.7,64.));
#65251=CARTESIAN_POINT('Origin',(58.5,-11.85,13.5));
#65252=CARTESIAN_POINT('',(56.6959605211562,-12.212132034356,11.087867965644));
#65253=CARTESIAN_POINT('Origin',(58.5,-11.6298989873223,12.4935028842544));
#65254=CARTESIAN_POINT('Ctrl Pts',(56.7593104814471,-12.025,11.275));
#65255=CARTESIAN_POINT('Ctrl Pts',(56.7276355013012,-12.116893843234,11.183106156766));
#65256=CARTESIAN_POINT('Ctrl Pts',(56.6959605211562,-12.212132034356,11.087867965644));
#65257=CARTESIAN_POINT('Origin',(58.5,-11.85,13.5));
#65258=CARTESIAN_POINT('Origin',(24.0625,12.106066017178,11.343933982822));
#65259=CARTESIAN_POINT('',(56.6959605211562,12.212132034356,11.087867965644));
#65260=CARTESIAN_POINT('Origin',(58.5,11.6298989873223,12.4935028842544));
#65261=CARTESIAN_POINT('',(27.1391971013664,12.212132034356,11.087867965644));
#65262=CARTESIAN_POINT('',(24.0625,12.212132034356,11.087867965644));
#65263=CARTESIAN_POINT('Origin',(24.,10.0189862838483,16.3825901807804));
#65264=CARTESIAN_POINT('Origin',(58.5,0.,13.5));
#65265=CARTESIAN_POINT('Origin',(58.5,9.79999999999997,13.5));
#65266=CARTESIAN_POINT('Origin',(58.5,11.85,13.5));
#65267=CARTESIAN_POINT('Ctrl Pts',(56.6959605211562,12.212132034356,11.087867965644));
#65268=CARTESIAN_POINT('Ctrl Pts',(56.7276355013016,12.1168938432326,11.1831061567674));
#65269=CARTESIAN_POINT('Ctrl Pts',(56.7593104814471,12.025,11.275));
#65270=CARTESIAN_POINT('Origin',(18.,0.,64.));
#65271=CARTESIAN_POINT('',(24.,-11.7,64.));
#65272=CARTESIAN_POINT('',(24.,0.,64.));
#65273=CARTESIAN_POINT('',(24.125,-11.7,64.));
#65274=CARTESIAN_POINT('Origin',(18.,0.,64.));
#65275=CARTESIAN_POINT('',(24.,11.7,64.));
#65276=CARTESIAN_POINT('',(24.125,11.7,64.));
#65277=CARTESIAN_POINT('',(24.,12.,64.));
#65278=CARTESIAN_POINT('',(24.,0.,64.));
#65279=CARTESIAN_POINT('',(24.,12.,64.));
#65280=CARTESIAN_POINT('Origin',(24.0004975859988,0.,56.0004975859988));
#65281=CARTESIAN_POINT('Ctrl Pts',(24.,-11.7,64.));
#65282=CARTESIAN_POINT('Ctrl Pts',(24.5022176904815,-11.7000312390044,64.0000312390044));
#65283=CARTESIAN_POINT('Ctrl Pts',(25.0215928562724,-11.7000605560293,63.9520071546108));
#65284=CARTESIAN_POINT('Ctrl Pts',(26.0547668862757,-11.7001122298415,63.749634158072));
#65285=CARTESIAN_POINT('Ctrl Pts',(26.5685742270846,-11.7001345898519,63.5953285238635));
#65286=CARTESIAN_POINT('Ctrl Pts',(27.5540556052171,-11.7001704995408,63.1872005862129));
#65287=CARTESIAN_POINT('Ctrl Pts',(28.0265144414246,-11.7001840778188,62.9330532656189));
#65288=CARTESIAN_POINT('Ctrl Pts',(28.9002511996986,-11.7002018897492,62.345696912753));
#65289=CARTESIAN_POINT('Ctrl Pts',(29.3015045180536,-11.7002061195955,62.0124512814371));
#65290=CARTESIAN_POINT('Ctrl Pts',(30.0117917671937,-11.700206125091,61.3022523895444));
#65291=CARTESIAN_POINT('Ctrl Pts',(30.3450873135436,-11.7002019009279,60.901040531463));
#65292=CARTESIAN_POINT('Ctrl Pts',(30.9325523584188,-11.7001841003031,60.0273768495693));
#65293=CARTESIAN_POINT('Ctrl Pts',(31.1867584529271,-11.7001705276473,59.5549496340214));
#65294=CARTESIAN_POINT('Ctrl Pts',(31.5950089854782,-11.700134628742,58.5695190363596));
#65295=CARTESIAN_POINT('Ctrl Pts',(31.7493785383029,-11.7001122739014,58.0557308958014));
#65296=CARTESIAN_POINT('Ctrl Pts',(31.9518800645024,-11.7000606096502,57.0225820498513));
#65297=CARTESIAN_POINT('Ctrl Pts',(31.9999687609956,-11.7000312970161,56.5032128624791));
#65298=CARTESIAN_POINT('Ctrl Pts',(32.0000000206335,-11.7000000412671,56.0006634554817));
#65299=CARTESIAN_POINT('Ctrl Pts',(32.0000000206344,-11.7000000206344,56.0003317314806));
#65300=CARTESIAN_POINT('Ctrl Pts',(32.,-11.7,56.));
#65301=CARTESIAN_POINT('Origin',(24.0004975859988,0.,56.0004975859988));
#65302=CARTESIAN_POINT('Ctrl Pts',(32.,11.7,56.));
#65303=CARTESIAN_POINT('Ctrl Pts',(32.000031241594,11.700031241594,56.5022593219641));
#65304=CARTESIAN_POINT('Ctrl Pts',(31.9519992003628,11.7000605607168,57.0216761760518));
#65305=CARTESIAN_POINT('Ctrl Pts',(31.7495941438916,11.7001122374015,58.0549284493937));
#65306=CARTESIAN_POINT('Ctrl Pts',(31.5952644237359,11.7001345981877,58.5687723493041));
#65307=CARTESIAN_POINT('Ctrl Pts',(31.1870742898692,11.700170507956,59.5543172013999));
#65308=CARTESIAN_POINT('Ctrl Pts',(30.9328887646418,11.7001840855418,60.0268031112652));
#65309=CARTESIAN_POINT('Ctrl Pts',(30.3454454128867,11.7002018946398,60.9005813312616));
#65310=CARTESIAN_POINT('Ctrl Pts',(30.0121509738491,11.7002061223446,61.3018490261509));
#65311=CARTESIAN_POINT('Ctrl Pts',(29.3018490261509,11.7002061223446,62.0121509738491));
#65312=CARTESIAN_POINT('Ctrl Pts',(28.9005813312616,11.7002018946398,62.3454454128867));
#65313=CARTESIAN_POINT('Ctrl Pts',(28.0268031112652,11.7001840855418,62.9328887646418));
#65314=CARTESIAN_POINT('Ctrl Pts',(27.5543172013999,11.700170507956,63.1870742898692));
#65315=CARTESIAN_POINT('Ctrl Pts',(26.5687723493041,11.7001345981878,63.5952644237359));
#65316=CARTESIAN_POINT('Ctrl Pts',(26.0549284493937,11.7001122374015,63.7495941438916));
#65317=CARTESIAN_POINT('Ctrl Pts',(25.0216761760518,11.7000605607168,63.9519992003628));
#65318=CARTESIAN_POINT('Ctrl Pts',(24.5022593219641,11.700031241594,64.000031241594));
#65319=CARTESIAN_POINT('Ctrl Pts',(24.,11.7,64.));
#65320=CARTESIAN_POINT('Origin',(24.0004975859988,12.,56.0004975859988));
#65321=CARTESIAN_POINT('Origin',(25.0000000077377,12.,55.5637382272397));
#65322=CARTESIAN_POINT('Origin',(24.,0.,64.));
#65323=CARTESIAN_POINT('',(24.125,-11.7,64.));
#65324=CARTESIAN_POINT('',(4.72,-4.72,64.));
#65325=CARTESIAN_POINT('',(8.95,-4.72,64.));
#65326=CARTESIAN_POINT('',(4.72,-2.26,64.));
#65327=CARTESIAN_POINT('',(24.125,11.7,64.));
#65328=CARTESIAN_POINT('Origin',(24.,-11.85,56.));
#65329=CARTESIAN_POINT('',(32.,-11.7,56.));
#65330=CARTESIAN_POINT('',(24.,-11.7,64.));
#65331=CARTESIAN_POINT('Origin',(44.,0.,100.));
#65332=CARTESIAN_POINT('',(32.,-12.,100.));
#65333=CARTESIAN_POINT('Origin',(44.,-12.,100.));
#65334=CARTESIAN_POINT('',(32.,-11.7,100.));
#65335=CARTESIAN_POINT('',(32.,0.,100.));
#65336=CARTESIAN_POINT('Origin',(44.,-11.7,100.));
#65337=CARTESIAN_POINT('Origin',(32.,0.,100.));
#65338=CARTESIAN_POINT('',(32.,-11.7,97.));
#65339=CARTESIAN_POINT('',(32.,-11.7,79.25));
#65340=CARTESIAN_POINT('',(32.,-12.,97.));
#65341=CARTESIAN_POINT('',(32.,-12.,97.));
#65342=CARTESIAN_POINT('',(32.,0.,97.));
#65343=CARTESIAN_POINT('Origin',(32.,0.,100.));
#65344=CARTESIAN_POINT('',(32.,11.7,97.));
#65345=CARTESIAN_POINT('',(32.,11.7,79.25));
#65346=CARTESIAN_POINT('',(32.,12.,97.));
#65347=CARTESIAN_POINT('',(32.,0.,97.));
#65348=CARTESIAN_POINT('',(32.,12.,97.));
#65349=CARTESIAN_POINT('Origin',(27.,0.,92.));
#65350=CARTESIAN_POINT('',(4.72,4.72,92.));
#65351=CARTESIAN_POINT('',(-0.74,4.72,92.));
#65352=CARTESIAN_POINT('',(4.72,-4.72,92.));
#65353=CARTESIAN_POINT('',(4.72,-2.26,92.));
#65354=CARTESIAN_POINT('',(-6.05,-4.72,92.));
#65355=CARTESIAN_POINT('Origin',(27.,0.,92.));
#65356=CARTESIAN_POINT('',(27.,-11.7,92.));
#65357=CARTESIAN_POINT('',(9.125,-11.7,92.));
#65358=CARTESIAN_POINT('',(27.,-12.,92.));
#65359=CARTESIAN_POINT('',(27.,0.,92.));
#65360=CARTESIAN_POINT('',(-6.,-12.,92.));
#65361=CARTESIAN_POINT('',(-6.,-12.,92.));
#65362=CARTESIAN_POINT('',(-6.,0.,92.));
#65363=CARTESIAN_POINT('Origin',(27.,0.,92.));
#65364=CARTESIAN_POINT('',(-6.,11.7,92.));
#65365=CARTESIAN_POINT('',(27.,11.7,92.));
#65366=CARTESIAN_POINT('',(9.125,11.7,92.));
#65367=CARTESIAN_POINT('',(-6.,12.,92.));
#65368=CARTESIAN_POINT('',(-6.,0.,92.));
#65369=CARTESIAN_POINT('',(27.,12.,92.));
#65370=CARTESIAN_POINT('',(-6.,12.,92.));
#65371=CARTESIAN_POINT('',(27.,0.,92.));
#65372=CARTESIAN_POINT('Origin',(-5.9999073877354,0.,87.9999073877354));
#65373=CARTESIAN_POINT('Origin',(-5.9999073877354,-12.,87.9999073877354));
#65374=CARTESIAN_POINT('Origin',(18.5190608795662,-12.,105.));
#65375=CARTESIAN_POINT('Origin',(26.9998842346692,-12.,97.0001157653307));
#65376=CARTESIAN_POINT('Origin',(-5.9999073877354,0.,87.9999073877354));
#65377=CARTESIAN_POINT('Origin',(-5.9999073877354,12.,87.9999073877354));
#65378=CARTESIAN_POINT('Ctrl Pts',(-8.42436827442023,11.7000371816705,91.1815312379424));
#65379=CARTESIAN_POINT('Ctrl Pts',(-8.36188086740803,11.7000368373637,91.2291478894839));
#65380=CARTESIAN_POINT('Ctrl Pts',(-8.29762358003265,11.7000364158445,91.2751995818108));
#65381=CARTESIAN_POINT('Ctrl Pts',(-8.013329790593,11.7000342590358,91.4663398648887));
#65382=CARTESIAN_POINT('Ctrl Pts',(-7.77709609606059,11.7000317321777,91.5934374252052));
#65383=CARTESIAN_POINT('Ctrl Pts',(-7.28434258369623,11.7000250491913,91.7975492958902));
#65384=CARTESIAN_POINT('Ctrl Pts',(-7.02743037635763,11.7000208877413,91.8747261446359));
#65385=CARTESIAN_POINT('Ctrl Pts',(-6.51082246976743,11.700011270506,91.9759594082611));
#65386=CARTESIAN_POINT('Ctrl Pts',(-6.25112253076428,11.700005814122,91.999994185878));
#65387=CARTESIAN_POINT('Ctrl Pts',(-5.99999999999999,11.7,92.));
#65388=CARTESIAN_POINT('Origin',(26.9998842346692,0.,97.0001157653307));
#65389=CARTESIAN_POINT('',(27.,0.,92.));
#65390=CARTESIAN_POINT('Origin',(26.9998842346692,12.,97.0001157653307));
#65391=CARTESIAN_POINT('',(32.,0.,97.));
#65392=CARTESIAN_POINT('Origin',(18.5190608795662,12.,105.));
#65393=CARTESIAN_POINT('Origin',(-5.99999999999999,11.85,88.));
#65394=CARTESIAN_POINT('',(-6.,11.7,92.));
#65395=CARTESIAN_POINT('Origin',(-0.74,4.62,91.9));
#65396=CARTESIAN_POINT('',(4.52,4.52,91.8));
#65397=CARTESIAN_POINT('Origin',(32.,0.,27.4736520332184));
#65398=CARTESIAN_POINT('',(32.,-11.7,19.));
#65399=CARTESIAN_POINT('',(32.,0.,19.));
#65400=CARTESIAN_POINT('',(32.,-11.7,40.25));
#65401=CARTESIAN_POINT('Origin',(32.,0.,27.4736520332184));
#65402=CARTESIAN_POINT('',(32.,11.7,19.));
#65403=CARTESIAN_POINT('',(32.,11.7,40.25));
#65404=CARTESIAN_POINT('',(32.,12.,19.));
#65405=CARTESIAN_POINT('',(32.,0.,19.));
#65406=CARTESIAN_POINT('',(32.,12.,19.));
#65407=CARTESIAN_POINT('Origin',(24.0004975859988,0.,18.9995024140012));
#65408=CARTESIAN_POINT('',(27.0397667852433,-11.7001517572237,11.5998482427763));
#65409=CARTESIAN_POINT('Origin',(24.0004975859988,-4.3004975859987,18.9995024140012));
#65410=CARTESIAN_POINT('Ctrl Pts',(32.,-11.7,19.));
#65411=CARTESIAN_POINT('Ctrl Pts',(32.0000312390044,-11.7000312390044,18.4977823095185));
#65412=CARTESIAN_POINT('Ctrl Pts',(31.9520071546108,-11.7000605560293,17.9784071437276));
#65413=CARTESIAN_POINT('Ctrl Pts',(31.749634158072,-11.7001122298415,16.9452331137243));
#65414=CARTESIAN_POINT('Ctrl Pts',(31.5953285238635,-11.7001345898519,16.4314257729154));
#65415=CARTESIAN_POINT('Ctrl Pts',(31.1872005862129,-11.7001704995408,15.4459443947829));
#65416=CARTESIAN_POINT('Ctrl Pts',(30.9330532656189,-11.7001840778189,14.9734855585754));
#65417=CARTESIAN_POINT('Ctrl Pts',(30.345696912753,-11.7002018897492,14.0997488003014));
#65418=CARTESIAN_POINT('Ctrl Pts',(30.0124512814371,-11.7002061195955,13.6984954819464));
#65419=CARTESIAN_POINT('Ctrl Pts',(29.3022523895444,-11.700206125091,12.9882082328063));
#65420=CARTESIAN_POINT('Ctrl Pts',(28.901040531463,-11.7002019009279,12.6549126864564));
#65421=CARTESIAN_POINT('Ctrl Pts',(28.0273768495693,-11.7001841003031,12.0674476415812));
#65422=CARTESIAN_POINT('Ctrl Pts',(27.5549496340214,-11.7001705276473,11.8132415470729));
#65423=CARTESIAN_POINT('Ctrl Pts',(27.0547499335288,-11.7001523055404,11.6060155946897));
#65424=CARTESIAN_POINT('Ctrl Pts',(27.0472607306568,-11.7001520318827,11.6029262403352));
#65425=CARTESIAN_POINT('Ctrl Pts',(27.0397667852433,-11.7001517572237,11.5998482427763));
#65426=CARTESIAN_POINT('Origin',(24.0004975859988,0.,18.9995024140012));
#65427=CARTESIAN_POINT('',(26.1706823007161,12.,11.3));
#65428=CARTESIAN_POINT('',(27.0397667852433,11.7001517572237,11.5998482427763));
#65429=CARTESIAN_POINT('Origin',(24.0004975859988,4.3004975859987,18.9995024140012));
#65430=CARTESIAN_POINT('Origin',(24.0004975859988,12.,18.9995024140012));
#65431=CARTESIAN_POINT('Ctrl Pts',(27.0397667852433,11.7001517572237,11.5998482427763));
#65432=CARTESIAN_POINT('Ctrl Pts',(27.0470305895134,11.7001520234479,11.602831714176));
#65433=CARTESIAN_POINT('Ctrl Pts',(27.0542899373568,11.7001522887312,11.6058258552508));
#65434=CARTESIAN_POINT('Ctrl Pts',(27.5543172013999,11.700170507956,11.8129257101308));
#65435=CARTESIAN_POINT('Ctrl Pts',(28.0268031112652,11.7001840855418,12.0671112353582));
#65436=CARTESIAN_POINT('Ctrl Pts',(28.9005813312616,11.7002018946398,12.6545545871133));
#65437=CARTESIAN_POINT('Ctrl Pts',(29.3018490261509,11.7002061223446,12.9878490261509));
#65438=CARTESIAN_POINT('Ctrl Pts',(30.0121509738491,11.7002061223446,13.6981509738491));
#65439=CARTESIAN_POINT('Ctrl Pts',(30.3454454128867,11.7002018946398,14.0994186687384));
#65440=CARTESIAN_POINT('Ctrl Pts',(30.9328887646418,11.7001840855418,14.9731968887348));
#65441=CARTESIAN_POINT('Ctrl Pts',(31.1870742898692,11.700170507956,15.4456827986001));
#65442=CARTESIAN_POINT('Ctrl Pts',(31.5952644237359,11.7001345981877,16.4312276506959));
#65443=CARTESIAN_POINT('Ctrl Pts',(31.7495941438916,11.7001122374015,16.9450715506063));
#65444=CARTESIAN_POINT('Ctrl Pts',(31.9519992003628,11.7000605607168,17.9783238239482));
#65445=CARTESIAN_POINT('Ctrl Pts',(32.000031241594,11.700031241594,18.4977406780359));
#65446=CARTESIAN_POINT('Ctrl Pts',(32.,11.7,19.));
#65447=CARTESIAN_POINT('Origin',(2.98958333333334,0.,37.3005642361111));
#65448=CARTESIAN_POINT('',(32.,0.,27.4736520332184));
#65449=CARTESIAN_POINT('Origin',(28.5000000077377,12.,19.2681696700813));
#65450=CARTESIAN_POINT('',(26.1875000038689,12.,11.3));
#65451=CARTESIAN_POINT('Origin',(23.875,12.15,11.15));
#65452=CARTESIAN_POINT('',(27.0983866769659,12.,11.3));
#65453=CARTESIAN_POINT('Ctrl Pts',(27.0397667852433,11.7001517572237,11.5998482427763));
#65454=CARTESIAN_POINT('Ctrl Pts',(27.0690767311041,11.8486440903987,11.4513559096013));
#65455=CARTESIAN_POINT('Ctrl Pts',(27.0983866769659,12.,11.3));
#65456=CARTESIAN_POINT('Ctrl Pts',(27.0983866769659,12.,11.3));
#65457=CARTESIAN_POINT('Ctrl Pts',(27.1187918891661,12.1053720627028,11.1946279372972));
#65458=CARTESIAN_POINT('Ctrl Pts',(27.1391971013664,12.212132034356,11.087867965644));
#65459=CARTESIAN_POINT('Origin',(24.,11.85,19.));
#65460=CARTESIAN_POINT('',(32.,11.7,19.));
#65461=CARTESIAN_POINT('Origin',(32.,0.,19.));
#65462=CARTESIAN_POINT('',(32.,11.7,40.25));
#65463=CARTESIAN_POINT('',(32.,-11.7,40.25));
#65464=CARTESIAN_POINT('Origin',(54.3509571552277,-12.,80.3999996185303));
#65465=CARTESIAN_POINT('',(54.3509571552277,-12.4,86.7057294845581));
#65466=CARTESIAN_POINT('',(54.3509571552277,-12.,86.7057294845581));
#65467=CARTESIAN_POINT('',(54.3509571552277,-12.4,80.3999996185303));
#65468=CARTESIAN_POINT('',(54.3509571552277,-12.4,86.7057294845581));
#65469=CARTESIAN_POINT('',(54.3509571552277,-12.,80.3999996185303));
#65470=CARTESIAN_POINT('Origin',(52.6085274219513,-12.,80.3999996185303));
#65471=CARTESIAN_POINT('',(52.6085274219513,-12.4,80.3999996185303));
#65472=CARTESIAN_POINT('',(54.3509571552277,-12.4,80.3999996185303));
#65473=CARTESIAN_POINT('',(52.6085274219513,-12.,80.3999996185303));
#65474=CARTESIAN_POINT('Origin',(52.6085274219513,-12.,84.5319232940674));
#65475=CARTESIAN_POINT('',(52.6085274219513,-12.4,84.5319232940674));
#65476=CARTESIAN_POINT('',(52.6085274219513,-12.4,80.3999996185303));
#65477=CARTESIAN_POINT('',(52.6085274219513,-12.,84.5319232940674));
#65478=CARTESIAN_POINT('Ctrl Pts',(51.7901794910431,-12.,84.0117321014404));
#65479=CARTESIAN_POINT('Ctrl Pts',(51.7901794910431,-12.4,84.0117321014404));
#65480=CARTESIAN_POINT('Ctrl Pts',(52.1856091022491,-12.,84.2105045318604));
#65481=CARTESIAN_POINT('Ctrl Pts',(52.1856091022491,-12.4,84.2105045318604));
#65482=CARTESIAN_POINT('Ctrl Pts',(52.6085274219513,-12.,84.5319232940674));
#65483=CARTESIAN_POINT('Ctrl Pts',(52.6085274219513,-12.4,84.5319232940674));
#65484=CARTESIAN_POINT('',(51.7901794910431,-12.4,84.0117321014404));
#65485=CARTESIAN_POINT('Ctrl Pts',(51.7901794910431,-12.4,84.0117321014404));
#65486=CARTESIAN_POINT('Ctrl Pts',(52.1856091022491,-12.4,84.2105045318604));
#65487=CARTESIAN_POINT('Ctrl Pts',(52.6085274219513,-12.4,84.5319232940674));
#65488=CARTESIAN_POINT('',(51.7901794910431,-12.,84.0117321014404));
#65489=CARTESIAN_POINT('Ctrl Pts',(50.7984325885773,-12.,83.6311044692993));
#65490=CARTESIAN_POINT('Ctrl Pts',(50.7984325885773,-12.4,83.6311044692993));
#65491=CARTESIAN_POINT('Ctrl Pts',(51.394749879837,-12.,83.8129596710205));
#65492=CARTESIAN_POINT('Ctrl Pts',(51.394749879837,-12.4,83.8129596710205));
#65493=CARTESIAN_POINT('Ctrl Pts',(51.7901794910431,-12.,84.0117321014404));
#65494=CARTESIAN_POINT('Ctrl Pts',(51.7901794910431,-12.4,84.0117321014404));
#65495=CARTESIAN_POINT('',(50.7984325885773,-12.4,83.6311044692993));
#65496=CARTESIAN_POINT('Ctrl Pts',(50.7984325885773,-12.4,83.6311044692993));
#65497=CARTESIAN_POINT('Ctrl Pts',(51.394749879837,-12.4,83.8129596710205));
#65498=CARTESIAN_POINT('Ctrl Pts',(51.7901794910431,-12.4,84.0117321014404));
#65499=CARTESIAN_POINT('',(50.7984325885773,-12.,83.6311044692993));
#65500=CARTESIAN_POINT('Origin',(50.7984325885773,-12.,85.0436553955078));
#65501=CARTESIAN_POINT('',(50.7984325885773,-12.4,85.0436553955078));
#65502=CARTESIAN_POINT('',(50.7984325885773,-12.4,83.6311044692993));
#65503=CARTESIAN_POINT('',(50.7984325885773,-12.,85.0436553955078));
#65504=CARTESIAN_POINT('Ctrl Pts',(52.1644623279572,-12.,85.7245559692383));
#65505=CARTESIAN_POINT('Ctrl Pts',(52.1644623279572,-12.4,85.7245559692383));
#65506=CARTESIAN_POINT('Ctrl Pts',(51.6781055927277,-12.,85.3270111083984));
#65507=CARTESIAN_POINT('Ctrl Pts',(51.6781055927277,-12.4,85.3270111083984));
#65508=CARTESIAN_POINT('Ctrl Pts',(50.7984325885773,-12.,85.0436553955078));
#65509=CARTESIAN_POINT('Ctrl Pts',(50.7984325885773,-12.4,85.0436553955078));
#65510=CARTESIAN_POINT('',(52.1644623279572,-12.4,85.7245559692383));
#65511=CARTESIAN_POINT('Ctrl Pts',(52.1644623279572,-12.4,85.7245559692383));
#65512=CARTESIAN_POINT('Ctrl Pts',(51.6781055927277,-12.4,85.3270111083984));
#65513=CARTESIAN_POINT('Ctrl Pts',(50.7984325885773,-12.4,85.0436553955078));
#65514=CARTESIAN_POINT('',(52.1644623279572,-12.,85.7245559692383));
#65515=CARTESIAN_POINT('Ctrl Pts',(52.9257175922394,-12.,86.7057294845581));
#65516=CARTESIAN_POINT('Ctrl Pts',(52.9257175922394,-12.4,86.7057294845581));
#65517=CARTESIAN_POINT('Ctrl Pts',(52.6508209705353,-12.,86.122100353241));
#65518=CARTESIAN_POINT('Ctrl Pts',(52.6508209705353,-12.4,86.122100353241));
#65519=CARTESIAN_POINT('Ctrl Pts',(52.1644623279572,-12.,85.7245559692383));
#65520=CARTESIAN_POINT('Ctrl Pts',(52.1644623279572,-12.4,85.7245559692383));
#65521=CARTESIAN_POINT('',(52.9257175922394,-12.4,86.7057294845581));
#65522=CARTESIAN_POINT('Ctrl Pts',(52.9257175922394,-12.4,86.7057294845581));
#65523=CARTESIAN_POINT('Ctrl Pts',(52.6508209705353,-12.4,86.122100353241));
#65524=CARTESIAN_POINT('Ctrl Pts',(52.1644623279572,-12.4,85.7245559692383));
#65525=CARTESIAN_POINT('',(52.9257175922394,-12.,86.7057294845581));
#65526=CARTESIAN_POINT('Origin',(54.3509571552277,-12.,86.7057294845581));
#65527=CARTESIAN_POINT('',(52.9257175922394,-12.4,86.7057294845581));
#65528=CARTESIAN_POINT('Origin',(52.5746948719025,-12.4,83.5528645515442));
#65529=CARTESIAN_POINT('Origin',(35.4379951953888,-12.,86.5999994277954));
#65530=CARTESIAN_POINT('',(33.6490461826324,-12.4,86.5999994277954));
#65531=CARTESIAN_POINT('',(33.6490461826324,-12.,86.5999994277954));
#65532=CARTESIAN_POINT('',(35.4379951953888,-12.4,86.5999994277954));
#65533=CARTESIAN_POINT('',(33.6490461826324,-12.4,86.5999994277954));
#65534=CARTESIAN_POINT('',(35.4379951953888,-12.,86.5999994277954));
#65535=CARTESIAN_POINT('Origin',(37.772510766983,-12.,83.1698579788208));
#65536=CARTESIAN_POINT('',(37.772510766983,-12.4,83.1698579788208));
#65537=CARTESIAN_POINT('',(35.4379951953888,-12.4,86.5999994277954));
#65538=CARTESIAN_POINT('',(37.772510766983,-12.,83.1698579788208));
#65539=CARTESIAN_POINT('Origin',(37.772510766983,-12.,86.5999994277954));
#65540=CARTESIAN_POINT('',(37.772510766983,-12.4,86.5999994277954));
#65541=CARTESIAN_POINT('',(37.772510766983,-12.4,83.1698579788208));
#65542=CARTESIAN_POINT('',(37.772510766983,-12.,86.5999994277954));
#65543=CARTESIAN_POINT('Origin',(39.5783770084381,-12.,86.5999994277954));
#65544=CARTESIAN_POINT('',(39.5783770084381,-12.4,86.5999994277954));
#65545=CARTESIAN_POINT('',(37.772510766983,-12.4,86.5999994277954));
#65546=CARTESIAN_POINT('',(39.5783770084381,-12.,86.5999994277954));
#65547=CARTESIAN_POINT('Origin',(39.5783770084381,-12.,80.3999996185303));
#65548=CARTESIAN_POINT('',(39.5783770084381,-12.4,80.3999996185303));
#65549=CARTESIAN_POINT('',(39.5783770084381,-12.4,86.5999994277954));
#65550=CARTESIAN_POINT('',(39.5783770084381,-12.,80.3999996185303));
#65551=CARTESIAN_POINT('Origin',(37.772510766983,-12.,80.3999996185303));
#65552=CARTESIAN_POINT('',(37.772510766983,-12.4,80.3999996185303));
#65553=CARTESIAN_POINT('',(39.5783770084381,-12.4,80.3999996185303));
#65554=CARTESIAN_POINT('',(37.772510766983,-12.,80.3999996185303));
#65555=CARTESIAN_POINT('Origin',(35.4506828784943,-12.,83.8042373657227));
#65556=CARTESIAN_POINT('',(35.4506828784943,-12.4,83.8042373657227));
#65557=CARTESIAN_POINT('',(37.772510766983,-12.4,80.3999996185303));
#65558=CARTESIAN_POINT('',(35.4506828784943,-12.,83.8042373657227));
#65559=CARTESIAN_POINT('Origin',(35.4506828784943,-12.,80.3999996185303));
#65560=CARTESIAN_POINT('',(35.4506828784943,-12.4,80.3999996185303));
#65561=CARTESIAN_POINT('',(35.4506828784943,-12.4,83.8042373657227));
#65562=CARTESIAN_POINT('',(35.4506828784943,-12.,80.3999996185303));
#65563=CARTESIAN_POINT('Origin',(33.6490461826324,-12.,80.3999996185303));
#65564=CARTESIAN_POINT('',(33.6490461826324,-12.4,80.3999996185303));
#65565=CARTESIAN_POINT('',(35.4506828784943,-12.4,80.3999996185303));
#65566=CARTESIAN_POINT('',(33.6490461826324,-12.,80.3999996185303));
#65567=CARTESIAN_POINT('Origin',(33.6490461826324,-12.,86.5999994277954));
#65568=CARTESIAN_POINT('',(33.6490461826324,-12.4,80.3999996185303));
#65569=CARTESIAN_POINT('Origin',(36.6137115955353,-12.4,83.4999995231628));
#65570=CARTESIAN_POINT('Ctrl Pts',(42.5261261463165,-12.,83.4873123168945));
#65571=CARTESIAN_POINT('Ctrl Pts',(42.5261261463165,-12.4,83.4873123168945));
#65572=CARTESIAN_POINT('Ctrl Pts',(42.5261261463165,-12.,84.4346513748169));
#65573=CARTESIAN_POINT('Ctrl Pts',(42.5261261463165,-12.4,84.4346513748169));
#65574=CARTESIAN_POINT('Ctrl Pts',(42.8771488666534,-12.,84.8448829650879));
#65575=CARTESIAN_POINT('Ctrl Pts',(42.8771488666534,-12.4,84.8448829650879));
#65576=CARTESIAN_POINT('',(42.8771488666534,-12.,84.8448829650879));
#65577=CARTESIAN_POINT('',(42.5261261463165,-12.,83.4873123168945));
#65578=CARTESIAN_POINT('Ctrl Pts',(42.8771488666534,-12.,84.8448829650879));
#65579=CARTESIAN_POINT('Ctrl Pts',(42.5261261463165,-12.,84.4346513748169));
#65580=CARTESIAN_POINT('Ctrl Pts',(42.5261261463165,-12.,83.4873123168945));
#65581=CARTESIAN_POINT('',(42.8771488666534,-12.4,84.8448829650879));
#65582=CARTESIAN_POINT('',(42.8771488666534,-12.,84.8448829650879));
#65583=CARTESIAN_POINT('',(42.5261261463165,-12.4,83.4873123168945));
#65584=CARTESIAN_POINT('Ctrl Pts',(42.5261261463165,-12.4,83.4873123168945));
#65585=CARTESIAN_POINT('Ctrl Pts',(42.5261261463165,-12.4,84.4346513748169));
#65586=CARTESIAN_POINT('Ctrl Pts',(42.8771488666534,-12.4,84.8448829650879));
#65587=CARTESIAN_POINT('',(42.5261261463165,-12.,83.4873123168945));
#65588=CARTESIAN_POINT('Ctrl Pts',(42.875034570694,-12.,82.1381988525391));
#65589=CARTESIAN_POINT('Ctrl Pts',(42.875034570694,-12.4,82.1381988525391));
#65590=CARTESIAN_POINT('Ctrl Pts',(42.5261261463165,-12.,82.5484304428101));
#65591=CARTESIAN_POINT('Ctrl Pts',(42.5261261463165,-12.4,82.5484304428101));
#65592=CARTESIAN_POINT('Ctrl Pts',(42.5261261463165,-12.,83.4873123168945));
#65593=CARTESIAN_POINT('Ctrl Pts',(42.5261261463165,-12.4,83.4873123168945));
#65594=CARTESIAN_POINT('',(42.875034570694,-12.,82.1381988525391));
#65595=CARTESIAN_POINT('Ctrl Pts',(42.5261261463165,-12.,83.4873123168945));
#65596=CARTESIAN_POINT('Ctrl Pts',(42.5261261463165,-12.,82.5484304428101));
#65597=CARTESIAN_POINT('Ctrl Pts',(42.875034570694,-12.,82.1381988525391));
#65598=CARTESIAN_POINT('',(42.875034570694,-12.4,82.1381988525391));
#65599=CARTESIAN_POINT('Ctrl Pts',(42.875034570694,-12.4,82.1381988525391));
#65600=CARTESIAN_POINT('Ctrl Pts',(42.5261261463165,-12.4,82.5484304428101));
#65601=CARTESIAN_POINT('Ctrl Pts',(42.5261261463165,-12.4,83.4873123168945));
#65602=CARTESIAN_POINT('',(42.875034570694,-12.,82.1381988525391));
#65603=CARTESIAN_POINT('Ctrl Pts',(43.8244888782501,-12.,81.7279672622681));
#65604=CARTESIAN_POINT('Ctrl Pts',(43.8244888782501,-12.4,81.7279672622681));
#65605=CARTESIAN_POINT('Ctrl Pts',(43.2239429950714,-12.,81.7279672622681));
#65606=CARTESIAN_POINT('Ctrl Pts',(43.2239429950714,-12.4,81.7279672622681));
#65607=CARTESIAN_POINT('Ctrl Pts',(42.875034570694,-12.,82.1381988525391));
#65608=CARTESIAN_POINT('Ctrl Pts',(42.875034570694,-12.4,82.1381988525391));
#65609=CARTESIAN_POINT('',(43.8244888782501,-12.,81.7279672622681));
#65610=CARTESIAN_POINT('Ctrl Pts',(42.875034570694,-12.,82.1381988525391));
#65611=CARTESIAN_POINT('Ctrl Pts',(43.2239429950714,-12.,81.7279672622681));
#65612=CARTESIAN_POINT('Ctrl Pts',(43.8244888782501,-12.,81.7279672622681));
#65613=CARTESIAN_POINT('',(43.8244888782501,-12.4,81.7279672622681));
#65614=CARTESIAN_POINT('Ctrl Pts',(43.8244888782501,-12.4,81.7279672622681));
#65615=CARTESIAN_POINT('Ctrl Pts',(43.2239429950714,-12.4,81.7279672622681));
#65616=CARTESIAN_POINT('Ctrl Pts',(42.875034570694,-12.4,82.1381988525391));
#65617=CARTESIAN_POINT('',(43.8244888782501,-12.,81.7279672622681));
#65618=CARTESIAN_POINT('Ctrl Pts',(44.780287027359,-12.,82.1297407150269));
#65619=CARTESIAN_POINT('Ctrl Pts',(44.780287027359,-12.4,82.1297407150269));
#65620=CARTESIAN_POINT('Ctrl Pts',(44.4419510364532,-12.,81.7279672622681));
#65621=CARTESIAN_POINT('Ctrl Pts',(44.4419510364532,-12.4,81.7279672622681));
#65622=CARTESIAN_POINT('Ctrl Pts',(43.8244888782501,-12.,81.7279672622681));
#65623=CARTESIAN_POINT('Ctrl Pts',(43.8244888782501,-12.4,81.7279672622681));
#65624=CARTESIAN_POINT('',(44.780287027359,-12.,82.1297407150269));
#65625=CARTESIAN_POINT('Ctrl Pts',(43.8244888782501,-12.,81.7279672622681));
#65626=CARTESIAN_POINT('Ctrl Pts',(44.4419510364532,-12.,81.7279672622681));
#65627=CARTESIAN_POINT('Ctrl Pts',(44.780287027359,-12.,82.1297407150269));
#65628=CARTESIAN_POINT('',(44.780287027359,-12.4,82.1297407150269));
#65629=CARTESIAN_POINT('Ctrl Pts',(44.780287027359,-12.4,82.1297407150269));
#65630=CARTESIAN_POINT('Ctrl Pts',(44.4419510364532,-12.4,81.7279672622681));
#65631=CARTESIAN_POINT('Ctrl Pts',(43.8244888782501,-12.4,81.7279672622681));
#65632=CARTESIAN_POINT('',(44.780287027359,-12.,82.1297407150269));
#65633=CARTESIAN_POINT('Ctrl Pts',(45.1186230182648,-12.,83.5718955993652));
#65634=CARTESIAN_POINT('Ctrl Pts',(45.1186230182648,-12.4,83.5718955993652));
#65635=CARTESIAN_POINT('Ctrl Pts',(45.1186230182648,-12.,82.5315141677856));
#65636=CARTESIAN_POINT('Ctrl Pts',(45.1186230182648,-12.4,82.5315141677856));
#65637=CARTESIAN_POINT('Ctrl Pts',(44.780287027359,-12.,82.1297407150269));
#65638=CARTESIAN_POINT('Ctrl Pts',(44.780287027359,-12.4,82.1297407150269));
#65639=CARTESIAN_POINT('',(45.1186230182648,-12.,83.5718955993652));
#65640=CARTESIAN_POINT('Ctrl Pts',(44.780287027359,-12.,82.1297407150269));
#65641=CARTESIAN_POINT('Ctrl Pts',(45.1186230182648,-12.,82.5315141677856));
#65642=CARTESIAN_POINT('Ctrl Pts',(45.1186230182648,-12.,83.5718955993652));
#65643=CARTESIAN_POINT('',(45.1186230182648,-12.4,83.5718955993652));
#65644=CARTESIAN_POINT('Ctrl Pts',(45.1186230182648,-12.4,83.5718955993652));
#65645=CARTESIAN_POINT('Ctrl Pts',(45.1186230182648,-12.4,82.5315141677856));
#65646=CARTESIAN_POINT('Ctrl Pts',(44.780287027359,-12.4,82.1297407150269));
#65647=CARTESIAN_POINT('',(45.1186230182648,-12.,83.5718955993652));
#65648=CARTESIAN_POINT('Ctrl Pts',(44.7654850482941,-12.,84.8512268066406));
#65649=CARTESIAN_POINT('Ctrl Pts',(44.7654850482941,-12.4,84.8512268066406));
#65650=CARTESIAN_POINT('Ctrl Pts',(45.1186230182648,-12.,84.4473390579224));
#65651=CARTESIAN_POINT('Ctrl Pts',(45.1186230182648,-12.4,84.4473390579224));
#65652=CARTESIAN_POINT('Ctrl Pts',(45.1186230182648,-12.,83.5718955993652));
#65653=CARTESIAN_POINT('Ctrl Pts',(45.1186230182648,-12.4,83.5718955993652));
#65654=CARTESIAN_POINT('',(44.7654850482941,-12.,84.8512268066406));
#65655=CARTESIAN_POINT('Ctrl Pts',(45.1186230182648,-12.,83.5718955993652));
#65656=CARTESIAN_POINT('Ctrl Pts',(45.1186230182648,-12.,84.4473390579224));
#65657=CARTESIAN_POINT('Ctrl Pts',(44.7654850482941,-12.,84.8512268066406));
#65658=CARTESIAN_POINT('',(44.7654850482941,-12.4,84.8512268066406));
#65659=CARTESIAN_POINT('Ctrl Pts',(44.7654850482941,-12.4,84.8512268066406));
#65660=CARTESIAN_POINT('Ctrl Pts',(45.1186230182648,-12.4,84.4473390579224));
#65661=CARTESIAN_POINT('Ctrl Pts',(45.1186230182648,-12.4,83.5718955993652));
#65662=CARTESIAN_POINT('',(44.7654850482941,-12.,84.8512268066406));
#65663=CARTESIAN_POINT('Ctrl Pts',(43.8075726032257,-12.,85.2551155090332));
#65664=CARTESIAN_POINT('Ctrl Pts',(43.8075726032257,-12.4,85.2551155090332));
#65665=CARTESIAN_POINT('Ctrl Pts',(44.4123470783234,-12.,85.2551155090332));
#65666=CARTESIAN_POINT('Ctrl Pts',(44.4123470783234,-12.4,85.2551155090332));
#65667=CARTESIAN_POINT('Ctrl Pts',(44.7654850482941,-12.,84.8512268066406));
#65668=CARTESIAN_POINT('Ctrl Pts',(44.7654850482941,-12.4,84.8512268066406));
#65669=CARTESIAN_POINT('',(43.8075726032257,-12.,85.2551155090332));
#65670=CARTESIAN_POINT('Ctrl Pts',(44.7654850482941,-12.,84.8512268066406));
#65671=CARTESIAN_POINT('Ctrl Pts',(44.4123470783234,-12.,85.2551155090332));
#65672=CARTESIAN_POINT('Ctrl Pts',(43.8075726032257,-12.,85.2551155090332));
#65673=CARTESIAN_POINT('',(43.8075726032257,-12.4,85.2551155090332));
#65674=CARTESIAN_POINT('Ctrl Pts',(43.8075726032257,-12.4,85.2551155090332));
#65675=CARTESIAN_POINT('Ctrl Pts',(44.4123470783234,-12.4,85.2551155090332));
#65676=CARTESIAN_POINT('Ctrl Pts',(44.7654850482941,-12.4,84.8512268066406));
#65677=CARTESIAN_POINT('',(43.8075726032257,-12.,85.2551155090332));
#65678=CARTESIAN_POINT('Ctrl Pts',(42.8771488666534,-12.,84.8448829650879));
#65679=CARTESIAN_POINT('Ctrl Pts',(42.8771488666534,-12.4,84.8448829650879));
#65680=CARTESIAN_POINT('Ctrl Pts',(43.2281725406647,-12.,85.2551155090332));
#65681=CARTESIAN_POINT('Ctrl Pts',(43.2281725406647,-12.4,85.2551155090332));
#65682=CARTESIAN_POINT('Ctrl Pts',(43.8075726032257,-12.,85.2551155090332));
#65683=CARTESIAN_POINT('Ctrl Pts',(43.8075726032257,-12.4,85.2551155090332));
#65684=CARTESIAN_POINT('Ctrl Pts',(43.8075726032257,-12.,85.2551155090332));
#65685=CARTESIAN_POINT('Ctrl Pts',(43.2281725406647,-12.,85.2551155090332));
#65686=CARTESIAN_POINT('Ctrl Pts',(42.8771488666534,-12.,84.8448829650879));
#65687=CARTESIAN_POINT('Ctrl Pts',(42.8771488666534,-12.4,84.8448829650879));
#65688=CARTESIAN_POINT('Ctrl Pts',(43.2281725406647,-12.4,85.2551155090332));
#65689=CARTESIAN_POINT('Ctrl Pts',(43.8075726032257,-12.4,85.2551155090332));
#65690=CARTESIAN_POINT('Ctrl Pts',(41.4561398029327,-12.,85.8598899841309));
#65691=CARTESIAN_POINT('Ctrl Pts',(41.4561398029327,-12.4,85.8598899841309));
#65692=CARTESIAN_POINT('Ctrl Pts',(40.6103012561798,-12.,85.0140514373779));
#65693=CARTESIAN_POINT('Ctrl Pts',(40.6103012561798,-12.4,85.0140514373779));
#65694=CARTESIAN_POINT('Ctrl Pts',(40.6103012561798,-12.,83.4957704544067));
#65695=CARTESIAN_POINT('Ctrl Pts',(40.6103012561798,-12.4,83.4957704544067));
#65696=CARTESIAN_POINT('',(40.6103012561798,-12.4,83.4957704544067));
#65697=CARTESIAN_POINT('',(40.6103012561798,-12.,83.4957704544067));
#65698=CARTESIAN_POINT('',(41.4561398029327,-12.4,85.8598899841309));
#65699=CARTESIAN_POINT('Ctrl Pts',(41.4561398029327,-12.4,85.8598899841309));
#65700=CARTESIAN_POINT('Ctrl Pts',(40.6103012561798,-12.4,85.0140514373779));
#65701=CARTESIAN_POINT('Ctrl Pts',(40.6103012561798,-12.4,83.4957704544067));
#65702=CARTESIAN_POINT('',(41.4561398029327,-12.,85.8598899841309));
#65703=CARTESIAN_POINT('Ctrl Pts',(43.8118011951447,-12.,86.7057290077209));
#65704=CARTESIAN_POINT('Ctrl Pts',(43.8118011951447,-12.4,86.7057290077209));
#65705=CARTESIAN_POINT('Ctrl Pts',(42.3019783496857,-12.,86.7057290077209));
#65706=CARTESIAN_POINT('Ctrl Pts',(42.3019783496857,-12.4,86.7057290077209));
#65707=CARTESIAN_POINT('Ctrl Pts',(41.4561398029327,-12.,85.8598899841309));
#65708=CARTESIAN_POINT('Ctrl Pts',(41.4561398029327,-12.4,85.8598899841309));
#65709=CARTESIAN_POINT('',(43.8118011951447,-12.4,86.7057290077209));
#65710=CARTESIAN_POINT('Ctrl Pts',(43.8118011951447,-12.4,86.7057290077209));
#65711=CARTESIAN_POINT('Ctrl Pts',(42.3019783496857,-12.4,86.7057290077209));
#65712=CARTESIAN_POINT('Ctrl Pts',(41.4561398029327,-12.4,85.8598899841309));
#65713=CARTESIAN_POINT('',(43.8118011951447,-12.,86.7057290077209));
#65714=CARTESIAN_POINT('Ctrl Pts',(46.1970684528351,-12.,85.874692440033));
#65715=CARTESIAN_POINT('Ctrl Pts',(46.1970684528351,-12.4,85.874692440033));
#65716=CARTESIAN_POINT('Ctrl Pts',(45.35968708992,-12.,86.7057290077209));
#65717=CARTESIAN_POINT('Ctrl Pts',(45.35968708992,-12.4,86.7057290077209));
#65718=CARTESIAN_POINT('Ctrl Pts',(43.8118011951447,-12.,86.7057290077209));
#65719=CARTESIAN_POINT('Ctrl Pts',(43.8118011951447,-12.4,86.7057290077209));
#65720=CARTESIAN_POINT('',(46.1970684528351,-12.4,85.874692440033));
#65721=CARTESIAN_POINT('Ctrl Pts',(46.1970684528351,-12.4,85.874692440033));
#65722=CARTESIAN_POINT('Ctrl Pts',(45.35968708992,-12.4,86.7057290077209));
#65723=CARTESIAN_POINT('Ctrl Pts',(43.8118011951447,-12.4,86.7057290077209));
#65724=CARTESIAN_POINT('',(46.1970684528351,-12.,85.874692440033));
#65725=CARTESIAN_POINT('Ctrl Pts',(47.0344479084015,-12.,83.5465202331543));
#65726=CARTESIAN_POINT('Ctrl Pts',(47.0344479084015,-12.4,83.5465202331543));
#65727=CARTESIAN_POINT('Ctrl Pts',(47.0344479084015,-12.,85.0436553955078));
#65728=CARTESIAN_POINT('Ctrl Pts',(47.0344479084015,-12.4,85.0436553955078));
#65729=CARTESIAN_POINT('Ctrl Pts',(46.1970684528351,-12.,85.874692440033));
#65730=CARTESIAN_POINT('Ctrl Pts',(46.1970684528351,-12.4,85.874692440033));
#65731=CARTESIAN_POINT('',(47.0344479084015,-12.4,83.5465202331543));
#65732=CARTESIAN_POINT('Ctrl Pts',(47.0344479084015,-12.4,83.5465202331543));
#65733=CARTESIAN_POINT('Ctrl Pts',(47.0344479084015,-12.4,85.0436553955078));
#65734=CARTESIAN_POINT('Ctrl Pts',(46.1970684528351,-12.4,85.874692440033));
#65735=CARTESIAN_POINT('',(47.0344479084015,-12.,83.5465202331543));
#65736=CARTESIAN_POINT('Ctrl Pts',(46.6686222553253,-12.,81.7639150619507));
#65737=CARTESIAN_POINT('Ctrl Pts',(46.6686222553253,-12.4,81.7639150619507));
#65738=CARTESIAN_POINT('Ctrl Pts',(47.0344479084015,-12.,82.4596176147461));
#65739=CARTESIAN_POINT('Ctrl Pts',(47.0344479084015,-12.4,82.4596176147461));
#65740=CARTESIAN_POINT('Ctrl Pts',(47.0344479084015,-12.,83.5465202331543));
#65741=CARTESIAN_POINT('Ctrl Pts',(47.0344479084015,-12.4,83.5465202331543));
#65742=CARTESIAN_POINT('',(46.6686222553253,-12.4,81.7639150619507));
#65743=CARTESIAN_POINT('Ctrl Pts',(46.6686222553253,-12.4,81.7639150619507));
#65744=CARTESIAN_POINT('Ctrl Pts',(47.0344479084015,-12.4,82.4596176147461));
#65745=CARTESIAN_POINT('Ctrl Pts',(47.0344479084015,-12.4,83.5465202331543));
#65746=CARTESIAN_POINT('',(46.6686222553253,-12.,81.7639150619507));
#65747=CARTESIAN_POINT('Ctrl Pts',(45.611323595047,-12.,80.6812410354614));
#65748=CARTESIAN_POINT('Ctrl Pts',(45.611323595047,-12.4,80.6812410354614));
#65749=CARTESIAN_POINT('Ctrl Pts',(46.3027966022491,-12.,81.0682125091553));
#65750=CARTESIAN_POINT('Ctrl Pts',(46.3027966022491,-12.4,81.0682125091553));
#65751=CARTESIAN_POINT('Ctrl Pts',(46.6686222553253,-12.,81.7639150619507));
#65752=CARTESIAN_POINT('Ctrl Pts',(46.6686222553253,-12.4,81.7639150619507));
#65753=CARTESIAN_POINT('',(45.611323595047,-12.4,80.6812410354614));
#65754=CARTESIAN_POINT('Ctrl Pts',(45.611323595047,-12.4,80.6812410354614));
#65755=CARTESIAN_POINT('Ctrl Pts',(46.3027966022491,-12.4,81.0682125091553));
#65756=CARTESIAN_POINT('Ctrl Pts',(46.6686222553253,-12.4,81.7639150619507));
#65757=CARTESIAN_POINT('',(45.611323595047,-12.,80.6812410354614));
#65758=CARTESIAN_POINT('Ctrl Pts',(43.8879272937775,-12.,80.2942695617676));
#65759=CARTESIAN_POINT('Ctrl Pts',(43.8879272937775,-12.4,80.2942695617676));
#65760=CARTESIAN_POINT('Ctrl Pts',(44.9198505878448,-12.,80.2942695617676));
#65761=CARTESIAN_POINT('Ctrl Pts',(44.9198505878448,-12.4,80.2942695617676));
#65762=CARTESIAN_POINT('Ctrl Pts',(45.611323595047,-12.,80.6812410354614));
#65763=CARTESIAN_POINT('Ctrl Pts',(45.611323595047,-12.4,80.6812410354614));
#65764=CARTESIAN_POINT('',(43.8879272937775,-12.4,80.2942695617676));
#65765=CARTESIAN_POINT('Ctrl Pts',(43.8879272937775,-12.4,80.2942695617676));
#65766=CARTESIAN_POINT('Ctrl Pts',(44.9198505878448,-12.4,80.2942695617676));
#65767=CARTESIAN_POINT('Ctrl Pts',(45.611323595047,-12.4,80.6812410354614));
#65768=CARTESIAN_POINT('',(43.8879272937775,-12.,80.2942695617676));
#65769=CARTESIAN_POINT('Ctrl Pts',(42.1518423557281,-12.,80.6283760070801));
#65770=CARTESIAN_POINT('Ctrl Pts',(42.1518423557281,-12.4,80.6283760070801));
#65771=CARTESIAN_POINT('Ctrl Pts',(42.8390867710114,-12.,80.2942695617676));
#65772=CARTESIAN_POINT('Ctrl Pts',(42.8390867710114,-12.4,80.2942695617676));
#65773=CARTESIAN_POINT('Ctrl Pts',(43.8879272937775,-12.,80.2942695617676));
#65774=CARTESIAN_POINT('Ctrl Pts',(43.8879272937775,-12.4,80.2942695617676));
#65775=CARTESIAN_POINT('',(42.1518423557281,-12.4,80.6283760070801));
#65776=CARTESIAN_POINT('Ctrl Pts',(42.1518423557281,-12.4,80.6283760070801));
#65777=CARTESIAN_POINT('Ctrl Pts',(42.8390867710114,-12.4,80.2942695617676));
#65778=CARTESIAN_POINT('Ctrl Pts',(43.8879272937775,-12.4,80.2942695617676));
#65779=CARTESIAN_POINT('',(42.1518423557281,-12.,80.6283760070801));
#65780=CARTESIAN_POINT('Ctrl Pts',(41.0374491214752,-12.,81.6856746673584));
#65781=CARTESIAN_POINT('Ctrl Pts',(41.0374491214752,-12.4,81.6856746673584));
#65782=CARTESIAN_POINT('Ctrl Pts',(41.4645979404449,-12.,80.9624824523926));
#65783=CARTESIAN_POINT('Ctrl Pts',(41.4645979404449,-12.4,80.9624824523926));
#65784=CARTESIAN_POINT('Ctrl Pts',(42.1518423557281,-12.,80.6283760070801));
#65785=CARTESIAN_POINT('Ctrl Pts',(42.1518423557281,-12.4,80.6283760070801));
#65786=CARTESIAN_POINT('',(41.0374491214752,-12.4,81.6856746673584));
#65787=CARTESIAN_POINT('Ctrl Pts',(41.0374491214752,-12.4,81.6856746673584));
#65788=CARTESIAN_POINT('Ctrl Pts',(41.4645979404449,-12.4,80.9624824523926));
#65789=CARTESIAN_POINT('Ctrl Pts',(42.1518423557281,-12.4,80.6283760070801));
#65790=CARTESIAN_POINT('',(41.0374491214752,-12.,81.6856746673584));
#65791=CARTESIAN_POINT('Ctrl Pts',(40.6103012561798,-12.,83.4957704544067));
#65792=CARTESIAN_POINT('Ctrl Pts',(40.6103012561798,-12.4,83.4957704544067));
#65793=CARTESIAN_POINT('Ctrl Pts',(40.6103012561798,-12.,82.4088668823242));
#65794=CARTESIAN_POINT('Ctrl Pts',(40.6103012561798,-12.4,82.4088668823242));
#65795=CARTESIAN_POINT('Ctrl Pts',(41.0374491214752,-12.,81.6856746673584));
#65796=CARTESIAN_POINT('Ctrl Pts',(41.0374491214752,-12.4,81.6856746673584));
#65797=CARTESIAN_POINT('Ctrl Pts',(40.6103012561798,-12.4,83.4957704544067));
#65798=CARTESIAN_POINT('Ctrl Pts',(40.6103012561798,-12.4,82.4088668823242));
#65799=CARTESIAN_POINT('Ctrl Pts',(41.0374491214752,-12.4,81.6856746673584));
#65800=CARTESIAN_POINT('Origin',(43.8223745822906,-12.4,83.4999992847443));
#65801=CARTESIAN_POINT('Origin',(49.5719635486603,-12.,82.1255111694336));
#65802=CARTESIAN_POINT('',(47.7322647571564,-12.4,82.1255111694336));
#65803=CARTESIAN_POINT('',(47.7322647571564,-12.,82.1255111694336));
#65804=CARTESIAN_POINT('',(49.5719635486603,-12.4,82.1255111694336));
#65805=CARTESIAN_POINT('',(47.7322647571564,-12.4,82.1255111694336));
#65806=CARTESIAN_POINT('',(49.5719635486603,-12.,82.1255111694336));
#65807=CARTESIAN_POINT('Origin',(49.5719635486603,-12.,80.3999996185303));
#65808=CARTESIAN_POINT('',(49.5719635486603,-12.4,80.3999996185303));
#65809=CARTESIAN_POINT('',(49.5719635486603,-12.4,82.1255111694336));
#65810=CARTESIAN_POINT('',(49.5719635486603,-12.,80.3999996185303));
#65811=CARTESIAN_POINT('Origin',(47.7322647571564,-12.,80.3999996185303));
#65812=CARTESIAN_POINT('',(47.7322647571564,-12.4,80.3999996185303));
#65813=CARTESIAN_POINT('',(49.5719635486603,-12.4,80.3999996185303));
#65814=CARTESIAN_POINT('',(47.7322647571564,-12.,80.3999996185303));
#65815=CARTESIAN_POINT('Origin',(47.7322647571564,-12.,82.1255111694336));
#65816=CARTESIAN_POINT('',(47.7322647571564,-12.4,80.3999996185303));
#65817=CARTESIAN_POINT('Origin',(48.6521141529083,-12.4,81.2627553939819));
#65818=CARTESIAN_POINT('Origin',(56.25,15.,10.5));
#65819=CARTESIAN_POINT('',(51.75,15.,10.5));
#65820=CARTESIAN_POINT('Origin',(54.,15.,10.5));
#65821=CARTESIAN_POINT('Origin',(54.,15.,10.765));
#65822=CARTESIAN_POINT('',(51.75,15.,10.765));
#65823=CARTESIAN_POINT('Origin',(56.25,-15.,10.5));
#65824=CARTESIAN_POINT('',(51.75,-15.,10.5));
#65825=CARTESIAN_POINT('Origin',(54.,-15.,10.5));
#65826=CARTESIAN_POINT('Origin',(54.,-15.,10.765));
#65827=CARTESIAN_POINT('',(51.75,-15.,10.765));
#65828=CARTESIAN_POINT('Origin',(-8.,15.,10.765));
#65829=CARTESIAN_POINT('',(-10.25,15.,10.765));
#65830=CARTESIAN_POINT('Origin',(-8.,-15.,10.765));
#65831=CARTESIAN_POINT('',(-10.25,-15.,10.765));
#65832=CARTESIAN_POINT('Origin',(-6.,11.,0.));
#65833=CARTESIAN_POINT('',(-6.,-11.,0.));
#65834=CARTESIAN_POINT('Origin',(48.,-11.,0.));
#65835=CARTESIAN_POINT('',(48.,-11.,0.));
#65836=CARTESIAN_POINT('Origin',(-6.,-11.,0.));
#65837=CARTESIAN_POINT('Origin',(0.,0.,11.));
#65838=CARTESIAN_POINT('Origin',(-11.9,9.5,0.1));
#65839=CARTESIAN_POINT('',(-12.,17.5,0.2));
#65840=CARTESIAN_POINT('',(-12.,9.5,0.2));
#65841=CARTESIAN_POINT('',(-11.8,17.5,0.));
#65842=CARTESIAN_POINT('Origin',(-12.,19.,0.));
#65843=CARTESIAN_POINT('',(-12.,17.5,0.));
#65844=CARTESIAN_POINT('Origin',(4.62,-2.26,64.1));
#65845=CARTESIAN_POINT('',(4.72,-4.72,64.));
#65846=CARTESIAN_POINT('Origin',(8.95,-4.62,64.1));
#65847=CARTESIAN_POINT('',(1.425,-4.52,64.2));
#65848=CARTESIAN_POINT('Origin',(-6.1,-4.52,62.));
#65849=CARTESIAN_POINT('',(4.52,-4.52,91.8));
#65850=CARTESIAN_POINT('',(-6.05,-4.52,91.8));
#65851=CARTESIAN_POINT('',(4.52,-4.52,62.));
#65852=CARTESIAN_POINT('Origin',(4.62,-2.26,91.9));
#65853=CARTESIAN_POINT('',(4.52,-2.26,91.8));
#65854=CARTESIAN_POINT('',(4.52,-4.52,91.8));
#65855=CARTESIAN_POINT('Origin',(-6.05,-4.62,91.9));
#65856=CARTESIAN_POINT('Origin',(4.52,-4.52,62.));
#65857=CARTESIAN_POINT('Origin',(9.31,13.9,78.));
#65858=CARTESIAN_POINT('',(2.855,14.,78.));
#65859=CARTESIAN_POINT('Origin',(9.31,14.,78.));
#65860=CARTESIAN_POINT('',(2.955,13.9,78.));
#65861=CARTESIAN_POINT('Origin',(9.31,14.,78.));
#65862=CARTESIAN_POINT('',(-0.390000000000001,14.,78.));
#65863=CARTESIAN_POINT('Origin',(9.31,14.,78.));
#65864=CARTESIAN_POINT('Origin',(9.31,-13.9,78.));
#65865=CARTESIAN_POINT('',(2.855,-14.,78.));
#65866=CARTESIAN_POINT('Origin',(9.31,-14.,78.));
#65867=CARTESIAN_POINT('',(2.955,-13.9,78.));
#65868=CARTESIAN_POINT('Origin',(9.31,-14.,78.));
#65869=CARTESIAN_POINT('',(-0.390000000000001,-14.,78.));
#65870=CARTESIAN_POINT('Origin',(9.31,-14.,78.));
#65871=CARTESIAN_POINT('Origin',(9.31,-12.15,78.));
#65872=CARTESIAN_POINT('',(-0.690000000000001,-12.3,78.));
#65873=CARTESIAN_POINT('',(-0.840000000000002,-12.15,78.));
#65874=CARTESIAN_POINT('Origin',(9.31,-12.3,78.));
#65875=CARTESIAN_POINT('Origin',(9.31,0.,78.));
#65876=CARTESIAN_POINT('',(-0.690000000000001,-13.7,78.));
#65877=CARTESIAN_POINT('',(-0.690000000000001,0.,78.));
#65878=CARTESIAN_POINT('Origin',(9.31,-13.7,78.));
#65879=CARTESIAN_POINT('Origin',(24.25,-12.,61.5));
#65880=CARTESIAN_POINT('Origin',(9.31,-13.85,78.));
#65881=CARTESIAN_POINT('',(-0.540000000000001,-13.85,78.));
#65882=CARTESIAN_POINT('Origin',(9.31,12.15,78.));
#65883=CARTESIAN_POINT('',(-0.690000000000001,12.3,78.));
#65884=CARTESIAN_POINT('',(-0.840000000000002,12.15,78.));
#65885=CARTESIAN_POINT('Origin',(9.31,12.3,78.));
#65886=CARTESIAN_POINT('Origin',(9.31,0.,78.));
#65887=CARTESIAN_POINT('',(-0.690000000000001,13.7,78.));
#65888=CARTESIAN_POINT('Origin',(9.31,13.7,78.));
#65889=CARTESIAN_POINT('',(-0.690000000000001,0.,78.));
#65890=CARTESIAN_POINT('Origin',(9.31,13.85,78.));
#65891=CARTESIAN_POINT('',(-0.540000000000001,13.85,78.));
#65892=CARTESIAN_POINT('Origin',(24.0625,-12.106066017178,11.343933982822));
#65893=CARTESIAN_POINT('',(27.1391971013664,-12.212132034356,11.087867965644));
#65894=CARTESIAN_POINT('Origin',(24.,-10.0189862838483,16.3825901807804));
#65895=CARTESIAN_POINT('',(24.0625,-12.212132034356,11.087867965644));
#65896=CARTESIAN_POINT('Origin',(44.,-11.85,100.));
#65897=CARTESIAN_POINT('',(32.,-11.7,100.));
#65898=CARTESIAN_POINT('Origin',(32.15,-11.85,79.25));
#65899=CARTESIAN_POINT('',(32.,-11.7,97.));
#65900=CARTESIAN_POINT('Origin',(27.,-11.85,97.));
#65901=CARTESIAN_POINT('',(27.,-11.7,92.));
#65902=CARTESIAN_POINT('Origin',(27.,-11.7,97.));
#65903=CARTESIAN_POINT('Origin',(9.125,-11.85,91.85));
#65904=CARTESIAN_POINT('Origin',(-9.85,-11.85,64.75));
#65905=CARTESIAN_POINT('',(-10.,-11.7,68.));
#65906=CARTESIAN_POINT('Origin',(-5.99999999999999,-11.85,68.));
#65907=CARTESIAN_POINT('',(-6.,-11.7,64.));
#65908=CARTESIAN_POINT('Origin',(24.125,-11.85,64.15));
#65909=CARTESIAN_POINT('Origin',(32.15,-11.85,40.25));
#65910=CARTESIAN_POINT('',(32.,-11.7,19.));
#65911=CARTESIAN_POINT('Origin',(24.,-11.85,19.));
#65912=CARTESIAN_POINT('',(27.0983866769659,-12.,11.3));
#65913=CARTESIAN_POINT('Ctrl Pts',(27.0983866769659,-12.,11.3));
#65914=CARTESIAN_POINT('Ctrl Pts',(27.0690767311041,-11.8486440903987,11.4513559096013));
#65915=CARTESIAN_POINT('Ctrl Pts',(27.0397667852433,-11.7001517572237,11.5998482427763));
#65916=CARTESIAN_POINT('Ctrl Pts',(27.1391971013664,-12.212132034356,11.087867965644));
#65917=CARTESIAN_POINT('Ctrl Pts',(27.1187918891661,-12.1053720627028,11.1946279372972));
#65918=CARTESIAN_POINT('Ctrl Pts',(27.0983866769659,-12.,11.3));
#65919=CARTESIAN_POINT('Origin',(27.,0.,97.));
#65920=CARTESIAN_POINT('Origin',(27.,11.7,97.));
#65921=CARTESIAN_POINT('Origin',(58.5,0.,13.5));
#65922=CARTESIAN_POINT('Origin',(58.5,-9.79999999999997,13.5));
#65923=CARTESIAN_POINT('Origin',(32.15,11.85,40.25));
#65924=CARTESIAN_POINT('',(32.,11.7,56.));
#65925=CARTESIAN_POINT('Origin',(24.,11.85,56.));
#65926=CARTESIAN_POINT('',(24.,11.7,64.));
#65927=CARTESIAN_POINT('Origin',(24.125,11.85,64.15));
#65928=CARTESIAN_POINT('Origin',(-9.85,11.85,64.75));
#65929=CARTESIAN_POINT('Origin',(9.125,11.85,91.85));
#65930=CARTESIAN_POINT('',(27.,11.7,92.));
#65931=CARTESIAN_POINT('Origin',(27.,11.85,97.));
#65932=CARTESIAN_POINT('',(32.,11.7,97.));
#65933=CARTESIAN_POINT('Origin',(32.15,11.85,79.25));
#65934=CARTESIAN_POINT('Origin',(58.9,-9.5,0.1));
#65935=CARTESIAN_POINT('',(59.,17.5,0.2));
#65936=CARTESIAN_POINT('',(58.8,17.5,0.));
#65937=CARTESIAN_POINT('',(59.,-17.5,0.2));
#65938=CARTESIAN_POINT('',(59.,-9.5,0.2));
#65939=CARTESIAN_POINT('',(59.,-17.5,0.2));
#65940=CARTESIAN_POINT('Origin',(57.5,17.5,0.1));
#65941=CARTESIAN_POINT('',(57.5,19.,0.2));
#65942=CARTESIAN_POINT('',(57.5,18.8,0.));
#65943=CARTESIAN_POINT('Origin',(57.5,17.5,0.2));
#65944=CARTESIAN_POINT('Origin',(41.25,18.9,0.1));
#65945=CARTESIAN_POINT('',(-10.5,19.,0.2));
#65946=CARTESIAN_POINT('',(-10.5,18.8,0.));
#65947=CARTESIAN_POINT('',(41.25,19.,0.2));
#65948=CARTESIAN_POINT('Origin',(-10.5,17.5,0.1));
#65949=CARTESIAN_POINT('Origin',(-10.5,17.5,0.2));
#65950=CARTESIAN_POINT('Origin',(-10.5,-17.5,0.1));
#65951=CARTESIAN_POINT('',(-10.5,-19.,0.2));
#65952=CARTESIAN_POINT('',(-10.5,-18.8,0.));
#65953=CARTESIAN_POINT('Origin',(-10.5,-17.5,0.2));
#65954=CARTESIAN_POINT('Origin',(5.75,-18.9,0.1));
#65955=CARTESIAN_POINT('',(57.5,-19.,0.2));
#65956=CARTESIAN_POINT('',(57.5,-18.8,0.));
#65957=CARTESIAN_POINT('',(5.75,-19.,0.2));
#65958=CARTESIAN_POINT('Origin',(57.5,-17.5,0.1));
#65959=CARTESIAN_POINT('Origin',(57.5,-17.5,0.2));
#65960=CARTESIAN_POINT('Origin',(-10.5,-17.5,0.));
#65961=CARTESIAN_POINT('',(-10.5,-19.,10.7));
#65962=CARTESIAN_POINT('',(-10.5,-19.,0.));
#65963=CARTESIAN_POINT('Origin',(-10.5,-17.5,10.7));
#65964=CARTESIAN_POINT('Origin',(-12.,-19.,0.));
#65965=CARTESIAN_POINT('',(57.5,-19.,10.7));
#65966=CARTESIAN_POINT('',(57.5,-19.,0.));
#65967=CARTESIAN_POINT('',(5.75,-19.,10.7));
#65968=CARTESIAN_POINT('Origin',(57.5,-17.5,0.));
#65969=CARTESIAN_POINT('',(59.,-17.5,10.7));
#65970=CARTESIAN_POINT('',(59.,-17.5,0.));
#65971=CARTESIAN_POINT('Origin',(57.5,-17.5,10.7));
#65972=CARTESIAN_POINT('Origin',(59.,-19.,0.));
#65973=CARTESIAN_POINT('',(59.,17.5,10.7));
#65974=CARTESIAN_POINT('',(59.,17.5,0.));
#65975=CARTESIAN_POINT('',(59.,-9.5,10.7));
#65976=CARTESIAN_POINT('Origin',(23.875,-12.15,11.15));
#65977=CARTESIAN_POINT('Origin',(-10.5,-17.5,10.85));
#65978=CARTESIAN_POINT('',(-10.5,-19.,10.7));
#65979=CARTESIAN_POINT('Origin',(-10.5,17.5,10.85));
#65980=CARTESIAN_POINT('',(-10.5,19.,10.7));
#65981=CARTESIAN_POINT('',(-10.5,18.7,11.));
#65982=CARTESIAN_POINT('Origin',(-10.5,17.5,10.7));
#65983=CARTESIAN_POINT('Origin',(41.25,18.85,10.85));
#65984=CARTESIAN_POINT('',(57.5,19.,10.7));
#65985=CARTESIAN_POINT('',(57.5,18.7,11.));
#65986=CARTESIAN_POINT('',(41.25,19.,10.7));
#65987=CARTESIAN_POINT('Origin',(57.5,17.5,10.85));
#65988=CARTESIAN_POINT('',(58.7,17.5,11.));
#65989=CARTESIAN_POINT('Origin',(57.5,17.5,10.7));
#65990=CARTESIAN_POINT('Origin',(58.85,-9.5,10.85));
#65991=CARTESIAN_POINT('',(58.7,-17.5,11.));
#65992=CARTESIAN_POINT('Origin',(57.5,-17.5,10.85));
#65993=CARTESIAN_POINT('',(57.5,-18.7,11.));
#65994=CARTESIAN_POINT('Origin',(5.75,-18.85,10.85));
#65995=CARTESIAN_POINT('Origin',(57.5,17.5,0.));
#65996=CARTESIAN_POINT('',(57.5,19.,0.));
#65997=CARTESIAN_POINT('Origin',(-10.5,17.5,0.));
#65998=CARTESIAN_POINT('',(-10.5,19.,0.));
#65999=CARTESIAN_POINT('Origin',(59.,19.,0.));
#70738=UNCERTAINTY_MEASURE_WITH_UNIT(LENGTH_MEASURE(0.001),#70758,
'DISTANCE_ACCURACY_VALUE',
'Maximum model space distance between geometric entities at asserted c
onnectivities');
#70740=UNCERTAINTY_MEASURE_WITH_UNIT(LENGTH_MEASURE(0.001),#70758,
'DISTANCE_ACCURACY_VALUE',
'Maximum model space distance between geometric entities at asserted c
onnectivities');
#70755=(
GEOMETRIC_REPRESENTATION_CONTEXT(3)
GLOBAL_UNCERTAINTY_ASSIGNED_CONTEXT((#70738))
GLOBAL_UNIT_ASSIGNED_CONTEXT((#70758,#70760,#70761))
REPRESENTATION_CONTEXT('','3D')
);
#70757=(
GEOMETRIC_REPRESENTATION_CONTEXT(3)
GLOBAL_UNCERTAINTY_ASSIGNED_CONTEXT((#70740))
GLOBAL_UNIT_ASSIGNED_CONTEXT((#70758,#70760,#70761))
REPRESENTATION_CONTEXT('','3D')
);
#70758=(
LENGTH_UNIT()
NAMED_UNIT(*)
SI_UNIT(.CENTI.,.METRE.)
);
#70760=(
NAMED_UNIT(*)
PLANE_ANGLE_UNIT()
SI_UNIT($,.RADIAN.)
);
#70761=(
NAMED_UNIT(*)
SI_UNIT($,.STERADIAN.)
SOLID_ANGLE_UNIT()
);
#70776=SHAPE_DEFINITION_REPRESENTATION(#70792,#70831);
#70792=PRODUCT_DEFINITION_SHAPE('',$,#70848);
#70831=SHAPE_REPRESENTATION('',(#28396),#70755);
#70833=PRODUCT_DEFINITION_CONTEXT('part definition',#70883,'design');
#70848=PRODUCT_DEFINITION('2026-10-19-03-02-56-883',
'01_Cast_Iron_C-Frame_NO.1_840x380_Base',#70864,#70833);
#70864=PRODUCT_DEFINITION_FORMATION('',$,#70899);
#70883=APPLICATION_CONTEXT(
'Core Data for Automotive Mechanical Design Process');
#70884=PRODUCT_CONTEXT('part definition',#70883,'mechanical');
#70899=PRODUCT('2026-10-19-03-02-56-883',
'01_Cast_Iron_C-Frame_NO.1_840x380_Base',$,(#70884));
#71020=COLOUR_RGB('Dark Blue',0.08,0.2,0.34);
#71021=FILL_AREA_STYLE_COLOUR('',#71020);
#71022=FILL_AREA_STYLE('',(#71021));
#71023=SURFACE_STYLE_FILL_AREA(#71022);
#71024=SURFACE_SIDE_STYLE('',(#71023));
#71025=SURFACE_STYLE_USAGE(.BOTH.,#71024);
#71026=PRESENTATION_STYLE_ASSIGNMENT((#71025));
ENDSEC;
END-ISO-10303-21;
